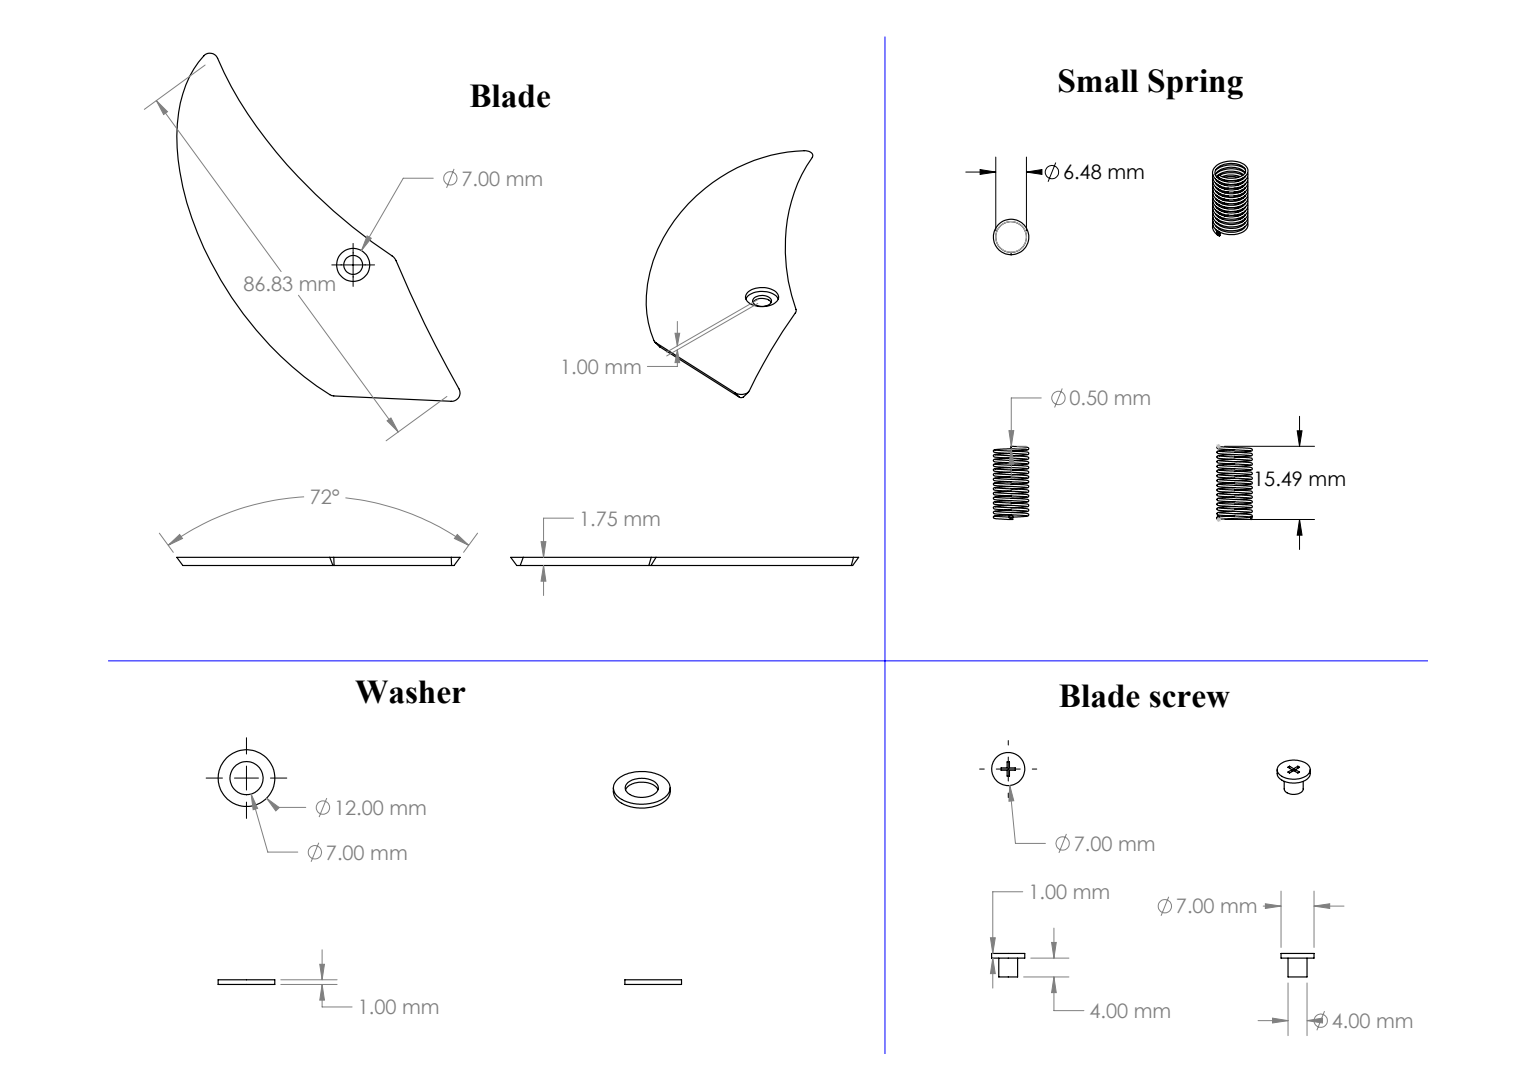
ISO-10303-21;
HEADER;
FILE_DESCRIPTION (('STEP AP203'),
    '1' );
FILE_NAME ('SmallSpring.step',
    '2026-10-08T11:28:20',
    ( '' ),
    ( '' ),
    'SwSTEP 2.0',
    'SolidWorks 2024',
    '' );
FILE_SCHEMA (( 'AUTOMOTIVE_DESIGN' ));
ENDSEC;

DATA;
#1=B_SPLINE_CURVE_WITH_KNOTS ( 'NONE', 3,
 ( #11082, #3985, #4982, #9929, #8605, #7599 ),
 .UNSPECIFIED., .F., .F.,
 ( 4, 2, 4 ),
 ( 0.000000000000000000, 0.0003771276215161150453, 0.0007542552430322300907 ),
 .UNSPECIFIED. ) ;
#3=CARTESIAN_POINT ( 'NONE',  ( 3.749999999999999112, 3.187500000000000444, -5.053300858899108405 ) ) ;
#9=CARTESIAN_POINT ( 'NONE',  ( 3.249999999999999556, 12.75000000000000178, -3.500000000000000000 ) ) ;
#19=CARTESIAN_POINT ( 'NONE',  ( -3.750000000000000000, 6.250000000000000000, -3.499999999999999112 ) ) ;
#20=CARTESIAN_POINT ( 'NONE',  ( 3.749999999999999556, 3.250000000000000000, -3.500000000000000444 ) ) ;
#24=CARTESIAN_POINT ( 'NONE',  ( -2.298097038856279362, 0.8750000000000000000, -5.798097038856278473 ) ) ;
#31=CARTESIAN_POINT ( 'NONE',  ( 0.000000000000000000, 3.000000000000000000, -0.2500000000000002220 ) ) ;
#37=CARTESIAN_POINT ( 'NONE',  ( -3.249999999999999556, 14.18750000000000000, -2.153805922287440833 ) ) ;
#42=CARTESIAN_POINT ( 'NONE',  ( 1.553300858899105963, 4.062500000000001776, -7.250000000000000888 ) ) ;
#43=CARTESIAN_POINT ( 'NONE',  ( -1.346194077712559167, 5.937500000000002665, -6.749999999999999112 ) ) ;
#47=CARTESIAN_POINT ( 'NONE',  ( 1.346194077712558057, 4.562500000000000888, -6.750000000000000000 ) ) ;
#59=CARTESIAN_POINT ( 'NONE',  ( 2.651650429449553314, 14.37500000000000000, -0.8483495705504476847 ) ) ;
#63=CARTESIAN_POINT ( 'NONE',  ( -3.249999999999999556, 3.750000000000000444, -3.500000000000000000 ) ) ;
#70=CARTESIAN_POINT ( 'NONE',  ( -3.249999999999999556, 1.250000000000000000, -3.499999999999999556 ) ) ;
#73=CARTESIAN_POINT ( 'NONE',  ( 2.298097038856278029, 7.125000000000000888, -5.798097038856279362 ) ) ;
#79=CARTESIAN_POINT ( 'NONE',  ( 2.298097038856279362, 1.875000000000000000, -1.201902961143720860 ) ) ;
#80=CARTESIAN_POINT ( 'NONE',  ( -1.553300858899107073, 1.937500000000000222, -7.249999999999999112 ) ) ;
#82=CARTESIAN_POINT ( 'NONE',  ( -3.750000000000000000, 7.312500000000000000, -5.053300858899105741 ) ) ;
#84=CARTESIAN_POINT ( 'NONE',  ( 3.749999999999999556, 4.250000000000000000, -3.500000000000000444 ) ) ;
#87=DIRECTION ( 'NONE',  ( 0.000000000000000000, 0.000000000000000000, -1.000000000000000000 ) ) ;
#90=CARTESIAN_POINT ( 'NONE',  ( 1.346194077712560944, 10.93750000000000000, -0.2500000000000010547 ) ) ;
#97=CARTESIAN_POINT ( 'NONE',  ( 3.749999999999998668, 4.687500000000000888, -5.053300858899107517 ) ) ;
#99=CARTESIAN_POINT ( 'NONE',  ( -3.750000000000000000, 5.812500000000000888, -5.053300858899105741 ) ) ;
#103=CARTESIAN_POINT ( 'NONE',  ( 3.249999999999998224, 3.187500000000000444, -4.846194077712561388 ) ) ;
#106=CARTESIAN_POINT ( 'NONE',  ( -2.298097038856278918, 2.375000000000000000, -5.798097038856277585 ) ) ;
#113=CARTESIAN_POINT ( 'NONE',  ( 1.346194077712560944, 14.93750000000000178, -0.2500000000000011102 ) ) ;
#115=EDGE_LOOP ( 'NONE', ( #2577, #6448, #3644, #14462 ) ) ;
#117=CARTESIAN_POINT ( 'NONE',  ( -4.592425496802573972E-16, 5.000000000000000000, -7.250000000000000000 ) ) ;
#118=CARTESIAN_POINT ( 'NONE',  ( -1.346194077712558945, 10.56249999999999822, -0.2500000000000002220 ) ) ;
#122=CARTESIAN_POINT ( 'NONE',  ( 1.346194077712558057, 3.562500000000000444, -6.750000000000000000 ) ) ;
#129=CARTESIAN_POINT ( 'NONE',  ( -3.249999999999999556, 9.187500000000000000, -2.153805922287440833 ) ) ;
#131=CARTESIAN_POINT ( 'NONE',  ( -4.592425496802573972E-16, 14.00000000000000000, -7.250000000000000000 ) ) ;
#136=CARTESIAN_POINT ( 'NONE',  ( 1.346194077712561166, 4.437500000000001776, -0.2500000000000011102 ) ) ;
#143=EDGE_LOOP ( 'NONE', ( #10004, #6723, #11790, #8217 ) ) ;
#145=CARTESIAN_POINT ( 'NONE',  ( 2.298097038856279362, 1.875000000000000000, -1.201902961143720860 ) ) ;
#147=CARTESIAN_POINT ( 'NONE',  ( 3.249999999999999556, 14.75000000000000178, -3.500000000000000000 ) ) ;
#148=CARTESIAN_POINT ( 'NONE',  ( -1.346194077712559167, 5.937500000000002665, -6.749999999999999112 ) ) ;
#154=CARTESIAN_POINT ( 'NONE',  ( -2.298097038856278918, 0.3750000000000000000, -5.798097038856277585 ) ) ;
#155=CARTESIAN_POINT ( 'NONE',  ( 2.651650429449552870, 1.124999999999999778, -6.151650429449553314 ) ) ;
#156=CARTESIAN_POINT ( 'NONE',  ( -2.651650429449552870, 4.125000000000000000, -0.8483495705504462414 ) ) ;
#158=CARTESIAN_POINT ( 'NONE',  ( 2.651650429449552870, 8.125000000000000000, -6.151650429449555091 ) ) ;
#161=EDGE_CURVE ( 'NONE', #6131, #12717, #6840, .T. ) ;
#166=CARTESIAN_POINT ( 'NONE',  ( 0.000000000000000000, 14.00000000000000000, -0.2500000000000002220 ) ) ;
#170=CARTESIAN_POINT ( 'NONE',  ( -3.749999999999999556, 8.750000000000000000, -3.499999999999999112 ) ) ;
#174=CARTESIAN_POINT ( 'NONE',  ( 1.553300858899108849, 9.937499999999998224, 0.2499999999999993616 ) ) ;
#175=CARTESIAN_POINT ( 'NONE',  ( -3.749999999999999556, 5.750000000000000000, -3.499999999999999112 ) ) ;
#178=CARTESIAN_POINT ( 'NONE',  ( -2.298097038856278029, 2.625000000000000000, -1.201902961143720638 ) ) ;
#181=CARTESIAN_POINT ( 'NONE',  ( 2.298097038856279362, 6.875000000000000000, -1.201902961143720860 ) ) ;
#189=CARTESIAN_POINT ( 'NONE',  ( -3.980102097228897245E-16, 14.50000000000000000, -6.749999999999999112 ) ) ;
#193=CARTESIAN_POINT ( 'NONE',  ( 2.651650429449552870, 7.125000000000000888, -6.151650429449555091 ) ) ;
#194=CARTESIAN_POINT ( 'NONE',  ( -2.298097038856279362, 8.874999999999996447, -5.798097038856278473 ) ) ;
#197=CARTESIAN_POINT ( 'NONE',  ( -3.249999999999999556, 5.187500000000001776, -2.153805922287440833 ) ) ;
#204=CARTESIAN_POINT ( 'NONE',  ( -3.249999999999999556, 0.3125000000000000555, -4.846194077712557835 ) ) ;
#206=CARTESIAN_POINT ( 'NONE',  ( -3.750000000000000000, 12.81250000000000178, -5.053300858899105741 ) ) ;
#209=CARTESIAN_POINT ( 'NONE',  ( 1.346194077712561166, 3.437500000000000444, -0.2500000000000011102 ) ) ;
#216=CARTESIAN_POINT ( 'NONE',  ( -2.298097038856278918, 8.375000000000000000, -5.798097038856277585 ) ) ;
#218=CARTESIAN_POINT ( 'NONE',  ( 2.298097038856278473, 14.62500000000000000, -5.798097038856279362 ) ) ;
#220=CARTESIAN_POINT ( 'NONE',  ( 0.000000000000000000, 7.500000000000000888, -0.2500000000000002220 ) ) ;
#225=CARTESIAN_POINT ( 'NONE',  ( 2.298097038856278473, 1.625000000000000222, -5.798097038856279362 ) ) ;
#226=CARTESIAN_POINT ( 'NONE',  ( -2.651650429449552870, 2.625000000000000000, -0.8483495705504467965 ) ) ;
#227=CARTESIAN_POINT ( 'NONE',  ( 1.553300858899108849, 4.937500000000000888, 0.2499999999999993616 ) ) ;
#229=CARTESIAN_POINT ( 'NONE',  ( 1.553300858899105963, 6.062500000000000888, -7.250000000000000888 ) ) ;
#239=CARTESIAN_POINT ( 'NONE',  ( 1.346194077712560944, 8.937500000000001776, -0.2500000000000010547 ) ) ;
#242=CARTESIAN_POINT ( 'NONE',  ( -3.750000000000000000, 10.81250000000000000, -5.053300858899105741 ) ) ;
#246=CARTESIAN_POINT ( 'NONE',  ( 2.651650429449553759, 9.875000000000000000, -0.8483495705504471296 ) ) ;
#247=CARTESIAN_POINT ( 'NONE',  ( 3.749999999999998668, 4.187500000000000888, -5.053300858899108405 ) ) ;
#251=CARTESIAN_POINT ( 'NONE',  ( 2.298097038856278029, 5.125000000000000000, -5.798097038856279362 ) ) ;
#253=CARTESIAN_POINT ( 'NONE',  ( 2.651650429449553759, 10.87500000000000178, -0.8483495705504471296 ) ) ;
#258=CARTESIAN_POINT ( 'NONE',  ( 3.249999999999998668, 8.687500000000000000, -4.846194077712560500 ) ) ;
#260=CARTESIAN_POINT ( 'NONE',  ( -0.3766621274091715987, 0.2398196381212478467, -0.1347136637304948426 ) ) ;
#270=CARTESIAN_POINT ( 'NONE',  ( -3.750000000000000000, 10.68750000000000178, -1.946699141100893149 ) ) ;
#271=CARTESIAN_POINT ( 'NONE',  ( 1.346194077712558279, 6.062500000000000000, -6.750000000000000888 ) ) ;
#272=CARTESIAN_POINT ( 'NONE',  ( -3.249999999999999556, 10.75000000000000000, -3.500000000000000000 ) ) ;
#274=VECTOR ( 'NONE', #10771, 1000.000000000000000 ) ;
#277=CARTESIAN_POINT ( 'NONE',  ( -2.298097038856278473, 5.125000000000000000, -1.201902961143720416 ) ) ;
#287=CARTESIAN_POINT ( 'NONE',  ( 2.298097038856279362, 0.8750000000000000000, -1.201902961143720860 ) ) ;
#288=CARTESIAN_POINT ( 'NONE',  ( -1.553300858899107295, 11.43750000000000000, -7.250000000000000000 ) ) ;
#291=CARTESIAN_POINT ( 'NONE',  ( -2.651650429449552870, 11.62500000000000000, -0.8483495705504467965 ) ) ;
#294=CARTESIAN_POINT ( 'NONE',  ( -2.298097038856279362, 1.874999999999999778, -5.798097038856278473 ) ) ;
#303=CARTESIAN_POINT ( 'NONE',  ( 3.249999999999998668, 6.687500000000000888, -4.846194077712560500 ) ) ;
#305=CARTESIAN_POINT ( 'NONE',  ( 3.249999999999999556, 1.249999999999999778, -3.500000000000000000 ) ) ;
#306=CARTESIAN_POINT ( 'NONE',  ( 0.000000000000000000, 9.500000000000000000, -0.2500000000000002220 ) ) ;
#310=CARTESIAN_POINT ( 'NONE',  ( -1.346194077712559389, 4.062500000000000000, -0.2500000000000002220 ) ) ;
#311=CARTESIAN_POINT ( 'NONE',  ( 0.000000000000000000, 15.50000000000000178, -0.2500000000000002220 ) ) ;
#312=CARTESIAN_POINT ( 'NONE',  ( -1.553300858899106407, 7.062500000000000000, 0.2500000000000002220 ) ) ;
#314=CARTESIAN_POINT ( 'NONE',  ( -3.750000000000000000, 6.812500000000001776, -5.053300858899105741 ) ) ;
#318=VECTOR ( 'NONE', #638, 1000.000000000000000 ) ;
#326=CARTESIAN_POINT ( 'NONE',  ( 2.651650429449552870, 9.125000000000000000, -6.151650429449555091 ) ) ;
#330=CARTESIAN_POINT ( 'NONE',  ( 3.750000000000000000, 9.750000000000000000, -3.500000000000000444 ) ) ;
#331=CARTESIAN_POINT ( 'NONE',  ( -1.553300858899106629, 7.562500000000000888, 0.2499999999999998335 ) ) ;
#335=CARTESIAN_POINT ( 'NONE',  ( 1.346194077712561166, 4.437499999999999112, -0.2500000000000011102 ) ) ;
#336=CARTESIAN_POINT ( 'NONE',  ( 2.651650429449553759, 8.875000000000001776, -0.8483495705504471296 ) ) ;
#340=CARTESIAN_POINT ( 'NONE',  ( -1.346194077712559389, 7.437500000000000888, -6.749999999999999112 ) ) ;
#353=CARTESIAN_POINT ( 'NONE',  ( -2.651650429449552870, 12.62500000000000000, -0.8483495705504467965 ) ) ;
#354=CARTESIAN_POINT ( 'NONE',  ( 1.346194077712561166, 12.43750000000000000, -0.2500000000000011102 ) ) ;
#355=CARTESIAN_POINT ( 'NONE',  ( -3.249999999999999112, 11.81250000000000178, -4.846194077712558723 ) ) ;
#358=CARTESIAN_POINT ( 'NONE',  ( -1.346194077712559389, 7.062500000000000000, -0.2500000000000002220 ) ) ;
#367=EDGE_CURVE ( 'NONE', #14660, #7693, #12911, .T. ) ;
#370=CARTESIAN_POINT ( 'NONE',  ( -3.249999999999999556, 9.250000000000000000, -3.499999999999999556 ) ) ;
#371=CARTESIAN_POINT ( 'NONE',  ( -3.249999999999999556, 0.1875000000000000278, -2.153805922287440833 ) ) ;
#373=CARTESIAN_POINT ( 'NONE',  ( 3.749999999999999112, 14.81250000000000000, -1.946699141100892039 ) ) ;
#376=CARTESIAN_POINT ( 'NONE',  ( 0.000000000000000000, 1.000000000000000000, 0.2500000000000002220 ) ) ;
#385=CARTESIAN_POINT ( 'NONE',  ( 1.346194077712558279, 5.562500000000000000, -6.750000000000000000 ) ) ;
#387=CARTESIAN_POINT ( 'NONE',  ( -2.298097038856278473, 13.12500000000000000, -1.201902961143720416 ) ) ;
#388=CARTESIAN_POINT ( 'NONE',  ( 3.249999999999998224, 12.18750000000000178, -4.846194077712561388 ) ) ;
#392=CARTESIAN_POINT ( 'NONE',  ( 0.000000000000000000, 6.000000000000000000, -0.2500000000000002220 ) ) ;
#393=CARTESIAN_POINT ( 'NONE',  ( -3.749999999999999556, 0.7499999999999998890, -3.499999999999999112 ) ) ;
#394=CARTESIAN_POINT ( 'NONE',  ( 1.553300858899105963, 5.562500000000000000, -7.250000000000000000 ) ) ;
#396=CARTESIAN_POINT ( 'NONE',  ( 3.749999999999999556, 8.250000000000000000, -3.500000000000000444 ) ) ;
#401=CARTESIAN_POINT ( 'NONE',  ( 2.298097038856279362, 14.87500000000000178, -1.201902961143720860 ) ) ;
#404=CARTESIAN_POINT ( 'NONE',  ( 3.249999999999998224, 0.1875000000000000833, -4.846194077712561388 ) ) ;
#408=CARTESIAN_POINT ( 'NONE',  ( 2.651650429449553759, 7.875000000000000000, -0.8483495705504471296 ) ) ;
#409=CARTESIAN_POINT ( 'NONE',  ( -4.592425496802573972E-16, 8.000000000000000000, -7.250000000000000000 ) ) ;
#413=CARTESIAN_POINT ( 'NONE',  ( 2.298097038856278029, 6.125000000000000000, -5.798097038856279362 ) ) ;
#414=CARTESIAN_POINT ( 'NONE',  ( 2.651650429449552870, 11.62500000000000000, -6.151650429449554203 ) ) ;
#416=LINE ( 'NONE', #571, #1497 ) ;
#418=CARTESIAN_POINT ( 'NONE',  ( -3.249999999999999556, 7.250000000000000000, -3.499999999999999556 ) ) ;
#430=CARTESIAN_POINT ( 'NONE',  ( 1.553300858899105963, 11.06250000000000178, -7.249999999999999112 ) ) ;
#431=CARTESIAN_POINT ( 'NONE',  ( -3.249999999999999112, 11.68749999999999822, -2.153805922287440833 ) ) ;
#432=CARTESIAN_POINT ( 'NONE',  ( 2.298097038856279362, 12.37500000000000178, -1.201902961143720860 ) ) ;
#437=CARTESIAN_POINT ( 'NONE',  ( 1.346194077712560944, 6.937500000000000000, -0.2500000000000010547 ) ) ;
#438=EDGE_CURVE ( 'NONE', #15209, #13242, #13713, .T. ) ;
#443=CARTESIAN_POINT ( 'NONE',  ( -0.3766621274091715432, -0.2054769798019681903, -0.1347136637304948981 ) ) ;
#445=CARTESIAN_POINT ( 'NONE',  ( -3.249999999999999556, 1.187500000000000444, -2.153805922287440833 ) ) ;
#446=CARTESIAN_POINT ( 'NONE',  ( 3.749999999999999112, 12.81250000000000000, -1.946699141100892039 ) ) ;
#450=CARTESIAN_POINT ( 'NONE',  ( -3.749999999999999556, 0.1875000000000001110, -1.946699141100892927 ) ) ;
#459=CARTESIAN_POINT ( 'NONE',  ( -3.249999999999999556, 8.312500000000000000, -4.846194077712557835 ) ) ;
#461=CARTESIAN_POINT ( 'NONE',  ( 3.249999999999998668, 12.68750000000000178, -4.846194077712560500 ) ) ;
#462=CARTESIAN_POINT ( 'NONE',  ( 3.249999999999998224, 9.187500000000001776, -4.846194077712561388 ) ) ;
#466=CARTESIAN_POINT ( 'NONE',  ( -2.298097038856278918, 5.375000000000000000, -5.798097038856277585 ) ) ;
#467=CARTESIAN_POINT ( 'NONE',  ( 3.749999999999999556, 7.250000000000000000, -3.500000000000000444 ) ) ;
#469=CARTESIAN_POINT ( 'NONE',  ( 2.651650429449552870, 7.625000000000000000, -6.151650429449554203 ) ) ;
#471=CARTESIAN_POINT ( 'NONE',  ( 2.651650429449554203, 9.374999999999998224, -0.8483495705504471296 ) ) ;
#479=CARTESIAN_POINT ( 'NONE',  ( -3.249999999999999112, -0.3124999999999999445, -2.153805922287440833 ) ) ;
#483=CARTESIAN_POINT ( 'NONE',  ( -1.553300858899106629, 7.062500000000000000, 0.2500000000000002220 ) ) ;
#484=CARTESIAN_POINT ( 'NONE',  ( -1.553300858899106629, 9.562500000000000000, 0.2499999999999998335 ) ) ;
#487=CARTESIAN_POINT ( 'NONE',  ( 2.298097038856279362, 10.37500000000000000, -1.201902961143720860 ) ) ;
#488=CARTESIAN_POINT ( 'NONE',  ( -1.553300858899107295, 8.437500000000000000, -7.250000000000000000 ) ) ;
#491=CARTESIAN_POINT ( 'NONE',  ( 1.346194077712560944, 8.937500000000001776, -0.2500000000000010547 ) ) ;
#497=FACE_OUTER_BOUND ( 'NONE', #2057, .T. ) ;
#502=CARTESIAN_POINT ( 'NONE',  ( -2.651650429449552870, 10.62500000000000178, -0.8483495705504467965 ) ) ;
#503=CARTESIAN_POINT ( 'NONE',  ( 0.000000000000000000, 9.500000000000001776, -0.2500000000000002220 ) ) ;
#504=CARTESIAN_POINT ( 'NONE',  ( 1.346194077712558057, 1.562500000000000000, -6.750000000000000000 ) ) ;
#506=CARTESIAN_POINT ( 'NONE',  ( -3.249999999999999556, 7.250000000000000000, -3.499999999999999556 ) ) ;
#518=CARTESIAN_POINT ( 'NONE',  ( -3.980102097228897245E-16, 0.5000000000000000000, -6.749999999999999112 ) ) ;
#519=CARTESIAN_POINT ( 'NONE',  ( -1.553300858899107295, 12.43750000000000000, -7.250000000000000000 ) ) ;
#523=CARTESIAN_POINT ( 'NONE',  ( 3.749999999999998668, 1.687500000000000000, -5.053300858899107517 ) ) ;
#533=CARTESIAN_POINT ( 'NONE',  ( -3.249999999999999556, 7.250000000000000000, -3.499999999999999556 ) ) ;
#536=CARTESIAN_POINT ( 'NONE',  ( 3.249999999999998224, 1.312500000000000000, -2.153805922287439945 ) ) ;
#538=CARTESIAN_POINT ( 'NONE',  ( 2.298097038856279362, 11.37500000000000000, -1.201902961143720860 ) ) ;
#541=CARTESIAN_POINT ( 'NONE',  ( 3.249999999999999556, 4.750000000000000000, -3.500000000000000000 ) ) ;
#542=CARTESIAN_POINT ( 'NONE',  ( -2.651650429449552870, 5.875000000000000888, -6.151650429449552426 ) ) ;
#543=CARTESIAN_POINT ( 'NONE',  ( -1.553300858899106407, 11.06250000000000000, 0.2500000000000002220 ) ) ;
#546=CARTESIAN_POINT ( 'NONE',  ( 0.000000000000000000, 8.500000000000000000, 0.2500000000000002220 ) ) ;
#558=CARTESIAN_POINT ( 'NONE',  ( 1.553300858899109516, 12.43750000000000000, 0.2499999999999993616 ) ) ;
#559=VERTEX_POINT ( 'NONE', #11746 ) ;
#562=CARTESIAN_POINT ( 'NONE',  ( -2.651650429449552870, 11.12500000000000000, -0.8483495705504462414 ) ) ;
#563=CARTESIAN_POINT ( 'NONE',  ( 1.553300858899105963, 9.062500000000003553, -7.249999999999999112 ) ) ;
#567=CARTESIAN_POINT ( 'NONE',  ( -1.346194077712559167, 7.937500000000001776, -6.749999999999999112 ) ) ;
#568=CARTESIAN_POINT ( 'NONE',  ( 1.553300858899105963, 0.06250000000000016653, -7.250000000000000888 ) ) ;
#571=CARTESIAN_POINT ( 'NONE',  ( -0.3766621274091715987, -0.2500000000000000000, 0.1491815183709511716 ) ) ;
#573=CARTESIAN_POINT ( 'NONE',  ( -3.980102097228897245E-16, 13.50000000000000000, -6.749999999999999112 ) ) ;
#578=CARTESIAN_POINT ( 'NONE',  ( 0.000000000000000000, 1.530808498934191509E-17, 0.000000000000000000 ) ) ;
#582=CARTESIAN_POINT ( 'NONE',  ( 3.749999999999998668, 14.18750000000000178, -5.053300858899108405 ) ) ;
#584=CARTESIAN_POINT ( 'NONE',  ( -3.249999999999999556, 10.75000000000000178, -3.500000000000000000 ) ) ;
#586=CARTESIAN_POINT ( 'NONE',  ( 0.000000000000000000, 0.000000000000000000, -0.2500000000000002220 ) ) ;
#588=CARTESIAN_POINT ( 'NONE',  ( -1.346194077712559389, 9.437500000000000000, -6.749999999999999112 ) ) ;
#600=CARTESIAN_POINT ( 'NONE',  ( -3.249999999999999556, 5.187500000000001776, -2.153805922287440833 ) ) ;
#601=CARTESIAN_POINT ( 'NONE',  ( 2.651650429449552870, 12.62500000000000000, -6.151650429449554203 ) ) ;
#607=CARTESIAN_POINT ( 'NONE',  ( -2.651650429449552870, 0.1250000000000000278, -0.8483495705504462414 ) ) ;
#612=DIRECTION ( 'NONE',  ( -1.000000000000000000, 0.000000000000000000, 0.000000000000000000 ) ) ;
#614=LINE ( 'NONE', #5091, #1247 ) ;
#616=CARTESIAN_POINT ( 'NONE',  ( -2.298097038856278918, 9.375000000000000000, -5.798097038856277585 ) ) ;
#617=DIRECTION ( 'NONE',  ( 0.000000000000000000, 0.000000000000000000, -1.000000000000000000 ) ) ;
#618=CARTESIAN_POINT ( 'NONE',  ( -3.980102097228897738E-16, 5.000000000000000000, -6.749999999999999112 ) ) ;
#619=CARTESIAN_POINT ( 'NONE',  ( 3.249999999999998224, 10.31250000000000000, -2.153805922287439945 ) ) ;
#622=CARTESIAN_POINT ( 'NONE',  ( 1.346194077712560944, 4.937500000000001776, -0.2500000000000010547 ) ) ;
#623=CARTESIAN_POINT ( 'NONE',  ( -1.553300858899106629, 4.562500000000000000, 0.2499999999999998335 ) ) ;
#624=CARTESIAN_POINT ( 'NONE',  ( 2.651650429449552870, 10.62500000000000000, -6.151650429449554203 ) ) ;
#628=CARTESIAN_POINT ( 'NONE',  ( -1.553300858899106629, 10.56249999999999822, 0.2500000000000002220 ) ) ;
#636=CARTESIAN_POINT ( 'NONE',  ( 1.553300858899105963, 12.06250000000000000, -7.250000000000000888 ) ) ;
#638=DIRECTION ( 'NONE',  ( -0.000000000000000000, -1.000000000000000000, -0.000000000000000000 ) ) ;
#640=CARTESIAN_POINT ( 'NONE',  ( 3.749999999999999556, 10.25000000000000178, -3.500000000000000444 ) ) ;
#642=CARTESIAN_POINT ( 'NONE',  ( 0.000000000000000000, 8.500000000000000000, -0.2500000000000002220 ) ) ;
#645=CARTESIAN_POINT ( 'NONE',  ( -3.749999999999999556, 13.31250000000000000, -5.053300858899104853 ) ) ;
#650=CARTESIAN_POINT ( 'NONE',  ( -3.249999999999999556, 10.31250000000000000, -4.846194077712557835 ) ) ;
#652=CARTESIAN_POINT ( 'NONE',  ( -1.346194077712559389, 11.06250000000000000, -0.2500000000000002220 ) ) ;
#653=DIRECTION ( 'NONE',  ( 1.000000000000000000, 0.000000000000000000, -0.000000000000000000 ) ) ;
#659=CARTESIAN_POINT ( 'NONE',  ( 2.651650429449552870, 2.625000000000000000, -6.151650429449554203 ) ) ;
#660=CARTESIAN_POINT ( 'NONE',  ( -1.346194077712558945, 12.56250000000000355, -0.2500000000000002220 ) ) ;
#661=CARTESIAN_POINT ( 'NONE',  ( 3.249999999999999112, 0.8125000000000001110, -2.153805922287439945 ) ) ;
#663=CARTESIAN_POINT ( 'NONE',  ( 0.000000000000000000, 11.00000000000000000, -0.2500000000000002220 ) ) ;
#674=CARTESIAN_POINT ( 'NONE',  ( -3.249999999999999556, 6.312500000000000888, -4.846194077712557835 ) ) ;
#676=CARTESIAN_POINT ( 'NONE',  ( -4.592425496802573972E-16, 2.000000000000000000, -7.250000000000000000 ) ) ;
#680=CARTESIAN_POINT ( 'NONE',  ( -3.749999999999999556, 3.312500000000000000, -5.053300858899104853 ) ) ;
#684=CARTESIAN_POINT ( 'NONE',  ( 2.651650429449553759, 1.875000000000000000, -0.8483495705504471296 ) ) ;
#690=CARTESIAN_POINT ( 'NONE',  ( -2.298097038856279362, 3.875000000000000444, -5.798097038856278473 ) ) ;
#691=CARTESIAN_POINT ( 'NONE',  ( -1.346194077712559167, 12.93750000000000178, -6.749999999999999112 ) ) ;
#694=CARTESIAN_POINT ( 'NONE',  ( 3.249999999999999112, 6.812500000000000000, -2.153805922287439945 ) ) ;
#695=CARTESIAN_POINT ( 'NONE',  ( -3.750000000000000000, 3.687500000000000444, -1.946699141100893149 ) ) ;
#696=CARTESIAN_POINT ( 'NONE',  ( -3.750000000000000000, 10.25000000000000000, -3.499999999999999112 ) ) ;
#697=LINE ( 'NONE', #14933, #4951 ) ;
#700=CARTESIAN_POINT ( 'NONE',  ( -4.592425496802573972E-16, 10.00000000000000000, -7.250000000000000000 ) ) ;
#709=CARTESIAN_POINT ( 'NONE',  ( 2.651650429449552870, 14.12500000000000000, -6.151650429449555091 ) ) ;
#715=CARTESIAN_POINT ( 'NONE',  ( -1.346194077712559167, 8.937500000000000000, -6.749999999999999112 ) ) ;
#717=CARTESIAN_POINT ( 'NONE',  ( -1.553300858899106629, -0.4374999999999998890, 0.2500000000000002220 ) ) ;
#721=CARTESIAN_POINT ( 'NONE',  ( 1.346194077712558057, 11.56249999999999822, -6.750000000000000000 ) ) ;
#724=CARTESIAN_POINT ( 'NONE',  ( -1.346194077712559389, 8.437500000000000000, -6.749999999999999112 ) ) ;
#731=CARTESIAN_POINT ( 'NONE',  ( -2.651650429449553314, 1.375000000000000000, -6.151650429449552426 ) ) ;
#732=CARTESIAN_POINT ( 'NONE',  ( 2.651650429449553314, 1.375000000000000000, -0.8483495705504476847 ) ) ;
#734=CARTESIAN_POINT ( 'NONE',  ( -3.980102097228897738E-16, 14.00000000000000000, -6.749999999999999112 ) ) ;
#736=CARTESIAN_POINT ( 'NONE',  ( -2.298097038856278473, 9.125000000000000000, -1.201902961143720416 ) ) ;
#746=CARTESIAN_POINT ( 'NONE',  ( 3.249999999999999112, 5.812500000000000000, -2.153805922287439945 ) ) ;
#748=CARTESIAN_POINT ( 'NONE',  ( -1.553300858899107073, 0.9375000000000002220, -7.249999999999999112 ) ) ;
#753=CARTESIAN_POINT ( 'NONE',  ( 0.000000000000000000, 0.000000000000000000, -0.2500000000000002220 ) ) ;
#755=CARTESIAN_POINT ( 'NONE',  ( 2.651650429449553759, 6.875000000000000000, -0.8483495705504471296 ) ) ;
#758=CARTESIAN_POINT ( 'NONE',  ( 1.553300858899105963, 0.5625000000000002220, -7.250000000000000000 ) ) ;
#760=CARTESIAN_POINT ( 'NONE',  ( 2.298097038856278029, 13.12500000000000178, -5.798097038856279362 ) ) ;
#767=CARTESIAN_POINT ( 'NONE',  ( 1.346194077712558279, 4.062500000000001776, -6.750000000000000888 ) ) ;
#772=CARTESIAN_POINT ( 'NONE',  ( 3.749999999999999556, 5.249999999999999112, -3.500000000000000444 ) ) ;
#774=CARTESIAN_POINT ( 'NONE',  ( 3.749999999999999556, 8.812500000000000000, -1.946699141100892261 ) ) ;
#777=CARTESIAN_POINT ( 'NONE',  ( -2.298097038856278918, 8.375000000000000000, -5.798097038856277585 ) ) ;
#778=CARTESIAN_POINT ( 'NONE',  ( -3.749999999999999556, 10.75000000000000000, -3.499999999999999112 ) ) ;
#787=CARTESIAN_POINT ( 'NONE',  ( 2.298097038856278029, 4.125000000000000000, -5.798097038856279362 ) ) ;
#794=CARTESIAN_POINT ( 'NONE',  ( 1.346194077712561166, 8.437500000000000000, -0.2500000000000011102 ) ) ;
#798=CARTESIAN_POINT ( 'NONE',  ( -2.651650429449552870, 14.12500000000000000, -0.8483495705504462414 ) ) ;
#802=CARTESIAN_POINT ( 'NONE',  ( 0.000000000000000000, 12.00000000000000000, -0.2500000000000002220 ) ) ;
#805=CARTESIAN_POINT ( 'NONE',  ( 1.346194077712560944, 9.937499999999998224, -0.2500000000000010547 ) ) ;
#811=CARTESIAN_POINT ( 'NONE',  ( 1.553300858899105963, 15.06250000000000178, -7.249999999999999112 ) ) ;
#812=CARTESIAN_POINT ( 'NONE',  ( 3.749999999999999112, 1.312500000000000000, -1.946699141100893149 ) ) ;
#813=CARTESIAN_POINT ( 'NONE',  ( 3.249999999999999112, 1.812500000000000222, -2.153805922287439945 ) ) ;
#815=CARTESIAN_POINT ( 'NONE',  ( 2.298097038856278473, 12.62500000000000000, -5.798097038856279362 ) ) ;
#816=DIRECTION ( 'NONE',  ( 0.000000000000000000, 0.000000000000000000, -1.000000000000000000 ) ) ;
#825=CARTESIAN_POINT ( 'NONE',  ( 1.346194077712558057, 3.562500000000000444, -6.750000000000000000 ) ) ;
#827=CARTESIAN_POINT ( 'NONE',  ( 3.749999999999999556, 0.2500000000000001110, -3.500000000000000444 ) ) ;
#831=CARTESIAN_POINT ( 'NONE',  ( 3.749999999999998668, 4.687500000000000888, -5.053300858899107517 ) ) ;
#836=CARTESIAN_POINT ( 'NONE',  ( 3.749999999999999556, 2.812500000000000000, -1.946699141100892261 ) ) ;
#845=CARTESIAN_POINT ( 'NONE',  ( -3.249999999999999112, 1.687499999999999778, -2.153805922287440833 ) ) ;
#847=CARTESIAN_POINT ( 'NONE',  ( -3.749999999999999556, 10.75000000000000178, -3.499999999999999112 ) ) ;
#848=CARTESIAN_POINT ( 'NONE',  ( -4.592425496802573972E-16, 14.50000000000000000, -7.249999999999999112 ) ) ;
#851=CARTESIAN_POINT ( 'NONE',  ( 3.249999999999998668, 7.687500000000000000, -4.846194077712560500 ) ) ;
#852=CARTESIAN_POINT ( 'NONE',  ( 0.000000000000000000, 14.50000000000000000, 0.2500000000000002220 ) ) ;
#862=CARTESIAN_POINT ( 'NONE',  ( 1.346194077712561166, 4.437500000000001776, -0.2500000000000011102 ) ) ;
#863=EDGE_LOOP ( 'NONE', ( #950, #5112, #7904, #11736 ) ) ;
#869=CARTESIAN_POINT ( 'NONE',  ( -1.346194077712558945, 11.56250000000000178, -0.2500000000000002220 ) ) ;
#871=CARTESIAN_POINT ( 'NONE',  ( 1.553300858899105963, 14.56250000000000000, -7.250000000000000888 ) ) ;
#874=PLANE ( 'NONE',  #5289 ) ;
#877=CARTESIAN_POINT ( 'NONE',  ( -2.298097038856278918, 7.375000000000000888, -5.798097038856277585 ) ) ;
#884=CARTESIAN_POINT ( 'NONE',  ( 3.749999999999999112, 2.812500000000000000, -1.946699141100892039 ) ) ;
#885=CARTESIAN_POINT ( 'NONE',  ( 3.249999999999999556, 15.25000000000000355, -3.500000000000000000 ) ) ;
#888=CARTESIAN_POINT ( 'NONE',  ( -3.249999999999999556, 7.250000000000000000, -3.499999999999999556 ) ) ;
#889=CARTESIAN_POINT ( 'NONE',  ( 1.346194077712560944, 10.93750000000000000, -0.2500000000000010547 ) ) ;
#892=( LENGTH_UNIT ( ) NAMED_UNIT ( * ) SI_UNIT ( .MILLI., .METRE. ) );
#899=CARTESIAN_POINT ( 'NONE',  ( 3.249999999999998668, 11.68750000000000000, -4.846194077712560500 ) ) ;
#900=ORIENTED_EDGE ( 'NONE', *, *, #13823, .F. ) ;
#902=CARTESIAN_POINT ( 'NONE',  ( 2.298097038856278473, 5.625000000000000000, -5.798097038856279362 ) ) ;
#904=CARTESIAN_POINT ( 'NONE',  ( 3.749999999999999556, 1.250000000000000222, -3.500000000000000444 ) ) ;
#908=CARTESIAN_POINT ( 'NONE',  ( 1.346194077712560944, 0.9374999999999998890, -0.2500000000000010547 ) ) ;
#909=CARTESIAN_POINT ( 'NONE',  ( 1.553300858899108849, 3.937500000000000000, 0.2499999999999993616 ) ) ;
#910=CARTESIAN_POINT ( 'NONE',  ( 0.000000000000000000, 3.061616997868383018E-17, 0.2500000000000002220 ) ) ;
#915=CARTESIAN_POINT ( 'NONE',  ( 3.249999999999999556, 6.250000000000000000, -3.500000000000000000 ) ) ;
#919=CARTESIAN_POINT ( 'NONE',  ( -3.750000000000000000, 10.68750000000000178, -1.946699141100893149 ) ) ;
#920=CARTESIAN_POINT ( 'NONE',  ( 2.651650429449553759, 11.87500000000000000, -0.8483495705504471296 ) ) ;
#924=CARTESIAN_POINT ( 'NONE',  ( 3.249999999999999556, 7.750000000000000000, -3.500000000000000000 ) ) ;
#925=CARTESIAN_POINT ( 'NONE',  ( 1.346194077712558279, 1.062500000000000444, -6.750000000000000888 ) ) ;
#930=CARTESIAN_POINT ( 'NONE',  ( -2.298097038856278918, 0.3750000000000000000, -5.798097038856277585 ) ) ;
#932=CARTESIAN_POINT ( 'NONE',  ( 1.346194077712558279, 3.062500000000000000, -6.750000000000000888 ) ) ;
#939=CARTESIAN_POINT ( 'NONE',  ( -2.298097038856278029, 10.62500000000000178, -1.201902961143720638 ) ) ;
#941=CARTESIAN_POINT ( 'NONE',  ( -3.750000000000000000, 1.812499999999999778, -5.053300858899105741 ) ) ;
#946=CARTESIAN_POINT ( 'NONE',  ( -3.249999999999999556, 10.25000000000000000, -3.499999999999999556 ) ) ;
#950=ORIENTED_EDGE ( 'NONE', *, *, #9967, .F. ) ;
#952=CARTESIAN_POINT ( 'NONE',  ( 3.749999999999999556, 15.25000000000000355, -3.500000000000000444 ) ) ;
#953=CARTESIAN_POINT ( 'NONE',  ( 3.249999999999998224, 13.31250000000000178, -2.153805922287439945 ) ) ;
#956=CARTESIAN_POINT ( 'NONE',  ( -1.346194077712559389, 14.43750000000000000, -6.749999999999999112 ) ) ;
#959=CARTESIAN_POINT ( 'NONE',  ( -1.346194077712559389, 5.437500000000002665, -6.749999999999999112 ) ) ;
#966=CARTESIAN_POINT ( 'NONE',  ( 2.298097038856279362, 11.87500000000000000, -1.201902961143720860 ) ) ;
#968=EDGE_LOOP ( 'NONE', ( #12812, #2857, #5859, #13093 ) ) ;
#969=CARTESIAN_POINT ( 'NONE',  ( 1.553300858899105963, 9.062500000000000000, -7.250000000000000888 ) ) ;
#971=CARTESIAN_POINT ( 'NONE',  ( -3.750000000000000000, 0.8125000000000001110, -5.053300858899105741 ) ) ;
#972=CARTESIAN_POINT ( 'NONE',  ( 1.346194077712561166, 5.437500000000000888, -0.2500000000000011102 ) ) ;
#975=CARTESIAN_POINT ( 'NONE',  ( -2.298097038856278918, 4.375000000000000000, -5.798097038856277585 ) ) ;
#976=CARTESIAN_POINT ( 'NONE',  ( -2.651650429449552870, 7.125000000000000000, -0.8483495705504462414 ) ) ;
#986=CARTESIAN_POINT ( 'NONE',  ( 1.346194077712561166, 6.437499999999999112, -0.2500000000000011102 ) ) ;
#988=CARTESIAN_POINT ( 'NONE',  ( -2.651650429449552870, 7.874999999999999112, -6.151650429449552426 ) ) ;
#989=CARTESIAN_POINT ( 'NONE',  ( 1.553300858899108849, 11.93750000000000000, 0.2499999999999993616 ) ) ;
#993=CARTESIAN_POINT ( 'NONE',  ( -3.750000000000000000, 13.68750000000000178, -1.946699141100893149 ) ) ;
#1001=CARTESIAN_POINT ( 'NONE',  ( -3.249999999999999556, 4.250000000000000000, -3.499999999999999556 ) ) ;
#1004=CARTESIAN_POINT ( 'NONE',  ( -2.298097038856279362, 3.875000000000000444, -5.798097038856278473 ) ) ;
#1006=DIRECTION ( 'NONE',  ( 0.000000000000000000, 0.000000000000000000, -1.000000000000000000 ) ) ;
#1012=CARTESIAN_POINT ( 'NONE',  ( -3.249999999999999556, 11.75000000000000178, -3.500000000000000000 ) ) ;
#1015=CARTESIAN_POINT ( 'NONE',  ( 2.651650429449554203, 0.3750000000000001110, -0.8483495705504471296 ) ) ;
#1024=CARTESIAN_POINT ( 'NONE',  ( 0.000000000000000000, 10.00000000000000000, -0.2500000000000002220 ) ) ;
#1026=CARTESIAN_POINT ( 'NONE',  ( 0.000000000000000000, 3.061616997868383018E-17, 0.1491815183709511716 ) ) ;
#1030=CARTESIAN_POINT ( 'NONE',  ( -2.651650429449553314, 5.375000000000000000, -6.151650429449552426 ) ) ;
#1031=CARTESIAN_POINT ( 'NONE',  ( -2.651650429449552870, 1.625000000000000000, -0.8483495705504467965 ) ) ;
#1035=CARTESIAN_POINT ( 'NONE',  ( -3.249999999999999556, 13.25000000000000000, -3.499999999999999556 ) ) ;
#1038=CARTESIAN_POINT ( 'NONE',  ( 3.249999999999999556, 2.750000000000000000, -3.500000000000000000 ) ) ;
#1045=CARTESIAN_POINT ( 'NONE',  ( 1.346194077712560944, 12.93750000000000355, -0.2500000000000011102 ) ) ;
#1049=CARTESIAN_POINT ( 'NONE',  ( 3.750000000000000000, 8.312500000000003553, -1.946699141100892705 ) ) ;
#1051=CARTESIAN_POINT ( 'NONE',  ( -1.553300858899107073, 6.937500000000001776, -7.249999999999999112 ) ) ;
#1052=CARTESIAN_POINT ( 'NONE',  ( 3.249999999999998224, 6.312500000000000000, -2.153805922287439945 ) ) ;
#1055=CARTESIAN_POINT ( 'NONE',  ( -3.249999999999999556, 3.187500000000000000, -2.153805922287440833 ) ) ;
#1057=CARTESIAN_POINT ( 'NONE',  ( 3.750000000000000000, 7.750000000000000000, -3.500000000000000444 ) ) ;
#1064=CARTESIAN_POINT ( 'NONE',  ( -2.298097038856278029, 7.625000000000000000, -1.201902961143720638 ) ) ;
#1068=CARTESIAN_POINT ( 'NONE',  ( 0.000000000000000000, 7.499999999999999112, 0.2499999999999998057 ) ) ;
#1072=CARTESIAN_POINT ( 'NONE',  ( 3.249999999999999112, 7.812500000000000000, -2.153805922287439945 ) ) ;
#1073=CARTESIAN_POINT ( 'NONE',  ( -3.750000000000000000, 13.81250000000000178, -5.053300858899105741 ) ) ;
#1081=CARTESIAN_POINT ( 'NONE',  ( 3.249999999999999556, 4.750000000000000000, -3.500000000000000000 ) ) ;
#1083=CARTESIAN_POINT ( 'NONE',  ( -1.346194077712559167, 0.9375000000000002220, -6.749999999999999112 ) ) ;
#1090=CARTESIAN_POINT ( 'NONE',  ( 3.249999999999999556, 13.25000000000000178, -3.500000000000000000 ) ) ;
#1093=CARTESIAN_POINT ( 'NONE',  ( 2.651650429449552870, 1.124999999999999778, -6.151650429449555091 ) ) ;
#1095=CARTESIAN_POINT ( 'NONE',  ( -0.3766621274091715987, 0.5000000000000000000, 0.1491815183709511716 ) ) ;
#1098=CARTESIAN_POINT ( 'NONE',  ( -3.249999999999999556, 14.31250000000000000, -4.846194077712557835 ) ) ;
#1105=DIRECTION ( 'NONE',  ( 0.000000000000000000, -1.000000000000000000, 0.000000000000000000 ) ) ;
#1106=CARTESIAN_POINT ( 'NONE',  ( 1.553300858899108849, 4.937500000000001776, 0.2499999999999993616 ) ) ;
#1107=CARTESIAN_POINT ( 'NONE',  ( -3.750000000000000000, 2.812500000000000444, -5.053300858899105741 ) ) ;
#1109=ORIENTED_EDGE ( 'NONE', *, *, #2808, .T. ) ;
#1111=CARTESIAN_POINT ( 'NONE',  ( 2.298097038856278473, 13.62500000000000000, -5.798097038856279362 ) ) ;
#1116=CARTESIAN_POINT ( 'NONE',  ( -2.298097038856278918, 5.375000000000000000, -5.798097038856277585 ) ) ;
#1122=CARTESIAN_POINT ( 'NONE',  ( 2.298097038856279362, 12.87500000000000178, -1.201902961143720860 ) ) ;
#1124=VERTEX_POINT ( 'NONE', #7016 ) ;
#1126=CARTESIAN_POINT ( 'NONE',  ( 3.749999999999999556, 7.250000000000001776, -3.500000000000000444 ) ) ;
#1127=CARTESIAN_POINT ( 'NONE',  ( 2.298097038856279362, 6.375000000000000888, -1.201902961143720860 ) ) ;
#1130=CARTESIAN_POINT ( 'NONE',  ( 1.346194077712560944, 3.937500000000000000, -0.2500000000000010547 ) ) ;
#1132=CARTESIAN_POINT ( 'NONE',  ( 2.651650429449553759, 9.875000000000000000, -0.8483495705504471296 ) ) ;
#1140=CARTESIAN_POINT ( 'NONE',  ( -3.249999999999999112, 7.687500000000000000, -2.153805922287440833 ) ) ;
#1142=CARTESIAN_POINT ( 'NONE',  ( -2.651650429449552870, 9.875000000000000000, -6.151650429449552426 ) ) ;
#1146=CARTESIAN_POINT ( 'NONE',  ( 1.346194077712561166, 0.4375000000000000555, -0.2500000000000011102 ) ) ;
#1149=CARTESIAN_POINT ( 'NONE',  ( -3.980102097228897245E-16, 14.50000000000000000, -6.749999999999999112 ) ) ;
#1153=CARTESIAN_POINT ( 'NONE',  ( -2.298097038856278473, 4.125000000000000000, -1.201902961143720416 ) ) ;
#1155=CARTESIAN_POINT ( 'NONE',  ( -3.249999999999999112, 8.687499999999998224, -2.153805922287440833 ) ) ;
#1160=CARTESIAN_POINT ( 'NONE',  ( -3.249999999999999556, 0.2500000000000000000, -3.499999999999999556 ) ) ;
#1161=CARTESIAN_POINT ( 'NONE',  ( 3.249999999999999556, 14.25000000000000178, -3.500000000000000000 ) ) ;
#1163=CARTESIAN_POINT ( 'NONE',  ( 1.553300858899105963, 3.062500000000000000, -7.250000000000000888 ) ) ;
#1170=CARTESIAN_POINT ( 'NONE',  ( -1.346194077712559389, 13.06250000000000000, -0.2500000000000002220 ) ) ;
#1177=CARTESIAN_POINT ( 'NONE',  ( -1.553300858899107295, 4.437500000000000888, -7.250000000000000000 ) ) ;
#1178=CARTESIAN_POINT ( 'NONE',  ( -3.750000000000000000, 3.687500000000000444, -1.946699141100893149 ) ) ;
#1181=CARTESIAN_POINT ( 'NONE',  ( 3.249999999999999556, 2.249999999999999556, -3.500000000000000000 ) ) ;
#1184=SHAPE_REPRESENTATION_RELATIONSHIP ( 'NONE' , 'NONE' ,  #9314, #2810 ) ;
#1185=CARTESIAN_POINT ( 'NONE',  ( -3.249999999999999556, 5.312500000000001776, -4.846194077712557835 ) ) ;
#1191=CARTESIAN_POINT ( 'NONE',  ( 1.346194077712558279, 13.56250000000000000, -6.750000000000000000 ) ) ;
#1195=CARTESIAN_POINT ( 'NONE',  ( 3.750000000000000000, 4.312500000000000000, -1.946699141100892705 ) ) ;
#1196=CARTESIAN_POINT ( 'NONE',  ( -3.980102097228897738E-16, 7.000000000000000000, -6.749999999999999112 ) ) ;
#1197=ORIENTED_EDGE ( 'NONE', *, *, #3286, .F. ) ;
#1199=CARTESIAN_POINT ( 'NONE',  ( 3.249999999999998668, 2.687500000000000888, -4.846194077712560500 ) ) ;
#1208=CARTESIAN_POINT ( 'NONE',  ( -1.553300858899106629, 11.56250000000000178, 0.2499999999999998335 ) ) ;
#1211=CARTESIAN_POINT ( 'NONE',  ( -3.249999999999999112, 2.687500000000000888, -2.153805922287440833 ) ) ;
#1220=CARTESIAN_POINT ( 'NONE',  ( 1.346194077712558279, 1.562500000000000000, -6.750000000000000000 ) ) ;
#1223=CARTESIAN_POINT ( 'NONE',  ( -2.298097038856278029, 5.625000000000000888, -1.201902961143720638 ) ) ;
#1224=ORIENTED_EDGE ( 'NONE', *, *, #8081, .T. ) ;
#1230=CARTESIAN_POINT ( 'NONE',  ( -1.346194077712559389, 1.437500000000000000, -6.749999999999999112 ) ) ;
#1232=CARTESIAN_POINT ( 'NONE',  ( -1.553300858899106629, 1.562500000000000222, 0.2499999999999998335 ) ) ;
#1234=CARTESIAN_POINT ( 'NONE',  ( 2.651650429449553759, 4.875000000000000000, -0.8483495705504471296 ) ) ;
#1236=CARTESIAN_POINT ( 'NONE',  ( 1.553300858899105963, 4.062500000000001776, -7.250000000000000888 ) ) ;
#1242=CARTESIAN_POINT ( 'NONE',  ( -1.346194077712559389, 11.06250000000000000, -0.2500000000000002220 ) ) ;
#1244=CIRCLE ( 'NONE', #12616, 0.2500000000000002220 ) ;
#1247=VECTOR ( 'NONE', #11189, 1000.000000000000000 ) ;
#1252=CARTESIAN_POINT ( 'NONE',  ( 1.553300858899105963, 3.562500000000000444, -7.250000000000000888 ) ) ;
#1253=CARTESIAN_POINT ( 'NONE',  ( -1.553300858899107073, 5.937500000000000000, -7.249999999999999112 ) ) ;
#1254=CARTESIAN_POINT ( 'NONE',  ( -0.3766621274091715987, 0.5000000000000000000, -6.863050255469941519 ) ) ;
#1258=CARTESIAN_POINT ( 'NONE',  ( 2.298097038856279362, 1.375000000000000000, -1.201902961143720860 ) ) ;
#1263=CARTESIAN_POINT ( 'NONE',  ( -3.249999999999999556, 4.250000000000000000, -3.499999999999999556 ) ) ;
#1269=CARTESIAN_POINT ( 'NONE',  ( -3.249999999999999556, 13.25000000000000000, -3.499999999999999556 ) ) ;
#1274=CARTESIAN_POINT ( 'NONE',  ( -1.553300858899107073, 3.937500000000001332, -7.249999999999999112 ) ) ;
#1275=CARTESIAN_POINT ( 'NONE',  ( 0.000000000000000000, 12.50000000000000178, -0.2500000000000002220 ) ) ;
#1278=CARTESIAN_POINT ( 'NONE',  ( 3.249999999999999112, 4.812500000000000888, -2.153805922287439945 ) ) ;
#1287=ORIENTED_EDGE ( 'NONE', *, *, #6290, .F. ) ;
#1291=CARTESIAN_POINT ( 'NONE',  ( 3.749999999999999556, 14.25000000000000178, -3.500000000000000444 ) ) ;
#1297=CARTESIAN_POINT ( 'NONE',  ( 3.249999999999998224, 2.312500000000000000, -2.153805922287439945 ) ) ;
#1304=CARTESIAN_POINT ( 'NONE',  ( 3.249999999999998668, 3.687500000000000444, -4.846194077712560500 ) ) ;
#1307=CARTESIAN_POINT ( 'NONE',  ( 3.249999999999999556, 7.250000000000001776, -3.500000000000000000 ) ) ;
#1312=CARTESIAN_POINT ( 'NONE',  ( -3.980102097228897245E-16, 0.5000000000000000000, -6.749999999999999112 ) ) ;
#1313=CARTESIAN_POINT ( 'NONE',  ( -3.749999999999999556, 2.750000000000000444, -3.499999999999999112 ) ) ;
#1314=CARTESIAN_POINT ( 'NONE',  ( 3.749999999999999112, 5.687500000000000000, -5.053300858899108405 ) ) ;
#1317=CARTESIAN_POINT ( 'NONE',  ( -2.651650429449552870, 5.625000000000000888, -0.8483495705504463524 ) ) ;
#1320=VECTOR ( 'NONE', #10549, 1000.000000000000000 ) ;
#1325=CARTESIAN_POINT ( 'NONE',  ( 2.298097038856278473, 10.62500000000000000, -5.798097038856279362 ) ) ;
#1329=CARTESIAN_POINT ( 'NONE',  ( -2.651650429449553314, 7.874999999999999112, -6.151650429449552426 ) ) ;
#1334=CARTESIAN_POINT ( 'NONE',  ( 2.651650429449553759, 6.875000000000000000, -0.8483495705504471296 ) ) ;
#1335=CARTESIAN_POINT ( 'NONE',  ( 0.000000000000000000, 4.499999999999999112, 0.2499999999999998057 ) ) ;
#1339=CARTESIAN_POINT ( 'NONE',  ( -2.298097038856279362, 2.875000000000000000, -5.798097038856278473 ) ) ;
#1343=CARTESIAN_POINT ( 'NONE',  ( -1.346194077712559389, 9.062499999999998224, -0.2500000000000002220 ) ) ;
#1354=CARTESIAN_POINT ( 'NONE',  ( -2.651650429449553314, 6.875000000000000000, -6.151650429449552426 ) ) ;
#1355=CARTESIAN_POINT ( 'NONE',  ( 3.249999999999999556, 9.249999999999998224, -3.500000000000000000 ) ) ;
#1359=CARTESIAN_POINT ( 'NONE',  ( 2.298097038856279362, 5.875000000000000000, -1.201902961143720860 ) ) ;
#1367=CARTESIAN_POINT ( 'NONE',  ( 1.346194077712558057, 9.562500000000000000, -6.750000000000000000 ) ) ;
#1370=CARTESIAN_POINT ( 'NONE',  ( 1.553300858899105963, 13.06250000000000178, -7.249999999999999112 ) ) ;
#1375=CARTESIAN_POINT ( 'NONE',  ( 1.346194077712558279, 2.062500000000000000, -6.750000000000000888 ) ) ;
#1383=CARTESIAN_POINT ( 'NONE',  ( -3.249999999999999556, 7.187500000000000000, -2.153805922287440833 ) ) ;
#1386=CARTESIAN_POINT ( 'NONE',  ( -3.249999999999999556, 0.7499999999999998890, -3.500000000000000000 ) ) ;
#1387=CARTESIAN_POINT ( 'NONE',  ( -3.249999999999999112, 6.812500000000001776, -4.846194077712558723 ) ) ;
#1392=CARTESIAN_POINT ( 'NONE',  ( 0.000000000000000000, 2.500000000000000000, 0.2499999999999998057 ) ) ;
#1393=CARTESIAN_POINT ( 'NONE',  ( -2.651650429449552870, 6.125000000000000000, -0.8483495705504462414 ) ) ;
#1395=CARTESIAN_POINT ( 'NONE',  ( -2.651650429449552870, 4.625000000000000888, -0.8483495705504463524 ) ) ;
#1399=CARTESIAN_POINT ( 'NONE',  ( 2.298097038856279362, 13.87500000000000000, -1.201902961143720860 ) ) ;
#1406=CARTESIAN_POINT ( 'NONE',  ( 3.749999999999999112, 10.18750000000000533, -5.053300858899108405 ) ) ;
#1410=CARTESIAN_POINT ( 'NONE',  ( 1.553300858899105963, 10.56250000000000000, -7.250000000000000888 ) ) ;
#1411=CARTESIAN_POINT ( 'NONE',  ( -1.553300858899107073, 3.937500000000000444, -7.249999999999999112 ) ) ;
#1414=CARTESIAN_POINT ( 'NONE',  ( 1.346194077712558279, 5.062500000000000000, -6.750000000000000888 ) ) ;
#1415=CARTESIAN_POINT ( 'NONE',  ( -3.750000000000000000, 8.250000000000000000, -3.499999999999999112 ) ) ;
#1420=CARTESIAN_POINT ( 'NONE',  ( -3.249999999999999556, 6.312500000000000888, -4.846194077712557835 ) ) ;
#1425=VERTEX_POINT ( 'NONE', #8399 ) ;
#1431=CARTESIAN_POINT ( 'NONE',  ( -4.592425496802573972E-16, 11.00000000000000178, -7.250000000000000000 ) ) ;
#1432=CARTESIAN_POINT ( 'NONE',  ( 1.346194077712561166, 7.437499999999999112, -0.2500000000000011102 ) ) ;
#1433=CARTESIAN_POINT ( 'NONE',  ( -2.298097038856278029, 11.62500000000000000, -1.201902961143720638 ) ) ;
#1436=CARTESIAN_POINT ( 'NONE',  ( -1.346194077712559389, 6.437500000000000888, -6.749999999999999112 ) ) ;
#1443=CARTESIAN_POINT ( 'NONE',  ( -3.249999999999999556, 2.250000000000000444, -3.499999999999999556 ) ) ;
#1445=CARTESIAN_POINT ( 'NONE',  ( 3.749999999999999112, 15.31250000000000355, -1.946699141100893149 ) ) ;
#1449=CARTESIAN_POINT ( 'NONE',  ( 3.249999999999998224, 3.312500000000000000, -2.153805922287439945 ) ) ;
#1456=CARTESIAN_POINT ( 'NONE',  ( -1.346194077712559167, 6.437500000000000888, -6.749999999999999112 ) ) ;
#1458=CARTESIAN_POINT ( 'NONE',  ( -2.298097038856278029, 0.6249999999999998890, -1.201902961143720638 ) ) ;
#1459=CARTESIAN_POINT ( 'NONE',  ( 2.298097038856279362, 5.375000000000000888, -1.201902961143720860 ) ) ;
#1461=LINE ( 'NONE', #2393, #4547 ) ;
#1463=CARTESIAN_POINT ( 'NONE',  ( -3.980102097228897245E-16, 5.500000000000000000, -6.749999999999999112 ) ) ;
#1464=CARTESIAN_POINT ( 'NONE',  ( -3.980102097228897738E-16, 15.00000000000000178, -6.749999999999999112 ) ) ;
#1465=CARTESIAN_POINT ( 'NONE',  ( 3.749999999999999112, 6.687500000000000888, -5.053300858899108405 ) ) ;
#1466=CARTESIAN_POINT ( 'NONE',  ( 3.749999999999999112, 8.187500000000000000, -5.053300858899108405 ) ) ;
#1474=CARTESIAN_POINT ( 'NONE',  ( 0.3766621274091721538, 0.3292059843107342232, -7.146945437571387671 ) ) ;
#1477=CARTESIAN_POINT ( 'NONE',  ( -4.592425496802573972E-16, 8.000000000000000000, -7.250000000000000000 ) ) ;
#1481=CARTESIAN_POINT ( 'NONE',  ( 3.749999999999998668, 8.687500000000000000, -5.053300858899107517 ) ) ;
#1482=CARTESIAN_POINT ( 'NONE',  ( 3.749999999999999112, 6.312500000000000000, -1.946699141100893149 ) ) ;
#1485=DIRECTION ( 'NONE',  ( -0.000000000000000000, -1.000000000000000000, -0.000000000000000000 ) ) ;
#1487=CARTESIAN_POINT ( 'NONE',  ( 0.000000000000000000, 3.500000000000000000, -0.2500000000000002220 ) ) ;
#1489=CARTESIAN_POINT ( 'NONE',  ( -1.553300858899107295, 11.43750000000000000, -7.250000000000000000 ) ) ;
#1492=EDGE_CURVE ( 'NONE', #4560, #559, #12979, .T. ) ;
#1496=CARTESIAN_POINT ( 'NONE',  ( -3.980102097228897245E-16, 7.500000000000000000, -6.749999999999999112 ) ) ;
#1497=VECTOR ( 'NONE', #9994, 1000.000000000000000 ) ;
#1503=CARTESIAN_POINT ( 'NONE',  ( -0.3766621274091715987, 0.5000000000000000000, 0.1491815183709511716 ) ) ;
#1504=CARTESIAN_POINT ( 'NONE',  ( -1.346194077712559167, 14.43750000000000000, -6.749999999999999112 ) ) ;
#1508=CARTESIAN_POINT ( 'NONE',  ( 3.749999999999999556, 14.25000000000000178, -3.500000000000000444 ) ) ;
#1509=CARTESIAN_POINT ( 'NONE',  ( 2.298097038856278029, 11.12500000000000178, -5.798097038856279362 ) ) ;
#1510=CARTESIAN_POINT ( 'NONE',  ( -3.249999999999999112, 10.68750000000000178, -2.153805922287440833 ) ) ;
#1514=CARTESIAN_POINT ( 'NONE',  ( -1.346194077712559389, 8.062500000000000000, -0.2500000000000002220 ) ) ;
#1524=CARTESIAN_POINT ( 'NONE',  ( -1.346194077712559389, 2.437500000000000444, -6.749999999999999112 ) ) ;
#1525=CARTESIAN_POINT ( 'NONE',  ( 2.651650429449553759, 11.87500000000000000, -0.8483495705504471296 ) ) ;
#1526=CARTESIAN_POINT ( 'NONE',  ( -0.3766621274091715987, -0.2500000000000000000, -0.1347136637304948981 ) ) ;
#1527=CARTESIAN_POINT ( 'NONE',  ( 2.651650429449552870, 15.12500000000000000, -6.151650429449553314 ) ) ;
#1536=CARTESIAN_POINT ( 'NONE',  ( -3.249999999999999556, 7.312500000000000000, -4.846194077712557835 ) ) ;
#1539=CARTESIAN_POINT ( 'NONE',  ( -3.980102097228897245E-16, 14.50000000000000000, -6.749999999999999112 ) ) ;
#1540=CARTESIAN_POINT ( 'NONE',  ( 2.298097038856279362, 9.374999999999998224, -1.201902961143720860 ) ) ;
#1545=CARTESIAN_POINT ( 'NONE',  ( 3.249999999999999556, 5.750000000000000000, -3.500000000000000000 ) ) ;
#1546=CARTESIAN_POINT ( 'NONE',  ( 3.749999999999999112, 1.312500000000000000, -1.946699141100893149 ) ) ;
#1547=CARTESIAN_POINT ( 'NONE',  ( -4.592425496802573972E-16, 3.500000000000000000, -7.249999999999999112 ) ) ;
#1549=CARTESIAN_POINT ( 'NONE',  ( -1.553300858899106629, 6.562500000000000888, 0.2500000000000002220 ) ) ;
#1555=CARTESIAN_POINT ( 'NONE',  ( 0.000000000000000000, 15.00000000000000000, -0.2500000000000002220 ) ) ;
#1559=CARTESIAN_POINT ( 'NONE',  ( 0.000000000000000000, 14.50000000000000000, 0.2500000000000002220 ) ) ;
#1563=CARTESIAN_POINT ( 'NONE',  ( -1.553300858899107295, 9.437500000000000000, -7.250000000000000000 ) ) ;
#1564=CARTESIAN_POINT ( 'NONE',  ( -1.553300858899107073, 8.937500000000000000, -7.249999999999999112 ) ) ;
#1569=CARTESIAN_POINT ( 'NONE',  ( -2.298097038856279362, 3.875000000000000444, -5.798097038856278473 ) ) ;
#1570=CARTESIAN_POINT ( 'NONE',  ( -3.750000000000000000, 9.250000000000000000, -3.499999999999999112 ) ) ;
#1573=CARTESIAN_POINT ( 'NONE',  ( -3.249999999999999556, 7.187500000000000000, -2.153805922287440833 ) ) ;
#1587=CARTESIAN_POINT ( 'NONE',  ( -1.553300858899106629, 11.56250000000000178, 0.2499999999999998335 ) ) ;
#1588=CARTESIAN_POINT ( 'NONE',  ( -1.346194077712559167, 9.937500000000001776, -6.749999999999999112 ) ) ;
#1590=CARTESIAN_POINT ( 'NONE',  ( -2.298097038856279362, 10.87499999999999822, -5.798097038856278473 ) ) ;
#1593=CARTESIAN_POINT ( 'NONE',  ( -2.298097038856278473, 6.125000000000000000, -1.201902961143720416 ) ) ;
#1601=CARTESIAN_POINT ( 'NONE',  ( -3.980102097228897245E-16, 1.500000000000000000, -6.749999999999999112 ) ) ;
#1603=CARTESIAN_POINT ( 'NONE',  ( -2.651650429449553314, 13.37500000000000000, -6.151650429449552426 ) ) ;
#1607=CARTESIAN_POINT ( 'NONE',  ( -3.750000000000000000, 2.250000000000000444, -3.499999999999999112 ) ) ;
#1610=CARTESIAN_POINT ( 'NONE',  ( -1.553300858899107073, 1.437500000000000000, -7.250000000000000000 ) ) ;
#1614=ORIENTED_EDGE ( 'NONE', *, *, #3097, .T. ) ;
#1616=CARTESIAN_POINT ( 'NONE',  ( 3.249999999999999112, 5.812500000000000000, -2.153805922287439945 ) ) ;
#1618=CARTESIAN_POINT ( 'NONE',  ( 1.346194077712558057, 14.56250000000000000, -6.750000000000000000 ) ) ;
#1619=CARTESIAN_POINT ( 'NONE',  ( 3.249999999999999556, 10.25000000000000178, -3.500000000000000000 ) ) ;
#1623=CARTESIAN_POINT ( 'NONE',  ( 1.346194077712560944, 2.937500000000000444, -0.2500000000000010547 ) ) ;
#1624=CARTESIAN_POINT ( 'NONE',  ( -1.553300858899106629, 5.562500000000000000, 0.2499999999999998335 ) ) ;
#1625=CARTESIAN_POINT ( 'NONE',  ( 3.750000000000000000, 8.750000000000000000, -3.500000000000000444 ) ) ;
#1627=CARTESIAN_POINT ( 'NONE',  ( -2.651650429449553314, 4.875000000000000000, -6.151650429449552426 ) ) ;
#1634=CARTESIAN_POINT ( 'NONE',  ( 0.000000000000000000, -0.4999999999999999445, -0.2500000000000002220 ) ) ;
#1636=CARTESIAN_POINT ( 'NONE',  ( 0.3766621274091715987, 0.5000000000000000000, -0.1347136637304948981 ) ) ;
#1638=CARTESIAN_POINT ( 'NONE',  ( -3.750000000000000000, 10.25000000000000000, -3.499999999999999112 ) ) ;
#1639=CARTESIAN_POINT ( 'NONE',  ( -3.750000000000000000, 8.687500000000003553, -1.946699141100893149 ) ) ;
#1643=CARTESIAN_POINT ( 'NONE',  ( -3.249999999999999556, 3.750000000000000444, -3.500000000000000000 ) ) ;
#1645=CARTESIAN_POINT ( 'NONE',  ( -2.651650429449553314, 11.37500000000000000, -6.151650429449552426 ) ) ;
#1649=CARTESIAN_POINT ( 'NONE',  ( 3.249999999999999556, 8.750000000000000000, -3.500000000000000000 ) ) ;
#1653=CARTESIAN_POINT ( 'NONE',  ( -0.3766621274091715987, -0.2500000000000000000, -7.146945437571387671 ) ) ;
#1654=DIRECTION ( 'NONE',  ( 0.000000000000000000, 1.000000000000000000, -0.000000000000000000 ) ) ;
#1658=CARTESIAN_POINT ( 'NONE',  ( 3.749999999999999112, 11.31250000000000355, -1.946699141100893149 ) ) ;
#1659=CARTESIAN_POINT ( 'NONE',  ( 0.000000000000000000, 10.50000000000000000, -0.2500000000000002220 ) ) ;
#1660=CARTESIAN_POINT ( 'NONE',  ( 3.249999999999998224, 13.18750000000000000, -4.846194077712561388 ) ) ;
#1663=CARTESIAN_POINT ( 'NONE',  ( 1.346194077712558057, 6.562500000000000000, -6.750000000000000000 ) ) ;
#1672=CARTESIAN_POINT ( 'NONE',  ( -1.346194077712559389, 0.4375000000000000555, -6.749999999999999112 ) ) ;
#1673=CARTESIAN_POINT ( 'NONE',  ( 0.000000000000000000, -0.4999999999999999445, 0.2500000000000002220 ) ) ;
#1676=CARTESIAN_POINT ( 'NONE',  ( -3.749999999999999556, 1.187500000000000444, -1.946699141100892927 ) ) ;
#1680=CARTESIAN_POINT ( 'NONE',  ( -3.750000000000000000, 2.250000000000000444, -3.499999999999999112 ) ) ;
#1681=EDGE_CURVE ( 'NONE', #9756, #1124, #614, .T. ) ;
#1687=CARTESIAN_POINT ( 'NONE',  ( -3.249999999999999556, 6.312500000000000000, -4.846194077712557835 ) ) ;
#1689=CARTESIAN_POINT ( 'NONE',  ( -3.249999999999999556, 13.31250000000000000, -4.846194077712557835 ) ) ;
#1690=CARTESIAN_POINT ( 'NONE',  ( -1.346194077712558945, 12.56250000000000355, -0.2500000000000002220 ) ) ;
#1693=CARTESIAN_POINT ( 'NONE',  ( 0.000000000000000000, 3.000000000000000000, -0.2500000000000002220 ) ) ;
#1694=CARTESIAN_POINT ( 'NONE',  ( -4.592425496802573972E-16, 5.000000000000000000, -7.250000000000000000 ) ) ;
#1695=CARTESIAN_POINT ( 'NONE',  ( 2.651650429449553759, 10.87500000000000178, -0.8483495705504471296 ) ) ;
#1698=CARTESIAN_POINT ( 'NONE',  ( 3.749999999999999556, 10.25000000000000178, -3.500000000000000444 ) ) ;
#1706=CARTESIAN_POINT ( 'NONE',  ( 3.750000000000000000, 12.31250000000000178, -1.946699141100892705 ) ) ;
#1710=CARTESIAN_POINT ( 'NONE',  ( -3.749999999999999556, 10.18750000000000000, -1.946699141100892927 ) ) ;
#1711=CARTESIAN_POINT ( 'NONE',  ( -1.553300858899107073, 7.937500000000001776, -7.249999999999999112 ) ) ;
#1714=CARTESIAN_POINT ( 'NONE',  ( 3.249999999999998224, 9.187500000000001776, -4.846194077712561388 ) ) ;
#1715=CARTESIAN_POINT ( 'NONE',  ( -3.750000000000000000, 14.25000000000000000, -3.499999999999999112 ) ) ;
#1719=CARTESIAN_POINT ( 'NONE',  ( -1.346194077712559389, 12.06250000000000000, -0.2500000000000002220 ) ) ;
#1727=ORIENTED_EDGE ( 'NONE', *, *, #1492, .F. ) ;
#1733=CARTESIAN_POINT ( 'NONE',  ( 1.553300858899109071, 11.43750000000000178, 0.2499999999999989175 ) ) ;
#1734=CARTESIAN_POINT ( 'NONE',  ( 3.249999999999998224, 12.18750000000000178, -4.846194077712561388 ) ) ;
#1735=CARTESIAN_POINT ( 'NONE',  ( -2.298097038856278029, 12.62500000000000000, -1.201902961143720638 ) ) ;
#1737=CARTESIAN_POINT ( 'NONE',  ( 0.000000000000000000, 13.00000000000000178, -0.2500000000000002220 ) ) ;
#1747=AXIS2_PLACEMENT_3D ( 'NONE', #1503, #9773, #13259 ) ;
#1749=CARTESIAN_POINT ( 'NONE',  ( -3.249999999999999556, 5.250000000000000000, -3.499999999999999556 ) ) ;
#1750=CARTESIAN_POINT ( 'NONE',  ( 3.749999999999999112, 13.81250000000000000, -1.946699141100892039 ) ) ;
#1754=ADVANCED_FACE ( 'NONE', ( #9954 ), #14844, .T. ) ;
#1756=CARTESIAN_POINT ( 'NONE',  ( 3.749999999999998668, 0.6875000000000000000, -5.053300858899107517 ) ) ;
#1765=CARTESIAN_POINT ( 'NONE',  ( -2.298097038856278918, 10.37500000000000000, -5.798097038856277585 ) ) ;
#1767=CARTESIAN_POINT ( 'NONE',  ( 3.249999999999998224, 3.312500000000000000, -2.153805922287439945 ) ) ;
#1769=CARTESIAN_POINT ( 'NONE',  ( -3.249999999999999556, 12.74999999999999822, -3.500000000000000000 ) ) ;
#1774=CARTESIAN_POINT ( 'NONE',  ( -3.249999999999999556, 3.187500000000000000, -2.153805922287440833 ) ) ;
#1775=CARTESIAN_POINT ( 'NONE',  ( 2.651650429449553314, 5.375000000000000000, -0.8483495705504476847 ) ) ;
#1776=CARTESIAN_POINT ( 'NONE',  ( -3.750000000000000000, 11.31249999999999822, -5.053300858899105741 ) ) ;
#1780=CARTESIAN_POINT ( 'NONE',  ( -1.553300858899107073, 9.937500000000001776, -7.249999999999999112 ) ) ;
#1788=CARTESIAN_POINT ( 'NONE',  ( 0.000000000000000000, 12.50000000000000178, 0.2500000000000002220 ) ) ;
#1792=CARTESIAN_POINT ( 'NONE',  ( -2.651650429449552870, 6.625000000000000000, -0.8483495705504467965 ) ) ;
#1798=CARTESIAN_POINT ( 'NONE',  ( -2.298097038856278029, 6.625000000000000000, -1.201902961143720638 ) ) ;
#1800=CARTESIAN_POINT ( 'NONE',  ( -3.749999999999999556, 12.18750000000000000, -1.946699141100892927 ) ) ;
#1805=CARTESIAN_POINT ( 'NONE',  ( 2.298097038856279362, 11.87500000000000000, -1.201902961143720860 ) ) ;
#1810=CARTESIAN_POINT ( 'NONE',  ( 0.000000000000000000, 3.061616997868383018E-17, -0.1347136637304948981 ) ) ;
#1814=CARTESIAN_POINT ( 'NONE',  ( -2.651650429449552870, 2.125000000000000000, -0.8483495705504462414 ) ) ;
#1816=CARTESIAN_POINT ( 'NONE',  ( -3.249999999999999556, 9.750000000000000000, -3.500000000000000000 ) ) ;
#1817=CARTESIAN_POINT ( 'NONE',  ( -2.298097038856278918, 0.3750000000000000000, -5.798097038856277585 ) ) ;
#1819=CARTESIAN_POINT ( 'NONE',  ( -1.346194077712559389, 10.43750000000000000, -6.749999999999999112 ) ) ;
#1831=CARTESIAN_POINT ( 'NONE',  ( -2.298097038856278918, 3.375000000000000000, -5.798097038856277585 ) ) ;
#1833=CARTESIAN_POINT ( 'NONE',  ( -3.750000000000000000, 12.25000000000000000, -3.499999999999999112 ) ) ;
#1838=CARTESIAN_POINT ( 'NONE',  ( -3.749999999999999556, 3.187500000000000000, -1.946699141100892927 ) ) ;
#1842=CARTESIAN_POINT ( 'NONE',  ( -3.750000000000000000, 0.3125000000000000555, -5.053300858899105741 ) ) ;
#1850=CARTESIAN_POINT ( 'NONE',  ( -3.980102097228897738E-16, 2.000000000000000000, -6.749999999999999112 ) ) ;
#1851=CARTESIAN_POINT ( 'NONE',  ( -2.298097038856279362, 8.874999999999996447, -5.798097038856278473 ) ) ;
#1855=CARTESIAN_POINT ( 'NONE',  ( 2.298097038856279362, 6.875000000000000000, -1.201902961143720860 ) ) ;
#1856=CARTESIAN_POINT ( 'NONE',  ( -2.651650429449552870, 3.625000000000000888, -0.8483495705504467965 ) ) ;
#1857=CARTESIAN_POINT ( 'NONE',  ( 2.651650429449553759, 8.875000000000001776, -0.8483495705504471296 ) ) ;
#1860=CARTESIAN_POINT ( 'NONE',  ( 2.651650429449554203, 10.37500000000000000, -0.8483495705504471296 ) ) ;
#1863=ADVANCED_FACE ( 'NONE', ( #4320 ), #9023, .F. ) ;
#1868=CARTESIAN_POINT ( 'NONE',  ( -2.298097038856278473, 0.1250000000000000000, -1.201902961143720416 ) ) ;
#1870=CARTESIAN_POINT ( 'NONE',  ( -2.651650429449552870, 13.62500000000000000, -0.8483495705504463524 ) ) ;
#1875=CARTESIAN_POINT ( 'NONE',  ( -3.249999999999999556, 10.18750000000000000, -2.153805922287440833 ) ) ;
#1877=CARTESIAN_POINT ( 'NONE',  ( 2.298097038856279362, 8.375000000000000000, -1.201902961143720860 ) ) ;
#1879=CARTESIAN_POINT ( 'NONE',  ( 3.749999999999998668, 13.68750000000000000, -5.053300858899107517 ) ) ;
#1882=CARTESIAN_POINT ( 'NONE',  ( 3.249999999999998668, 13.68750000000000000, -4.846194077712560500 ) ) ;
#1886=CARTESIAN_POINT ( 'NONE',  ( 3.249999999999998668, 7.687500000000000000, -4.846194077712560500 ) ) ;
#1891=CARTESIAN_POINT ( 'NONE',  ( -3.749999999999999556, 0.1875000000000001110, -1.946699141100892927 ) ) ;
#1892=CARTESIAN_POINT ( 'NONE',  ( 3.249999999999998224, 15.31250000000000355, -2.153805922287439945 ) ) ;
#1893=CARTESIAN_POINT ( 'NONE',  ( 1.346194077712561166, 14.43750000000000178, -0.2500000000000011102 ) ) ;
#1895=CARTESIAN_POINT ( 'NONE',  ( -3.249999999999999556, 12.18750000000000000, -2.153805922287440833 ) ) ;
#1905=CARTESIAN_POINT ( 'NONE',  ( 1.346194077712560944, 4.937500000000001776, -0.2500000000000010547 ) ) ;
#1907=CARTESIAN_POINT ( 'NONE',  ( 0.000000000000000000, 3.500000000000000000, 0.2500000000000002220 ) ) ;
#1908=VECTOR ( 'NONE', #3112, 1000.000000000000000 ) ;
#1912=CARTESIAN_POINT ( 'NONE',  ( 3.750000000000000000, 3.750000000000000000, -3.500000000000000444 ) ) ;
#1915=CARTESIAN_POINT ( 'NONE',  ( -1.553300858899106407, 2.062500000000000000, 0.2500000000000002220 ) ) ;
#1921=CARTESIAN_POINT ( 'NONE',  ( 2.298097038856279362, 4.375000000000000000, -1.201902961143720860 ) ) ;
#1925=CARTESIAN_POINT ( 'NONE',  ( -2.651650429449552870, 5.625000000000000000, -0.8483495705504467965 ) ) ;
#1926=CARTESIAN_POINT ( 'NONE',  ( -1.553300858899106407, 10.06250000000000000, 0.2500000000000002220 ) ) ;
#1928=ORIENTED_EDGE ( 'NONE', *, *, #10523, .T. ) ;
#1930=CARTESIAN_POINT ( 'NONE',  ( 3.749999999999999112, 11.18750000000000178, -5.053300858899108405 ) ) ;
#1938=CARTESIAN_POINT ( 'NONE',  ( -1.346194077712559167, 3.937500000000001332, -6.749999999999999112 ) ) ;
#1945=CARTESIAN_POINT ( 'NONE',  ( -3.249999999999999556, 7.750000000000000888, -3.500000000000000000 ) ) ;
#1947=CARTESIAN_POINT ( 'NONE',  ( -2.651650429449553314, 13.37500000000000000, -6.151650429449552426 ) ) ;
#1950=CARTESIAN_POINT ( 'NONE',  ( -3.980102097228897245E-16, 10.50000000000000000, -6.749999999999999112 ) ) ;
#1952=CARTESIAN_POINT ( 'NONE',  ( 3.249999999999998668, 9.687500000000000000, -4.846194077712560500 ) ) ;
#1959=CARTESIAN_POINT ( 'NONE',  ( -1.553300858899107073, 14.93750000000000000, -7.249999999999999112 ) ) ;
#1960=CARTESIAN_POINT ( 'NONE',  ( 1.553300858899105963, 1.062500000000000444, -7.249999999999999112 ) ) ;
#1961=CARTESIAN_POINT ( 'NONE',  ( 2.298097038856278473, 1.625000000000000222, -5.798097038856279362 ) ) ;
#1964=CARTESIAN_POINT ( 'NONE',  ( -3.249999999999999556, 12.25000000000000000, -3.499999999999999556 ) ) ;
#1967=FACE_OUTER_BOUND ( 'NONE', #863, .T. ) ;
#1976=ORIENTED_EDGE ( 'NONE', *, *, #12128, .F. ) ;
#1977=CARTESIAN_POINT ( 'NONE',  ( -3.249999999999999556, 3.250000000000000444, -3.499999999999999556 ) ) ;
#1979=CARTESIAN_POINT ( 'NONE',  ( -3.750000000000000000, 3.687500000000000444, -1.946699141100893149 ) ) ;
#1985=CARTESIAN_POINT ( 'NONE',  ( -4.592425496802573972E-16, 7.500000000000000000, -7.249999999999999112 ) ) ;
#1988=CARTESIAN_POINT ( 'NONE',  ( -3.750000000000000000, 3.312500000000000000, -5.053300858899105741 ) ) ;
#1995=CARTESIAN_POINT ( 'NONE',  ( 3.249999999999999556, 5.249999999999999112, -3.500000000000000000 ) ) ;
#1998=CIRCLE ( 'NONE', #13078, 0.2500000000000002220 ) ;
#1999=CARTESIAN_POINT ( 'NONE',  ( -1.553300858899106629, 10.56250000000000355, 0.2499999999999998335 ) ) ;
#2002=CARTESIAN_POINT ( 'NONE',  ( -4.592425496802573972E-16, 13.50000000000000000, -7.249999999999999112 ) ) ;
#2006=CARTESIAN_POINT ( 'NONE',  ( 1.346194077712558057, 8.562500000000001776, -6.750000000000000000 ) ) ;
#2007=CARTESIAN_POINT ( 'NONE',  ( -2.651650429449553314, 9.875000000000000000, -6.151650429449552426 ) ) ;
#2017=CARTESIAN_POINT ( 'NONE',  ( 0.000000000000000000, 3.500000000000000000, -0.2500000000000002220 ) ) ;
#2024=CARTESIAN_POINT ( 'NONE',  ( -3.980102097228897738E-16, 14.00000000000000000, -6.749999999999999112 ) ) ;
#2026=CARTESIAN_POINT ( 'NONE',  ( -3.749999999999999556, 14.31250000000000000, -5.053300858899104853 ) ) ;
#2027=CARTESIAN_POINT ( 'NONE',  ( -0.3766621274091715987, 0.2613176957160640579, -6.863050255469941519 ) ) ;
#2029=CARTESIAN_POINT ( 'NONE',  ( 0.000000000000000000, 14.00000000000000000, -0.2500000000000002220 ) ) ;
#2033=CARTESIAN_POINT ( 'NONE',  ( -1.346194077712559389, 9.062499999999998224, -0.2500000000000002220 ) ) ;
#2040=CARTESIAN_POINT ( 'NONE',  ( 1.553300858899108849, 0.9374999999999998890, 0.2499999999999993616 ) ) ;
#2041=CARTESIAN_POINT ( 'NONE',  ( 1.346194077712561166, 13.43750000000000355, -0.2500000000000011102 ) ) ;
#2044=CARTESIAN_POINT ( 'NONE',  ( 1.346194077712560944, 9.937499999999998224, -0.2500000000000010547 ) ) ;
#2056=CARTESIAN_POINT ( 'NONE',  ( -3.980102097228897245E-16, 11.50000000000000000, -6.749999999999999112 ) ) ;
#2057=EDGE_LOOP ( 'NONE', ( #1614, #6032, #7142, #9980, #14410, #900, #13890, #5734 ) ) ;
#2058=CARTESIAN_POINT ( 'NONE',  ( -1.346194077712559389, 3.437500000000000000, -6.749999999999999112 ) ) ;
#2060=CARTESIAN_POINT ( 'NONE',  ( 2.651650429449554203, 2.375000000000000000, -0.8483495705504471296 ) ) ;
#2064=CARTESIAN_POINT ( 'NONE',  ( -1.553300858899107295, 6.437500000000000888, -7.250000000000000000 ) ) ;
#2067=B_SPLINE_CURVE_WITH_KNOTS ( 'NONE', 3,
 ( #11597, #3483, #2255, #2104 ),
 .UNSPECIFIED., .F., .F.,
 ( 4, 4 ),
 ( 0.000000000000000000, 0.0003026718941486676129 ),
 .UNSPECIFIED. ) ;
#2076=CARTESIAN_POINT ( 'NONE',  ( -2.298097038856279362, 1.874999999999999778, -5.798097038856278473 ) ) ;
#2078=CARTESIAN_POINT ( 'NONE',  ( 2.651650429449553314, 10.37500000000000000, -0.8483495705504476847 ) ) ;
#2079=CARTESIAN_POINT ( 'NONE',  ( 1.553300858899108849, 14.93750000000000178, 0.2499999999999993616 ) ) ;
#2082=CARTESIAN_POINT ( 'NONE',  ( 1.553300858899105963, 14.06250000000000178, -7.250000000000000888 ) ) ;
#2091=CARTESIAN_POINT ( 'NONE',  ( -2.298097038856279362, 0.8750000000000000000, -5.798097038856278473 ) ) ;
#2094=AXIS2_PLACEMENT_3D ( 'NONE', #9344, #15087, #13922 ) ;
#2100=CARTESIAN_POINT ( 'NONE',  ( 1.346194077712561166, 13.43750000000000355, -0.2500000000000011102 ) ) ;
#2102=CARTESIAN_POINT ( 'NONE',  ( 2.651650429449554203, 1.375000000000000000, -0.8483495705504471296 ) ) ;
#2104=CARTESIAN_POINT ( 'NONE',  ( -0.3766621274091715432, -0.2054769798019681903, -0.1347136637304948981 ) ) ;
#2106=CARTESIAN_POINT ( 'NONE',  ( 2.298097038856278473, 14.62500000000000000, -5.798097038856279362 ) ) ;
#2109=CARTESIAN_POINT ( 'NONE',  ( 2.298097038856279362, 9.875000000000000000, -1.201902961143720860 ) ) ;
#2112=VERTEX_POINT ( 'NONE', #11812 ) ;
#2115=CARTESIAN_POINT ( 'NONE',  ( -3.749999999999999556, 14.75000000000000000, -3.499999999999999112 ) ) ;
#2116=CARTESIAN_POINT ( 'NONE',  ( 2.298097038856279362, 15.37500000000000178, -1.201902961143720860 ) ) ;
#2119=CARTESIAN_POINT ( 'NONE',  ( -3.249999999999999556, 7.187500000000000000, -2.153805922287440833 ) ) ;
#2120=CARTESIAN_POINT ( 'NONE',  ( -1.346194077712559167, 0.9375000000000000000, -6.749999999999999112 ) ) ;
#2121=ADVANCED_FACE ( 'NONE', ( #10515, #14075 ), #15247, .F. ) ;
#2125=CARTESIAN_POINT ( 'NONE',  ( -1.346194077712559389, 5.062500000000001776, -0.2500000000000002220 ) ) ;
#2131=CARTESIAN_POINT ( 'NONE',  ( 3.249999999999999556, 10.75000000000000000, -3.500000000000000000 ) ) ;
#2134=CARTESIAN_POINT ( 'NONE',  ( 2.651650429449554203, 11.37500000000000000, -0.8483495705504471296 ) ) ;
#2136=CARTESIAN_POINT ( 'NONE',  ( -2.651650429449552870, 0.6250000000000002220, -0.8483495705504463524 ) ) ;
#2137=CARTESIAN_POINT ( 'NONE',  ( -3.249999999999999112, 6.812500000000001776, -4.846194077712558723 ) ) ;
#2138=EDGE_LOOP ( 'NONE', ( #1727, #4975, #10021, #10676 ) ) ;
#2141=CARTESIAN_POINT ( 'NONE',  ( 2.298097038856279362, 1.875000000000000000, -1.201902961143720860 ) ) ;
#2143=CARTESIAN_POINT ( 'NONE',  ( 2.651650429449552870, 6.625000000000000000, -6.151650429449554203 ) ) ;
#2151=CARTESIAN_POINT ( 'NONE',  ( 0.000000000000000000, 8.500000000000000000, -0.2500000000000002220 ) ) ;
#2155=CARTESIAN_POINT ( 'NONE',  ( -1.553300858899107073, 7.937500000000001776, -7.249999999999999112 ) ) ;
#2161=CARTESIAN_POINT ( 'NONE',  ( 3.749999999999999556, 13.25000000000000000, -3.500000000000000444 ) ) ;
#2167=CARTESIAN_POINT ( 'NONE',  ( -1.346194077712558945, 4.062500000000000000, -0.2500000000000002220 ) ) ;
#2169=CARTESIAN_POINT ( 'NONE',  ( -3.249999999999999112, 1.812499999999999778, -4.846194077712558723 ) ) ;
#2174=CARTESIAN_POINT ( 'NONE',  ( -2.298097038856278029, 12.62500000000000000, -1.201902961143720638 ) ) ;
#2176=CARTESIAN_POINT ( 'NONE',  ( 1.553300858899109516, 2.437500000000000444, 0.2499999999999993616 ) ) ;
#2181=CARTESIAN_POINT ( 'NONE',  ( 2.298097038856278473, 6.625000000000000000, -5.798097038856279362 ) ) ;
#2187=CARTESIAN_POINT ( 'NONE',  ( 0.000000000000000000, 7.000000000000000000, 0.2500000000000002220 ) ) ;
#2188=CARTESIAN_POINT ( 'NONE',  ( -1.553300858899107073, 0.9375000000000000000, -7.249999999999999112 ) ) ;
#2191=CARTESIAN_POINT ( 'NONE',  ( 3.249999999999998224, 2.312500000000000000, -2.153805922287439945 ) ) ;
#2193=CARTESIAN_POINT ( 'NONE',  ( 1.346194077712560944, 5.937500000000000000, -0.2500000000000010547 ) ) ;
#2197=EDGE_CURVE ( 'NONE', #6060, #2112, #9479, .T. ) ;
#2200=CARTESIAN_POINT ( 'NONE',  ( 2.298097038856278473, 11.62500000000000000, -5.798097038856279362 ) ) ;
#2201=ORIENTED_EDGE ( 'NONE', *, *, #6737, .F. ) ;
#2203=CARTESIAN_POINT ( 'NONE',  ( -1.553300858899106629, 11.56250000000000178, 0.2500000000000002220 ) ) ;
#2205=CARTESIAN_POINT ( 'NONE',  ( 0.000000000000000000, 6.500000000000000000, 0.2500000000000002220 ) ) ;
#2206=CARTESIAN_POINT ( 'NONE',  ( -3.249999999999999112, 4.812500000000001776, -4.846194077712558723 ) ) ;
#2209=CARTESIAN_POINT ( 'NONE',  ( -3.249999999999999556, 1.312500000000000444, -4.846194077712557835 ) ) ;
#2210=CARTESIAN_POINT ( 'NONE',  ( 3.749999999999998668, 7.687500000000000000, -5.053300858899107517 ) ) ;
#2221=CARTESIAN_POINT ( 'NONE',  ( -1.346194077712559167, 7.937500000000001776, -6.749999999999999112 ) ) ;
#2223=CARTESIAN_POINT ( 'NONE',  ( -4.592425496802573972E-16, 8.000000000000000000, -7.250000000000000000 ) ) ;
#2224=CARTESIAN_POINT ( 'NONE',  ( 3.750000000000000000, 12.75000000000000178, -3.500000000000000444 ) ) ;
#2225=CARTESIAN_POINT ( 'NONE',  ( 3.249999999999999556, 11.75000000000000000, -3.500000000000000000 ) ) ;
#2226=CARTESIAN_POINT ( 'NONE',  ( 3.249999999999999556, 1.750000000000000000, -3.500000000000000000 ) ) ;
#2229=CARTESIAN_POINT ( 'NONE',  ( -3.249999999999999556, 8.250000000000000000, -3.499999999999999556 ) ) ;
#2230=CARTESIAN_POINT ( 'NONE',  ( 0.000000000000000000, -0.4999999999999999445, -0.2500000000000002220 ) ) ;
#2238=CARTESIAN_POINT ( 'NONE',  ( -2.298097038856278473, 2.125000000000000000, -1.201902961143720416 ) ) ;
#2243=CARTESIAN_POINT ( 'NONE',  ( 3.249999999999998224, 3.312500000000000000, -2.153805922287439945 ) ) ;
#2251=CARTESIAN_POINT ( 'NONE',  ( 2.298097038856279362, 13.37500000000000000, -1.201902961143720860 ) ) ;
#2253=CARTESIAN_POINT ( 'NONE',  ( 1.553300858899105963, 1.062500000000000444, -7.250000000000000888 ) ) ;
#2255=CARTESIAN_POINT ( 'NONE',  ( -0.3766621274094114624, -0.2521619801956713203, -0.04364880428836830084 ) ) ;
#2260=CARTESIAN_POINT ( 'NONE',  ( -1.346194077712559389, 14.43750000000000000, -6.749999999999999112 ) ) ;
#2261=ADVANCED_FACE ( 'NONE', ( #2944 ), #9667, .F. ) ;
#2262=CARTESIAN_POINT ( 'NONE',  ( 0.3766621274091715987, -0.2500000000000000000, -6.863050255469941519 ) ) ;
#2267=CARTESIAN_POINT ( 'NONE',  ( 3.749999999999998668, 3.687500000000000444, -5.053300858899107517 ) ) ;
#2268=CARTESIAN_POINT ( 'NONE',  ( 3.749999999999998668, 5.187499999999999112, -5.053300858899108405 ) ) ;
#2272=CARTESIAN_POINT ( 'NONE',  ( 3.249999999999998224, 1.187499999999999778, -4.846194077712561388 ) ) ;
#2276=CARTESIAN_POINT ( 'NONE',  ( -3.249999999999999556, 5.250000000000000000, -3.499999999999999556 ) ) ;
#2282=CARTESIAN_POINT ( 'NONE',  ( 3.249999999999999556, 9.750000000000000000, -3.500000000000000000 ) ) ;
#2285=CARTESIAN_POINT ( 'NONE',  ( 3.749999999999999556, 10.25000000000000178, -3.500000000000000444 ) ) ;
#2287=CARTESIAN_POINT ( 'NONE',  ( -2.651650429449553314, 3.875000000000000444, -6.151650429449552426 ) ) ;
#2288=CARTESIAN_POINT ( 'NONE',  ( 0.000000000000000000, 6.500000000000000000, -0.2500000000000002220 ) ) ;
#2290=B_SPLINE_CURVE_WITH_KNOTS ( 'NONE', 3,
 ( #1474, #6190, #2640, #7344 ),
 .UNSPECIFIED., .F., .F.,
 ( 4, 4 ),
 ( 0.000000000000000000, 0.0003021952495015066973 ),
 .UNSPECIFIED. ) ;
#2292=CARTESIAN_POINT ( 'NONE',  ( 3.249999999999999112, 3.812500000000000000, -2.153805922287439945 ) ) ;
#2293=CARTESIAN_POINT ( 'NONE',  ( -2.651650429449552870, 8.125000000000000000, -0.8483495705504462414 ) ) ;
#2301=CARTESIAN_POINT ( 'NONE',  ( 0.000000000000000000, 5.500000000000000000, -0.2500000000000002220 ) ) ;
#2305=CARTESIAN_POINT ( 'NONE',  ( -1.553300858899106629, 7.562500000000000888, 0.2499999999999998335 ) ) ;
#2306=CARTESIAN_POINT ( 'NONE',  ( -1.553300858899107073, 14.43750000000000000, -7.250000000000000000 ) ) ;
#2310=CARTESIAN_POINT ( 'NONE',  ( 1.346194077712558279, 0.06250000000000016653, -6.750000000000000888 ) ) ;
#2319=CARTESIAN_POINT ( 'NONE',  ( 1.346194077712560944, 2.937500000000000000, -0.2500000000000011102 ) ) ;
#2322=CARTESIAN_POINT ( 'NONE',  ( 0.000000000000000000, 8.500000000000000000, -0.2500000000000002220 ) ) ;
#2327=CARTESIAN_POINT ( 'NONE',  ( 0.000000000000000000, 1.000000000000000000, -0.2500000000000002220 ) ) ;
#2329=CARTESIAN_POINT ( 'NONE',  ( -2.298097038856279362, 11.87500000000000000, -5.798097038856278473 ) ) ;
#2332=CARTESIAN_POINT ( 'NONE',  ( -3.749999999999999556, 2.750000000000000444, -3.499999999999999112 ) ) ;
#2337=CARTESIAN_POINT ( 'NONE',  ( 2.298097038856278473, 12.62500000000000000, -5.798097038856279362 ) ) ;
#2344=CARTESIAN_POINT ( 'NONE',  ( 2.651650429449552870, 5.625000000000000000, -6.151650429449554203 ) ) ;
#2345=CARTESIAN_POINT ( 'NONE',  ( -2.651650429449552870, 3.625000000000000888, -0.8483495705504467965 ) ) ;
#2348=CARTESIAN_POINT ( 'NONE',  ( -3.249999999999999112, 1.812499999999999778, -4.846194077712558723 ) ) ;
#2352=CARTESIAN_POINT ( 'NONE',  ( -2.298097038856278918, 3.375000000000000000, -5.798097038856277585 ) ) ;
#2362=CARTESIAN_POINT ( 'NONE',  ( -3.750000000000000000, 7.812500000000000000, -5.053300858899105741 ) ) ;
#2363=CARTESIAN_POINT ( 'NONE',  ( 1.346194077712561166, 8.437500000000000000, -0.2500000000000011102 ) ) ;
#2366=CARTESIAN_POINT ( 'NONE',  ( -2.298097038856278473, 3.125000000000000000, -1.201902961143720416 ) ) ;
#2367=CARTESIAN_POINT ( 'NONE',  ( 2.651650429449552870, 10.62500000000000000, -6.151650429449554203 ) ) ;
#2375=CARTESIAN_POINT ( 'NONE',  ( -1.553300858899107073, 12.93750000000000178, -7.249999999999999112 ) ) ;
#2379=CARTESIAN_POINT ( 'NONE',  ( -2.298097038856278029, 0.6250000000000002220, -1.201902961143720638 ) ) ;
#2387=CARTESIAN_POINT ( 'NONE',  ( -2.298097038856278918, 2.375000000000000000, -5.798097038856277585 ) ) ;
#2389=CARTESIAN_POINT ( 'NONE',  ( 0.000000000000000000, 6.500000000000000000, -0.2500000000000002220 ) ) ;
#2393=CARTESIAN_POINT ( 'NONE',  ( -0.3766621274091715987, 0.5000000000000000000, -7.146945437571387671 ) ) ;
#2395=CARTESIAN_POINT ( 'NONE',  ( -3.249999999999999556, 1.250000000000000000, -3.499999999999999556 ) ) ;
#2396=CARTESIAN_POINT ( 'NONE',  ( 3.749999999999998668, 1.187499999999999778, -5.053300858899108405 ) ) ;
#2397=CARTESIAN_POINT ( 'NONE',  ( 2.651650429449552870, 3.625000000000000000, -6.151650429449554203 ) ) ;
#2399=CARTESIAN_POINT ( 'NONE',  ( -1.553300858899107073, 0.9375000000000002220, -7.249999999999999112 ) ) ;
#2404=CARTESIAN_POINT ( 'NONE',  ( 0.000000000000000000, 12.00000000000000000, -0.2500000000000002220 ) ) ;
#2412=CARTESIAN_POINT ( 'NONE',  ( 3.749999999999998668, 5.687500000000000000, -5.053300858899107517 ) ) ;
#2413=CARTESIAN_POINT ( 'NONE',  ( 1.553300858899105963, 4.062500000000001776, -7.249999999999999112 ) ) ;
#2416=CARTESIAN_POINT ( 'NONE',  ( 3.249999999999999556, 14.75000000000000178, -3.500000000000000000 ) ) ;
#2419=( NAMED_UNIT ( * ) SI_UNIT ( $, .STERADIAN. ) SOLID_ANGLE_UNIT ( ) );
#2420=CARTESIAN_POINT ( 'NONE',  ( 3.249999999999999112, 5.812500000000000000, -2.153805922287439945 ) ) ;
#2432=CARTESIAN_POINT ( 'NONE',  ( 2.651650429449552870, 4.125000000000000000, -6.151650429449555091 ) ) ;
#2434=CARTESIAN_POINT ( 'NONE',  ( -2.298097038856279362, 4.875000000000000000, -5.798097038856278473 ) ) ;
#2438=CARTESIAN_POINT ( 'NONE',  ( 3.249999999999998668, 4.687500000000000888, -4.846194077712560500 ) ) ;
#2446=CARTESIAN_POINT ( 'NONE',  ( 0.3766621274091715987, 0.5000000000000000000, -6.863050255469941519 ) ) ;
#2450=CARTESIAN_POINT ( 'NONE',  ( -1.553300858899106629, 13.56250000000000000, 0.2499999999999998335 ) ) ;
#2454=CARTESIAN_POINT ( 'NONE',  ( 3.249999999999998224, 4.312500000000000000, -2.153805922287439945 ) ) ;
#2458=CARTESIAN_POINT ( 'NONE',  ( 1.346194077712558057, 14.56250000000000000, -6.750000000000000000 ) ) ;
#2463=CARTESIAN_POINT ( 'NONE',  ( -3.249999999999999556, 1.187500000000000000, -2.153805922287440833 ) ) ;
#2465=CARTESIAN_POINT ( 'NONE',  ( -1.346194077712559167, 4.937500000000000888, -6.749999999999999112 ) ) ;
#2472=CARTESIAN_POINT ( 'NONE',  ( -3.249999999999999556, 1.187500000000000444, -2.153805922287440833 ) ) ;
#2473=CARTESIAN_POINT ( 'NONE',  ( -3.750000000000000000, 2.687500000000000888, -1.946699141100893149 ) ) ;
#2475=CARTESIAN_POINT ( 'NONE',  ( 3.750000000000000000, 6.750000000000000000, -3.500000000000000444 ) ) ;
#2477=CARTESIAN_POINT ( 'NONE',  ( -2.651650429449552870, 6.625000000000000888, -0.8483495705504463524 ) ) ;
#2483=CARTESIAN_POINT ( 'NONE',  ( 3.249999999999999556, 13.75000000000000000, -3.500000000000000000 ) ) ;
#2492=CARTESIAN_POINT ( 'NONE',  ( 3.749999999999999112, 6.812500000000000000, -1.946699141100892039 ) ) ;
#2493=CARTESIAN_POINT ( 'NONE',  ( 1.553300858899109071, 2.437500000000000444, 0.2499999999999989175 ) ) ;
#2497=CARTESIAN_POINT ( 'NONE',  ( -1.346194077712558945, 3.562500000000000888, -0.2500000000000002220 ) ) ;
#2502=EDGE_CURVE ( 'NONE', #6131, #13895, #14758, .T. ) ;
#2503=CARTESIAN_POINT ( 'NONE',  ( 1.346194077712558057, 6.562500000000000000, -6.750000000000000000 ) ) ;
#2515=CARTESIAN_POINT ( 'NONE',  ( -3.750000000000000000, 5.812500000000000888, -5.053300858899105741 ) ) ;
#2517=CARTESIAN_POINT ( 'NONE',  ( 2.298097038856279362, 9.374999999999998224, -1.201902961143720860 ) ) ;
#2520=CARTESIAN_POINT ( 'NONE',  ( -1.346194077712559389, 8.437500000000000000, -6.749999999999999112 ) ) ;
#2528=ORIENTED_EDGE ( 'NONE', *, *, #2502, .F. ) ;
#2531=CARTESIAN_POINT ( 'NONE',  ( 2.651650429449553314, 13.37500000000000000, -0.8483495705504476847 ) ) ;
#2536=CARTESIAN_POINT ( 'NONE',  ( -1.346194077712559167, 1.937500000000000222, -6.749999999999999112 ) ) ;
#2540=CARTESIAN_POINT ( 'NONE',  ( 1.346194077712560944, 14.93750000000000178, -0.2500000000000010547 ) ) ;
#2544=CARTESIAN_POINT ( 'NONE',  ( -1.346194077712558945, 6.062500000000000000, -0.2500000000000002220 ) ) ;
#2547=CARTESIAN_POINT ( 'NONE',  ( -2.298097038856279362, 0.8750000000000000000, -5.798097038856278473 ) ) ;
#2548=CARTESIAN_POINT ( 'NONE',  ( 3.249999999999999556, 6.250000000000000888, -3.500000000000000000 ) ) ;
#2553=CARTESIAN_POINT ( 'NONE',  ( 1.346194077712558057, 2.562500000000000444, -6.750000000000000000 ) ) ;
#2554=CARTESIAN_POINT ( 'NONE',  ( -2.651650429449552870, 1.874999999999999778, -6.151650429449552426 ) ) ;
#2555=CARTESIAN_POINT ( 'NONE',  ( -1.553300858899107073, 7.437500000000000888, -7.250000000000000000 ) ) ;
#2557=CARTESIAN_POINT ( 'NONE',  ( 2.651650429449554203, 5.375000000000000888, -0.8483495705504471296 ) ) ;
#2564=CARTESIAN_POINT ( 'NONE',  ( -2.298097038856278918, 12.37500000000000000, -5.798097038856277585 ) ) ;
#2568=CARTESIAN_POINT ( 'NONE',  ( -3.750000000000000000, 9.687500000000000000, -1.946699141100893149 ) ) ;
#2572=CARTESIAN_POINT ( 'NONE',  ( 2.651650429449553759, 8.875000000000001776, -0.8483495705504471296 ) ) ;
#2574=CARTESIAN_POINT ( 'NONE',  ( 3.749999999999998668, 3.187500000000000444, -5.053300858899108405 ) ) ;
#2575=AXIS2_PLACEMENT_3D ( 'NONE', #9445, #1105, #7107 ) ;
#2577=ORIENTED_EDGE ( 'NONE', *, *, #5243, .T. ) ;
#2578=CARTESIAN_POINT ( 'NONE',  ( -3.249999999999999112, 2.812500000000000444, -4.846194077712558723 ) ) ;
#2581=CARTESIAN_POINT ( 'NONE',  ( 1.346194077712560944, 6.937500000000000000, -0.2500000000000010547 ) ) ;
#2591=CARTESIAN_POINT ( 'NONE',  ( 3.749999999999999112, 14.31250000000000355, -1.946699141100893149 ) ) ;
#2592=CARTESIAN_POINT ( 'NONE',  ( 3.249999999999999556, 8.250000000000000000, -3.500000000000000000 ) ) ;
#2593=CARTESIAN_POINT ( 'NONE',  ( 3.249999999999998224, 10.18750000000000533, -4.846194077712561388 ) ) ;
#2598=CARTESIAN_POINT ( 'NONE',  ( 2.298097038856279362, 6.875000000000000000, -1.201902961143720860 ) ) ;
#2605=CARTESIAN_POINT ( 'NONE',  ( 3.249999999999998224, 13.31250000000000178, -2.153805922287439945 ) ) ;
#2609=CARTESIAN_POINT ( 'NONE',  ( 3.749999999999998668, 15.18750000000000355, -5.053300858899108405 ) ) ;
#2612=CARTESIAN_POINT ( 'NONE',  ( 2.298097038856279362, 2.375000000000000000, -1.201902961143720860 ) ) ;
#2619=CARTESIAN_POINT ( 'NONE',  ( 2.298097038856279362, 8.875000000000001776, -1.201902961143720860 ) ) ;
#2621=CARTESIAN_POINT ( 'NONE',  ( -1.346194077712559389, 13.06250000000000000, -0.2500000000000002220 ) ) ;
#2623=CARTESIAN_POINT ( 'NONE',  ( 1.346194077712561166, 8.437500000000000000, -0.2500000000000011102 ) ) ;
#2627=EDGE_CURVE ( 'NONE', #3762, #11999, #7419, .T. ) ;
#2630=CARTESIAN_POINT ( 'NONE',  ( 1.553300858899105963, 3.062500000000000000, -7.249999999999999112 ) ) ;
#2631=CARTESIAN_POINT ( 'NONE',  ( 0.000000000000000000, 5.000000000000000000, 0.2500000000000002220 ) ) ;
#2633=CARTESIAN_POINT ( 'NONE',  ( -1.553300858899106629, 7.562500000000000888, 0.2500000000000002220 ) ) ;
#2640=CARTESIAN_POINT ( 'NONE',  ( 0.3766621274094206773, 0.2481712481078264254, -6.953504530381456661 ) ) ;
#2644=CARTESIAN_POINT ( 'NONE',  ( 3.749999999999999556, 11.25000000000000000, -3.500000000000000444 ) ) ;
#2648=CARTESIAN_POINT ( 'NONE',  ( -3.749999999999999556, 7.312500000000000888, -5.053300858899104853 ) ) ;
#2649=CARTESIAN_POINT ( 'NONE',  ( 3.749999999999999556, 6.250000000000000000, -3.500000000000000444 ) ) ;
#2653=CARTESIAN_POINT ( 'NONE',  ( -3.249999999999999112, 5.812500000000000888, -4.846194077712558723 ) ) ;
#2655=CARTESIAN_POINT ( 'NONE',  ( -3.749999999999999556, 11.18749999999999822, -1.946699141100892927 ) ) ;
#2659=CARTESIAN_POINT ( 'NONE',  ( 2.298097038856279362, 8.875000000000001776, -1.201902961143720860 ) ) ;
#2669=CARTESIAN_POINT ( 'NONE',  ( -3.750000000000000000, 12.81250000000000178, -5.053300858899105741 ) ) ;
#2670=CARTESIAN_POINT ( 'NONE',  ( -1.346194077712558945, 10.56250000000000355, -0.2500000000000002220 ) ) ;
#2671=CARTESIAN_POINT ( 'NONE',  ( 3.249999999999998224, 9.312500000000000000, -2.153805922287439945 ) ) ;
#2674=CARTESIAN_POINT ( 'NONE',  ( 3.249999999999999556, 6.750000000000000000, -3.500000000000000000 ) ) ;
#2682=CARTESIAN_POINT ( 'NONE',  ( -2.298097038856278473, 1.125000000000000222, -1.201902961143720416 ) ) ;
#2683=CARTESIAN_POINT ( 'NONE',  ( -3.749999999999999556, 14.31250000000000000, -5.053300858899104853 ) ) ;
#2685=CARTESIAN_POINT ( 'NONE',  ( -3.750000000000000000, 13.81250000000000178, -5.053300858899105741 ) ) ;
#2689=CARTESIAN_POINT ( 'NONE',  ( -3.249999999999999556, 2.750000000000000444, -3.500000000000000000 ) ) ;
#2697=CARTESIAN_POINT ( 'NONE',  ( -3.980102097228897245E-16, 5.500000000000000000, -6.749999999999999112 ) ) ;
#2699=CARTESIAN_POINT ( 'NONE',  ( 2.298097038856279362, 11.87500000000000000, -1.201902961143720860 ) ) ;
#2700=CARTESIAN_POINT ( 'NONE',  ( -1.346194077712559167, 9.937500000000001776, -6.749999999999999112 ) ) ;
#2704=CARTESIAN_POINT ( 'NONE',  ( 1.346194077712558057, 5.562500000000000000, -6.750000000000000000 ) ) ;
#2705=CARTESIAN_POINT ( 'NONE',  ( 1.346194077712561166, 15.43750000000000178, -0.2500000000000011102 ) ) ;
#2706=CARTESIAN_POINT ( 'NONE',  ( -2.651650429449552870, 7.125000000000000000, -0.8483495705504462414 ) ) ;
#2708=CARTESIAN_POINT ( 'NONE',  ( -2.651650429449553314, 5.875000000000001776, -6.151650429449552426 ) ) ;
#2714=EDGE_CURVE ( 'NONE', #13895, #5120, #1998, .T. ) ;
#2720=CARTESIAN_POINT ( 'NONE',  ( 3.749999999999999112, 12.18750000000000178, -5.053300858899108405 ) ) ;
#2724=CARTESIAN_POINT ( 'NONE',  ( 3.750000000000000000, 8.750000000000000000, -3.500000000000000444 ) ) ;
#2725=CARTESIAN_POINT ( 'NONE',  ( -3.750000000000000000, 7.812500000000000000, -5.053300858899105741 ) ) ;
#2728=EDGE_LOOP ( 'NONE', ( #13599, #1224, #3776 ) ) ;
#2729=CARTESIAN_POINT ( 'NONE',  ( -3.980102097228897738E-16, 5.999999999999999112, -6.749999999999999112 ) ) ;
#2730=CARTESIAN_POINT ( 'NONE',  ( 3.750000000000000000, 8.750000000000000000, -3.500000000000000444 ) ) ;
#2735=CARTESIAN_POINT ( 'NONE',  ( 3.249999999999999112, 6.812500000000000000, -2.153805922287439945 ) ) ;
#2749=CARTESIAN_POINT ( 'NONE',  ( -1.553300858899107073, 13.93750000000000000, -7.249999999999999112 ) ) ;
#2750=CARTESIAN_POINT ( 'NONE',  ( 1.346194077712561166, 10.43750000000000178, -0.2500000000000011102 ) ) ;
#2751=CARTESIAN_POINT ( 'NONE',  ( -3.249999999999999112, 9.687500000000000000, -2.153805922287440833 ) ) ;
#2756=CARTESIAN_POINT ( 'NONE',  ( -3.249999999999999556, 8.250000000000000000, -3.499999999999999556 ) ) ;
#2763=ORIENTED_EDGE ( 'NONE', *, *, #7781, .F. ) ;
#2764=CARTESIAN_POINT ( 'NONE',  ( 3.249999999999998668, 0.6875000000000000000, -4.846194077712560500 ) ) ;
#2765=CARTESIAN_POINT ( 'NONE',  ( -2.651650429449553314, 12.37500000000000000, -6.151650429449552426 ) ) ;
#2768=CARTESIAN_POINT ( 'NONE',  ( -4.592425496802573972E-16, 0.5000000000000000000, -7.249999999999999112 ) ) ;
#2776=VERTEX_POINT ( 'NONE', #9925 ) ;
#2778=CARTESIAN_POINT ( 'NONE',  ( 2.298097038856278473, 7.625000000000000000, -5.798097038856279362 ) ) ;
#2780=CARTESIAN_POINT ( 'NONE',  ( -3.980102097228897245E-16, 12.50000000000000000, -6.749999999999999112 ) ) ;
#2782=CARTESIAN_POINT ( 'NONE',  ( 3.249999999999998224, 10.18750000000000533, -4.846194077712561388 ) ) ;
#2787=CARTESIAN_POINT ( 'NONE',  ( -3.249999999999999556, 4.312500000000000888, -4.846194077712557835 ) ) ;
#2788=CARTESIAN_POINT ( 'NONE',  ( -3.750000000000000000, 4.687500000000000000, -1.946699141100893149 ) ) ;
#2789=CARTESIAN_POINT ( 'NONE',  ( 3.750000000000000000, 10.75000000000000000, -3.500000000000000444 ) ) ;
#2791=CARTESIAN_POINT ( 'NONE',  ( -4.592425496802573972E-16, 7.000000000000000000, -7.250000000000000000 ) ) ;
#2800=CARTESIAN_POINT ( 'NONE',  ( 1.553300858899105963, 14.06250000000000178, -7.250000000000000888 ) ) ;
#2804=CARTESIAN_POINT ( 'NONE',  ( -1.553300858899106629, 8.062500000000000000, 0.2500000000000002220 ) ) ;
#2805=CARTESIAN_POINT ( 'NONE',  ( 3.749999999999998668, 7.187500000000000888, -5.053300858899108405 ) ) ;
#2808=EDGE_CURVE ( 'NONE', #5961, #12717, #5292, .T. ) ;
#2810=ADVANCED_BREP_SHAPE_REPRESENTATION ( '', ( #7115, #9419 ), #6710 ) ;
#2811=CARTESIAN_POINT ( 'NONE',  ( -1.346194077712558945, 4.562500000000000000, -0.2500000000000002220 ) ) ;
#2813=CARTESIAN_POINT ( 'NONE',  ( -4.592425496802573972E-16, 9.500000000000000000, -7.249999999999999112 ) ) ;
#2817=CARTESIAN_POINT ( 'NONE',  ( -2.298097038856278918, 9.375000000000000000, -5.798097038856277585 ) ) ;
#2827=DIRECTION ( 'NONE',  ( 0.000000000000000000, 0.000000000000000000, -1.000000000000000000 ) ) ;
#2830=CARTESIAN_POINT ( 'NONE',  ( -2.651650429449552870, 13.87500000000000178, -6.151650429449552426 ) ) ;
#2831=CARTESIAN_POINT ( 'NONE',  ( 2.298097038856278029, 13.12500000000000178, -5.798097038856279362 ) ) ;
#2832=CARTESIAN_POINT ( 'NONE',  ( 1.346194077712561166, 10.43750000000000178, -0.2500000000000011102 ) ) ;
#2835=CARTESIAN_POINT ( 'NONE',  ( 1.346194077712558057, 8.562500000000001776, -6.750000000000000000 ) ) ;
#2837=VECTOR ( 'NONE', #4354, 1000.000000000000000 ) ;
#2845=CARTESIAN_POINT ( 'NONE',  ( -1.346194077712559389, 2.062500000000000000, -0.2500000000000002220 ) ) ;
#2847=CARTESIAN_POINT ( 'NONE',  ( -2.651650429449552870, 14.12500000000000000, -0.8483495705504462414 ) ) ;
#2850=CARTESIAN_POINT ( 'NONE',  ( -3.749999999999999556, 0.3125000000000000555, -5.053300858899104853 ) ) ;
#2853=CARTESIAN_POINT ( 'NONE',  ( -2.651650429449553314, 0.3750000000000000555, -6.151650429449552426 ) ) ;
#2857=ORIENTED_EDGE ( 'NONE', *, *, #8813, .F. ) ;
#2858=CARTESIAN_POINT ( 'NONE',  ( 3.249999999999998668, 8.687500000000000000, -4.846194077712560500 ) ) ;
#2860=CARTESIAN_POINT ( 'NONE',  ( 1.346194077712560944, 14.93750000000000178, -0.2500000000000010547 ) ) ;
#2861=CARTESIAN_POINT ( 'NONE',  ( -1.346194077712559167, 8.937500000000000000, -6.749999999999999112 ) ) ;
#2865=CARTESIAN_POINT ( 'NONE',  ( 1.346194077712558057, 6.562500000000000000, -6.750000000000000000 ) ) ;
#2866=CARTESIAN_POINT ( 'NONE',  ( -2.651650429449552870, 4.875000000000000000, -6.151650429449552426 ) ) ;
#2867=CARTESIAN_POINT ( 'NONE',  ( -2.651650429449552870, 10.12500000000000000, -0.8483495705504462414 ) ) ;
#2870=CARTESIAN_POINT ( 'NONE',  ( 1.553300858899109516, 11.43750000000000178, 0.2499999999999993616 ) ) ;
#2875=CARTESIAN_POINT ( 'NONE',  ( -0.3766621274091713767, 0.2975415354274087432, -7.146945437571386783 ) ) ;
#2877=CARTESIAN_POINT ( 'NONE',  ( 1.346194077712558279, 0.06250000000000016653, -6.750000000000000888 ) ) ;
#2880=CARTESIAN_POINT ( 'NONE',  ( 2.651650429449552870, 7.625000000000000000, -6.151650429449554203 ) ) ;
#2881=CARTESIAN_POINT ( 'NONE',  ( 1.553300858899105963, 10.06250000000000000, -7.249999999999999112 ) ) ;
#2884=CARTESIAN_POINT ( 'NONE',  ( -3.249999999999999112, 7.812500000000000000, -4.846194077712558723 ) ) ;
#2885=CARTESIAN_POINT ( 'NONE',  ( -3.750000000000000000, 13.25000000000000000, -3.499999999999999112 ) ) ;
#2889=CARTESIAN_POINT ( 'NONE',  ( 1.346194077712558057, 10.56250000000000000, -6.750000000000000000 ) ) ;
#2899=CARTESIAN_POINT ( 'NONE',  ( -2.651650429449552870, 13.62500000000000000, -0.8483495705504467965 ) ) ;
#2900=CARTESIAN_POINT ( 'NONE',  ( -3.249999999999999112, 10.68750000000000178, -2.153805922287440833 ) ) ;
#2901=CARTESIAN_POINT ( 'NONE',  ( -2.298097038856279362, 12.87500000000000000, -5.798097038856278473 ) ) ;
#2903=CARTESIAN_POINT ( 'NONE',  ( -3.249999999999999556, 9.187500000000000000, -2.153805922287440833 ) ) ;
#2915=CARTESIAN_POINT ( 'NONE',  ( -2.298097038856278029, 13.62500000000000000, -1.201902961143720638 ) ) ;
#2916=CARTESIAN_POINT ( 'NONE',  ( -1.553300858899106629, 14.06249999999999822, 0.2500000000000002220 ) ) ;
#2919=CARTESIAN_POINT ( 'NONE',  ( -4.592425496802573972E-16, 1.500000000000000000, -7.249999999999999112 ) ) ;
#2922=CARTESIAN_POINT ( 'NONE',  ( -3.750000000000000000, 1.187500000000000000, -1.946699141100892927 ) ) ;
#2927=CARTESIAN_POINT ( 'NONE',  ( 1.346194077712560944, 9.937499999999998224, -0.2500000000000011102 ) ) ;
#2929=DIRECTION ( 'NONE',  ( -1.000000000000000000, 0.000000000000000000, -0.000000000000000000 ) ) ;
#2930=CARTESIAN_POINT ( 'NONE',  ( 3.249999999999998224, 2.312500000000000000, -2.153805922287439945 ) ) ;
#2931=CARTESIAN_POINT ( 'NONE',  ( 0.000000000000000000, 12.50000000000000178, -0.2500000000000002220 ) ) ;
#2934=CARTESIAN_POINT ( 'NONE',  ( 1.346194077712560944, 3.937500000000000000, -0.2500000000000010547 ) ) ;
#2935=CARTESIAN_POINT ( 'NONE',  ( 2.651650429449552870, 4.125000000000000000, -6.151650429449553314 ) ) ;
#2936=CARTESIAN_POINT ( 'NONE',  ( 1.553300858899108849, 10.93750000000000178, 0.2499999999999993616 ) ) ;
#2939=CARTESIAN_POINT ( 'NONE',  ( -3.749999999999999556, 11.75000000000000178, -3.499999999999999112 ) ) ;
#2944=FACE_OUTER_BOUND ( 'NONE', #3061, .T. ) ;
#2947=CARTESIAN_POINT ( 'NONE',  ( -2.651650429449553314, 12.87500000000000000, -6.151650429449552426 ) ) ;
#2951=CARTESIAN_POINT ( 'NONE',  ( 3.749999999999999556, 7.250000000000000000, -3.500000000000000444 ) ) ;
#2953=CARTESIAN_POINT ( 'NONE',  ( -3.249999999999999112, 6.687500000000000888, -2.153805922287440833 ) ) ;
#2955=CARTESIAN_POINT ( 'NONE',  ( -3.750000000000000000, -0.1874999999999998890, -5.053300858899105741 ) ) ;
#2958=CARTESIAN_POINT ( 'NONE',  ( -2.298097038856278918, 10.37500000000000000, -5.798097038856277585 ) ) ;
#2965=DIRECTION ( 'NONE',  ( 1.000000000000000000, 0.000000000000000000, 0.000000000000000000 ) ) ;
#2969=CARTESIAN_POINT ( 'NONE',  ( 0.000000000000000000, 2.000000000000000000, 0.2500000000000002220 ) ) ;
#2970=CARTESIAN_POINT ( 'NONE',  ( -1.346194077712558945, 9.562500000000000000, -0.2500000000000002220 ) ) ;
#2971=CARTESIAN_POINT ( 'NONE',  ( -3.980102097228897245E-16, 0.5000000000000000000, -6.749999999999999112 ) ) ;
#2975=CARTESIAN_POINT ( 'NONE',  ( -3.249999999999999556, 10.18750000000000000, -2.153805922287440833 ) ) ;
#2979=CARTESIAN_POINT ( 'NONE',  ( 3.249999999999999112, 8.812500000000000000, -2.153805922287439945 ) ) ;
#2987=CARTESIAN_POINT ( 'NONE',  ( 1.346194077712560944, 5.937500000000000000, -0.2500000000000010547 ) ) ;
#2989=CARTESIAN_POINT ( 'NONE',  ( 0.000000000000000000, 12.00000000000000000, 0.2500000000000002220 ) ) ;
#2992=VERTEX_POINT ( 'NONE', #10374 ) ;
#2994=CARTESIAN_POINT ( 'NONE',  ( 0.000000000000000000, 3.000000000000000000, 0.2500000000000002220 ) ) ;
#3007=CARTESIAN_POINT ( 'NONE',  ( -3.249999999999999556, 3.750000000000000444, -3.500000000000000000 ) ) ;
#3008=AXIS2_PLACEMENT_3D ( 'NONE', #13577, #5446, #9860 ) ;
#3009=CARTESIAN_POINT ( 'NONE',  ( 2.298097038856278029, 9.125000000000000000, -5.798097038856279362 ) ) ;
#3012=CARTESIAN_POINT ( 'NONE',  ( 2.298097038856279362, 4.875000000000000000, -1.201902961143720860 ) ) ;
#3013=CARTESIAN_POINT ( 'NONE',  ( -3.750000000000000000, 6.687500000000000888, -1.946699141100893149 ) ) ;
#3015=CARTESIAN_POINT ( 'NONE',  ( -3.750000000000000000, 8.250000000000000000, -3.499999999999999112 ) ) ;
#3018=CARTESIAN_POINT ( 'NONE',  ( 1.553300858899109516, 9.437500000000000000, 0.2499999999999993616 ) ) ;
#3024=CARTESIAN_POINT ( 'NONE',  ( 3.249999999999999112, 0.8125000000000001110, -2.153805922287439945 ) ) ;
#3026=CARTESIAN_POINT ( 'NONE',  ( -3.249999999999999556, -0.2499999999999998890, -3.500000000000000000 ) ) ;
#3032=CARTESIAN_POINT ( 'NONE',  ( 1.346194077712558279, 7.062499999999999112, -6.750000000000000888 ) ) ;
#3034=CARTESIAN_POINT ( 'NONE',  ( 3.750000000000000000, 12.75000000000000178, -3.500000000000000444 ) ) ;
#3038=CARTESIAN_POINT ( 'NONE',  ( -3.249999999999999556, 13.25000000000000000, -3.499999999999999556 ) ) ;
#3041=CARTESIAN_POINT ( 'NONE',  ( -1.346194077712559389, 7.437500000000000888, -6.749999999999999112 ) ) ;
#3047=CARTESIAN_POINT ( 'NONE',  ( 3.749999999999998668, 15.18750000000000355, -5.053300858899108405 ) ) ;
#3049=CARTESIAN_POINT ( 'NONE',  ( -3.249999999999999112, 14.81250000000000355, -4.846194077712558723 ) ) ;
#3050=CARTESIAN_POINT ( 'NONE',  ( 0.000000000000000000, 13.50000000000000178, -0.2500000000000002220 ) ) ;
#3052=CARTESIAN_POINT ( 'NONE',  ( 2.298097038856278473, 11.62500000000000000, -5.798097038856279362 ) ) ;
#3061=EDGE_LOOP ( 'NONE', ( #6055, #8446, #1976, #14980 ) ) ;
#3063=CARTESIAN_POINT ( 'NONE',  ( 3.249999999999998668, 4.687500000000000888, -4.846194077712560500 ) ) ;
#3065=CARTESIAN_POINT ( 'NONE',  ( 3.749999999999999556, 3.250000000000000000, -3.500000000000000444 ) ) ;
#3068=CARTESIAN_POINT ( 'NONE',  ( -3.750000000000000000, 0.2500000000000000555, -3.499999999999999112 ) ) ;
#3071=CARTESIAN_POINT ( 'NONE',  ( -1.553300858899107073, 0.4375000000000000555, -7.250000000000000000 ) ) ;
#3079=CARTESIAN_POINT ( 'NONE',  ( 3.249999999999998224, 3.187500000000000444, -4.846194077712561388 ) ) ;
#3082=CARTESIAN_POINT ( 'NONE',  ( -4.592425496802573972E-16, 7.000000000000000000, -7.250000000000000000 ) ) ;
#3083=CARTESIAN_POINT ( 'NONE',  ( 3.750000000000000000, 7.750000000000000000, -3.500000000000000444 ) ) ;
#3086=CARTESIAN_POINT ( 'NONE',  ( 3.749999999999999112, 9.187500000000001776, -5.053300858899108405 ) ) ;
#3097=EDGE_CURVE ( 'NONE', #4358, #11999, #6887, .T. ) ;
#3098=CARTESIAN_POINT ( 'NONE',  ( 3.249999999999998224, 2.187500000000000000, -4.846194077712561388 ) ) ;
#3103=CARTESIAN_POINT ( 'NONE',  ( -1.346194077712559389, 10.06250000000000000, -0.2500000000000002220 ) ) ;
#3106=CARTESIAN_POINT ( 'NONE',  ( -3.249999999999999112, 9.687500000000000000, -2.153805922287440833 ) ) ;
#3108=CARTESIAN_POINT ( 'NONE',  ( 1.553300858899105963, 12.56250000000000000, -7.250000000000000888 ) ) ;
#3111=CARTESIAN_POINT ( 'NONE',  ( -3.249999999999999556, 13.18749999999999822, -2.153805922287440833 ) ) ;
#3112=DIRECTION ( 'NONE',  ( 1.000000000000000000, 0.000000000000000000, 0.000000000000000000 ) ) ;
#3114=CARTESIAN_POINT ( 'NONE',  ( -3.980102097228897245E-16, 8.500000000000000000, -6.749999999999999112 ) ) ;
#3120=CARTESIAN_POINT ( 'NONE',  ( -3.749999999999999556, 0.3125000000000000555, -5.053300858899104853 ) ) ;
#3121=CARTESIAN_POINT ( 'NONE',  ( -3.750000000000000000, 1.687499999999999778, -1.946699141100893149 ) ) ;
#3122=CARTESIAN_POINT ( 'NONE',  ( -2.298097038856279362, 13.87500000000000178, -5.798097038856278473 ) ) ;
#3124=CARTESIAN_POINT ( 'NONE',  ( 1.346194077712558057, 11.56249999999999822, -6.750000000000000000 ) ) ;
#3134=CARTESIAN_POINT ( 'NONE',  ( -1.346194077712559389, 4.062500000000000000, -0.2500000000000002220 ) ) ;
#3136=CARTESIAN_POINT ( 'NONE',  ( 3.750000000000000000, 3.312500000000000000, -1.946699141100892705 ) ) ;
#3137=EDGE_LOOP ( 'NONE', ( #12523, #12066, #11392, #5379 ) ) ;
#3139=CARTESIAN_POINT ( 'NONE',  ( 0.000000000000000000, 6.000000000000000000, 0.2500000000000002220 ) ) ;
#3142=CARTESIAN_POINT ( 'NONE',  ( 1.553300858899108849, 2.937500000000000000, 0.2499999999999993616 ) ) ;
#3147=CARTESIAN_POINT ( 'NONE',  ( 2.298097038856279362, 2.375000000000000000, -1.201902961143720860 ) ) ;
#3150=CARTESIAN_POINT ( 'NONE',  ( -1.553300858899107073, 8.937500000000000000, -7.249999999999999112 ) ) ;
#3151=CARTESIAN_POINT ( 'NONE',  ( 0.000000000000000000, 12.00000000000000000, 0.2500000000000002220 ) ) ;
#3155=CARTESIAN_POINT ( 'NONE',  ( -1.346194077712559389, 8.437500000000000000, -6.749999999999999112 ) ) ;
#3156=CARTESIAN_POINT ( 'NONE',  ( -3.749999999999999556, 9.750000000000000000, -3.499999999999999112 ) ) ;
#3164=CARTESIAN_POINT ( 'NONE',  ( -3.249999999999999556, 2.750000000000000444, -3.500000000000000000 ) ) ;
#3172=CARTESIAN_POINT ( 'NONE',  ( 3.249999999999998224, 10.18750000000000533, -4.846194077712561388 ) ) ;
#3175=CARTESIAN_POINT ( 'NONE',  ( -4.592425496802573972E-16, 14.50000000000000000, -7.249999999999999112 ) ) ;
#3180=CARTESIAN_POINT ( 'NONE',  ( 1.346194077712560944, 10.93750000000000000, -0.2500000000000010547 ) ) ;
#3183=CARTESIAN_POINT ( 'NONE',  ( -3.980102097228897245E-16, 10.50000000000000000, -6.749999999999999112 ) ) ;
#3189=CARTESIAN_POINT ( 'NONE',  ( 2.651650429449552870, 1.625000000000000222, -6.151650429449554203 ) ) ;
#3190=CARTESIAN_POINT ( 'NONE',  ( 2.651650429449552870, 2.125000000000000000, -6.151650429449553314 ) ) ;
#3191=CARTESIAN_POINT ( 'NONE',  ( -3.249999999999999556, 13.75000000000000000, -3.500000000000000000 ) ) ;
#3193=CARTESIAN_POINT ( 'NONE',  ( 3.249999999999999556, 11.75000000000000000, -3.500000000000000000 ) ) ;
#3205=CARTESIAN_POINT ( 'NONE',  ( -3.249999999999999556, 11.31249999999999822, -4.846194077712557835 ) ) ;
#3207=CARTESIAN_POINT ( 'NONE',  ( 2.298097038856279362, 5.875000000000000000, -1.201902961143720860 ) ) ;
#3209=CARTESIAN_POINT ( 'NONE',  ( -3.750000000000000000, 1.812499999999999778, -5.053300858899105741 ) ) ;
#3212=CARTESIAN_POINT ( 'NONE',  ( 1.346194077712558057, 0.5625000000000001110, -6.750000000000000000 ) ) ;
#3214=CARTESIAN_POINT ( 'NONE',  ( 0.000000000000000000, 5.000000000000000000, 0.2500000000000002220 ) ) ;
#3225=CARTESIAN_POINT ( 'NONE',  ( 0.000000000000000000, 4.499999999999999112, -0.2500000000000002220 ) ) ;
#3229=CARTESIAN_POINT ( 'NONE',  ( 1.553300858899105963, 8.062500000000001776, -7.249999999999999112 ) ) ;
#3230=CARTESIAN_POINT ( 'NONE',  ( -3.750000000000000000, 14.18750000000000000, -1.946699141100892927 ) ) ;
#3234=CARTESIAN_POINT ( 'NONE',  ( 3.249999999999998224, 1.187500000000000222, -4.846194077712561388 ) ) ;
#3244=CARTESIAN_POINT ( 'NONE',  ( -1.346194077712558945, 1.562500000000000222, -0.2500000000000002220 ) ) ;
#3251=CARTESIAN_POINT ( 'NONE',  ( 0.000000000000000000, 10.50000000000000000, -0.2500000000000002220 ) ) ;
#3254=CARTESIAN_POINT ( 'NONE',  ( 2.651650429449552870, 4.125000000000000000, -6.151650429449555091 ) ) ;
#3257=CARTESIAN_POINT ( 'NONE',  ( -3.249999999999999556, 14.25000000000000000, -3.499999999999999556 ) ) ;
#3260=CARTESIAN_POINT ( 'NONE',  ( -3.249999999999999556, 8.250000000000000000, -3.499999999999999556 ) ) ;
#3268=CARTESIAN_POINT ( 'NONE',  ( 1.553300858899105963, 1.562500000000000000, -7.250000000000000888 ) ) ;
#3269=CARTESIAN_POINT ( 'NONE',  ( 2.298097038856278029, 15.12500000000000000, -5.798097038856279362 ) ) ;
#3271=CARTESIAN_POINT ( 'NONE',  ( -0.3766621274091715987, -0.2500000000000000000, -0.1347136637304948981 ) ) ;
#3273=CARTESIAN_POINT ( 'NONE',  ( -2.298097038856278473, 13.12500000000000000, -1.201902961143720416 ) ) ;
#3276=CARTESIAN_POINT ( 'NONE',  ( 1.346194077712558057, 2.562500000000000444, -6.750000000000000000 ) ) ;
#3284=CARTESIAN_POINT ( 'NONE',  ( -1.346194077712558945, 12.06250000000000000, -0.2500000000000002220 ) ) ;
#3286=EDGE_CURVE ( 'NONE', #4560, #2776, #2290, .T. ) ;
#3288=CARTESIAN_POINT ( 'NONE',  ( 0.000000000000000000, 3.000000000000000000, -0.2500000000000002220 ) ) ;
#3290=CARTESIAN_POINT ( 'NONE',  ( -4.592425496802573972E-16, 3.000000000000000444, -7.250000000000000000 ) ) ;
#3292=CARTESIAN_POINT ( 'NONE',  ( -2.298097038856278029, 5.625000000000000888, -1.201902961143720638 ) ) ;
#3297=CARTESIAN_POINT ( 'NONE',  ( -1.346194077712559389, 0.06250000000000000000, -0.2500000000000002220 ) ) ;
#3298=CARTESIAN_POINT ( 'NONE',  ( -1.553300858899106629, 4.062500000000000000, 0.2500000000000002220 ) ) ;
#3307=CARTESIAN_POINT ( 'NONE',  ( 1.346194077712561166, 5.437500000000000888, -0.2500000000000011102 ) ) ;
#3310=CARTESIAN_POINT ( 'NONE',  ( -4.592425496802573972E-16, 10.00000000000000000, -7.250000000000000000 ) ) ;
#3311=CARTESIAN_POINT ( 'NONE',  ( 1.553300858899105963, 14.56250000000000000, -7.250000000000000000 ) ) ;
#3314=CARTESIAN_POINT ( 'NONE',  ( 1.553300858899109516, 12.43750000000000000, 0.2499999999999993616 ) ) ;
#3321=CARTESIAN_POINT ( 'NONE',  ( -3.249999999999999556, 0.2500000000000000000, -3.499999999999999556 ) ) ;
#3323=CARTESIAN_POINT ( 'NONE',  ( -1.346194077712558945, 3.562500000000000888, -0.2500000000000002220 ) ) ;
#3330=CARTESIAN_POINT ( 'NONE',  ( 3.249999999999998224, 11.18750000000000178, -4.846194077712561388 ) ) ;
#3332=CARTESIAN_POINT ( 'NONE',  ( -3.750000000000000000, 2.812500000000000444, -5.053300858899105741 ) ) ;
#3338=CARTESIAN_POINT ( 'NONE',  ( 2.298097038856278473, 9.625000000000000000, -5.798097038856279362 ) ) ;
#3344=CARTESIAN_POINT ( 'NONE',  ( -2.651650429449553314, 6.375000000000000888, -6.151650429449552426 ) ) ;
#3345=CARTESIAN_POINT ( 'NONE',  ( 0.000000000000000000, 1.500000000000000222, 0.2499999999999998057 ) ) ;
#3348=CARTESIAN_POINT ( 'NONE',  ( 3.249999999999998224, 2.187500000000000000, -4.846194077712561388 ) ) ;
#3353=CARTESIAN_POINT ( 'NONE',  ( 2.298097038856279362, 3.875000000000000000, -1.201902961143720860 ) ) ;
#3359=CARTESIAN_POINT ( 'NONE',  ( 3.249999999999999556, 12.75000000000000178, -3.500000000000000000 ) ) ;
#3362=CARTESIAN_POINT ( 'NONE',  ( -1.553300858899107073, 8.937500000000000000, -7.249999999999999112 ) ) ;
#3364=CARTESIAN_POINT ( 'NONE',  ( 2.651650429449552870, 1.124999999999999778, -6.151650429449555091 ) ) ;
#3365=CARTESIAN_POINT ( 'NONE',  ( -3.249999999999999556, 7.750000000000000888, -3.500000000000000000 ) ) ;
#3368=CARTESIAN_POINT ( 'NONE',  ( 1.346194077712558057, 1.562500000000000000, -6.750000000000000000 ) ) ;
#3369=CARTESIAN_POINT ( 'NONE',  ( 1.553300858899108849, 6.937500000000000000, 0.2499999999999993616 ) ) ;
#3378=CARTESIAN_POINT ( 'NONE',  ( -3.249999999999999556, 6.750000000000000888, -3.500000000000000000 ) ) ;
#3380=CARTESIAN_POINT ( 'NONE',  ( 1.553300858899109071, 9.437500000000003553, 0.2499999999999989175 ) ) ;
#3384=CARTESIAN_POINT ( 'NONE',  ( -0.3766621274091715987, -0.1687972351630583345, 0.1491815183709511161 ) ) ;
#3385=CARTESIAN_POINT ( 'NONE',  ( 2.298097038856278029, 0.1250000000000001110, -5.798097038856279362 ) ) ;
#3393=CARTESIAN_POINT ( 'NONE',  ( -1.346194077712559167, 4.437500000000001776, -6.749999999999999112 ) ) ;
#3396=CARTESIAN_POINT ( 'NONE',  ( -3.249999999999999112, 0.8125000000000001110, -4.846194077712558723 ) ) ;
#3402=CARTESIAN_POINT ( 'NONE',  ( 2.298097038856279362, 11.37500000000000178, -1.201902961143720860 ) ) ;
#3404=CARTESIAN_POINT ( 'NONE',  ( -3.749999999999999556, 1.750000000000000222, -3.499999999999999112 ) ) ;
#3409=CARTESIAN_POINT ( 'NONE',  ( -3.249999999999999556, 12.31250000000000000, -4.846194077712557835 ) ) ;
#3415=CARTESIAN_POINT ( 'NONE',  ( -1.553300858899107295, 6.437500000000000888, -7.250000000000000000 ) ) ;
#3416=CARTESIAN_POINT ( 'NONE',  ( 2.651650429449553314, 3.375000000000000444, -0.8483495705504476847 ) ) ;
#3419=CARTESIAN_POINT ( 'NONE',  ( -1.346194077712559389, 14.06249999999999822, -0.2500000000000002220 ) ) ;
#3423=CARTESIAN_POINT ( 'NONE',  ( 2.298097038856278473, 4.625000000000000000, -5.798097038856279362 ) ) ;
#3429=CARTESIAN_POINT ( 'NONE',  ( 1.346194077712558279, 11.56250000000000000, -6.750000000000000000 ) ) ;
#3433=CARTESIAN_POINT ( 'NONE',  ( 0.000000000000000000, 8.500000000000000000, 0.2500000000000002220 ) ) ;
#3435=CARTESIAN_POINT ( 'NONE',  ( -3.750000000000000000, 7.687500000000000888, -1.946699141100893149 ) ) ;
#3436=CARTESIAN_POINT ( 'NONE',  ( 2.298097038856278029, 5.125000000000000888, -5.798097038856279362 ) ) ;
#3440=CARTESIAN_POINT ( 'NONE',  ( 3.249999999999999556, 3.750000000000000000, -3.500000000000000000 ) ) ;
#3441=CARTESIAN_POINT ( 'NONE',  ( -2.651650429449552870, 5.125000000000000000, -0.8483495705504462414 ) ) ;
#3451=CARTESIAN_POINT ( 'NONE',  ( -1.346194077712559167, 8.937500000000000000, -6.749999999999999112 ) ) ;
#3455=CARTESIAN_POINT ( 'NONE',  ( -3.749999999999999556, 8.750000000000001776, -3.499999999999999112 ) ) ;
#3456=CARTESIAN_POINT ( 'NONE',  ( 3.749999999999999556, 12.81250000000000178, -1.946699141100892261 ) ) ;
#3460=CARTESIAN_POINT ( 'NONE',  ( 1.553300858899105963, 13.06249999999999822, -7.250000000000000888 ) ) ;
#3469=CARTESIAN_POINT ( 'NONE',  ( 2.298097038856278473, 2.625000000000000000, -5.798097038856279362 ) ) ;
#3472=CARTESIAN_POINT ( 'NONE',  ( 3.249999999999998224, 8.312500000000003553, -2.153805922287439945 ) ) ;
#3480=CARTESIAN_POINT ( 'NONE',  ( -3.249999999999999112, 10.68750000000000178, -2.153805922287440833 ) ) ;
#3482=CARTESIAN_POINT ( 'NONE',  ( 3.749999999999999556, 1.250000000000000222, -3.500000000000000444 ) ) ;
#3483=CARTESIAN_POINT ( 'NONE',  ( -0.3766621274091715987, -0.2374287473167014662, 0.07324965529007555765 ) ) ;
#3489=CARTESIAN_POINT ( 'NONE',  ( 1.346194077712558057, 11.56249999999999822, -6.750000000000000000 ) ) ;
#3497=CARTESIAN_POINT ( 'NONE',  ( -3.749999999999999556, 5.187500000000001776, -1.946699141100892927 ) ) ;
#3498=CARTESIAN_POINT ( 'NONE',  ( -1.553300858899106629, 3.562500000000000888, 0.2499999999999998335 ) ) ;
#3499=CARTESIAN_POINT ( 'NONE',  ( 0.3766621274091715987, -0.2500000000000000000, 0.1491815183709511716 ) ) ;
#3502=CARTESIAN_POINT ( 'NONE',  ( -3.249999999999999556, 14.25000000000000000, -3.499999999999999556 ) ) ;
#3505=CARTESIAN_POINT ( 'NONE',  ( 3.249999999999999112, 3.812500000000000000, -2.153805922287439945 ) ) ;
#3513=CARTESIAN_POINT ( 'NONE',  ( -2.298097038856278473, 14.12500000000000000, -1.201902961143720416 ) ) ;
#3517=CARTESIAN_POINT ( 'NONE',  ( 2.651650429449552870, 6.125000000000000000, -6.151650429449555091 ) ) ;
#3518=CARTESIAN_POINT ( 'NONE',  ( 3.249999999999998224, 8.312500000000003553, -2.153805922287439945 ) ) ;
#3521=CARTESIAN_POINT ( 'NONE',  ( -3.249999999999999556, 2.187500000000000444, -2.153805922287440833 ) ) ;
#3522=CARTESIAN_POINT ( 'NONE',  ( 0.000000000000000000, 9.000000000000001776, 0.2500000000000002220 ) ) ;
#3525=CARTESIAN_POINT ( 'NONE',  ( 0.000000000000000000, 15.00000000000000000, 0.2500000000000002220 ) ) ;
#3530=CARTESIAN_POINT ( 'NONE',  ( -2.298097038856279362, 8.875000000000000000, -5.798097038856278473 ) ) ;
#3534=CARTESIAN_POINT ( 'NONE',  ( 1.553300858899109071, 12.43750000000000000, 0.2499999999999989175 ) ) ;
#3538=CARTESIAN_POINT ( 'NONE',  ( 2.651650429449554203, 14.37500000000000000, -0.8483495705504471296 ) ) ;
#3548=CARTESIAN_POINT ( 'NONE',  ( 3.249999999999998668, 1.687500000000000000, -4.846194077712560500 ) ) ;
#3550=CARTESIAN_POINT ( 'NONE',  ( -3.249999999999999556, 8.750000000000000000, -3.500000000000000000 ) ) ;
#3557=CARTESIAN_POINT ( 'NONE',  ( 1.346194077712561166, 11.43750000000000178, -0.2500000000000011102 ) ) ;
#3559=CARTESIAN_POINT ( 'NONE',  ( 1.553300858899108849, 6.937500000000000000, 0.2499999999999993616 ) ) ;
#3561=CARTESIAN_POINT ( 'NONE',  ( -3.749999999999999556, 0.7500000000000001110, -3.499999999999999112 ) ) ;
#3569=CARTESIAN_POINT ( 'NONE',  ( -2.298097038856278473, 11.12500000000000000, -1.201902961143720416 ) ) ;
#3577=CARTESIAN_POINT ( 'NONE',  ( 3.749999999999999112, 5.812500000000000000, -1.946699141100892039 ) ) ;
#3578=CARTESIAN_POINT ( 'NONE',  ( -3.749999999999999556, 4.750000000000000000, -3.499999999999999112 ) ) ;
#3583=CARTESIAN_POINT ( 'NONE',  ( -3.249999999999999556, 13.18749999999999822, -2.153805922287440833 ) ) ;
#3587=CARTESIAN_POINT ( 'NONE',  ( 3.249999999999998668, 5.687500000000000000, -4.846194077712560500 ) ) ;
#3597=LINE ( 'NONE', #5896, #1320 ) ;
#3598=CARTESIAN_POINT ( 'NONE',  ( 1.553300858899109516, 5.437500000000000888, 0.2499999999999993616 ) ) ;
#3599=CARTESIAN_POINT ( 'NONE',  ( -3.249999999999999112, 4.687500000000000888, -2.153805922287440833 ) ) ;
#3602=CARTESIAN_POINT ( 'NONE',  ( 1.346194077712558057, 2.562500000000000444, -6.750000000000000000 ) ) ;
#3610=CARTESIAN_POINT ( 'NONE',  ( -2.651650429449552870, 13.62500000000000000, -0.8483495705504467965 ) ) ;
#3614=CARTESIAN_POINT ( 'NONE',  ( 2.298097038856278029, 4.125000000000000000, -5.798097038856279362 ) ) ;
#3622=CARTESIAN_POINT ( 'NONE',  ( -3.249999999999999556, 3.250000000000000444, -3.499999999999999556 ) ) ;
#3624=CARTESIAN_POINT ( 'NONE',  ( 1.346194077712561166, 5.437500000000000888, -0.2500000000000011102 ) ) ;
#3627=AXIS2_PLACEMENT_3D ( 'NONE', #14889, #12471, #2827 ) ;
#3631=CARTESIAN_POINT ( 'NONE',  ( -3.249999999999999556, 2.250000000000000444, -3.499999999999999556 ) ) ;
#3632=CARTESIAN_POINT ( 'NONE',  ( 2.651650429449552870, 2.125000000000000000, -6.151650429449553314 ) ) ;
#3633=CARTESIAN_POINT ( 'NONE',  ( -1.553300858899106407, 5.062500000000000888, 0.2500000000000002220 ) ) ;
#3635=CARTESIAN_POINT ( 'NONE',  ( -3.750000000000000000, 7.812500000000000000, -5.053300858899105741 ) ) ;
#3640=CARTESIAN_POINT ( 'NONE',  ( 3.249999999999998668, 13.68750000000000000, -4.846194077712560500 ) ) ;
#3644=ORIENTED_EDGE ( 'NONE', *, *, #6843, .F. ) ;
#3647=CARTESIAN_POINT ( 'NONE',  ( 3.750000000000000000, 6.750000000000000000, -3.500000000000000444 ) ) ;
#3648=CARTESIAN_POINT ( 'NONE',  ( 2.651650429449553314, 4.375000000000000000, -0.8483495705504476847 ) ) ;
#3652=CARTESIAN_POINT ( 'NONE',  ( -1.346194077712559167, 3.937500000000000444, -6.749999999999999112 ) ) ;
#3657=CARTESIAN_POINT ( 'NONE',  ( -3.249999999999999556, 8.187500000000000000, -2.153805922287440833 ) ) ;
#3663=CARTESIAN_POINT ( 'NONE',  ( 0.000000000000000000, 0.2105996885190176970, -0.1347136637304948981 ) ) ;
#3664=CARTESIAN_POINT ( 'NONE',  ( 2.298097038856279362, 13.87500000000000000, -1.201902961143720860 ) ) ;
#3668=CARTESIAN_POINT ( 'NONE',  ( 3.749999999999999556, 5.250000000000000000, -3.500000000000000444 ) ) ;
#3669=CARTESIAN_POINT ( 'NONE',  ( -3.980102097228897738E-16, 8.999999999999998224, -6.749999999999999112 ) ) ;
#3672=CARTESIAN_POINT ( 'NONE',  ( -1.346194077712559389, 2.437500000000000444, -6.749999999999999112 ) ) ;
#3680=CARTESIAN_POINT ( 'NONE',  ( -2.651650429449552870, 14.62500000000000178, -0.8483495705504467965 ) ) ;
#3684=CARTESIAN_POINT ( 'NONE',  ( -3.249999999999999112, 3.812500000000000888, -4.846194077712558723 ) ) ;
#3693=CARTESIAN_POINT ( 'NONE',  ( -1.346194077712559167, 3.437500000000000000, -6.749999999999999112 ) ) ;
#3695=CARTESIAN_POINT ( 'NONE',  ( 0.000000000000000000, 15.00000000000000000, -0.2500000000000002220 ) ) ;
#3696=CARTESIAN_POINT ( 'NONE',  ( 3.249999999999998224, 5.187500000000001776, -4.846194077712561388 ) ) ;
#3702=CARTESIAN_POINT ( 'NONE',  ( -3.249999999999999556, 0.3125000000000000555, -4.846194077712557835 ) ) ;
#3703=CARTESIAN_POINT ( 'NONE',  ( 2.651650429449553314, 1.375000000000000000, -0.8483495705504476847 ) ) ;
#3705=CARTESIAN_POINT ( 'NONE',  ( 0.000000000000000000, 7.000000000000000000, 0.2500000000000002220 ) ) ;
#3707=CARTESIAN_POINT ( 'NONE',  ( -3.750000000000000000, 5.812500000000000888, -5.053300858899105741 ) ) ;
#3714=CARTESIAN_POINT ( 'NONE',  ( -3.249999999999999556, 11.25000000000000000, -3.499999999999999556 ) ) ;
#3721=CARTESIAN_POINT ( 'NONE',  ( 0.000000000000000000, 10.49999999999999822, 0.2500000000000002220 ) ) ;
#3725=CARTESIAN_POINT ( 'NONE',  ( -2.651650429449552870, 7.125000000000000000, -0.8483495705504462414 ) ) ;
#3726=CARTESIAN_POINT ( 'NONE',  ( 1.553300858899109071, 3.437500000000000444, 0.2499999999999989175 ) ) ;
#3727=LINE ( 'NONE', #8432, #7229 ) ;
#3729=CARTESIAN_POINT ( 'NONE',  ( 3.249999999999999556, 4.249999999999999112, -3.500000000000000000 ) ) ;
#3734=CARTESIAN_POINT ( 'NONE',  ( -2.298097038856278918, 8.375000000000000000, -5.798097038856277585 ) ) ;
#3748=CARTESIAN_POINT ( 'NONE',  ( 2.651650429449554203, 6.375000000000000888, -0.8483495705504471296 ) ) ;
#3749=CARTESIAN_POINT ( 'NONE',  ( 2.298097038856278029, 11.12500000000000000, -5.798097038856279362 ) ) ;
#3752=CARTESIAN_POINT ( 'NONE',  ( -3.249999999999999556, 6.187500000000000888, -2.153805922287440833 ) ) ;
#3762=VERTEX_POINT ( 'NONE', #910 ) ;
#3763=CARTESIAN_POINT ( 'NONE',  ( 1.346194077712560944, 9.937499999999998224, -0.2500000000000010547 ) ) ;
#3764=CARTESIAN_POINT ( 'NONE',  ( 3.249999999999999556, 13.25000000000000000, -3.500000000000000000 ) ) ;
#3767=CARTESIAN_POINT ( 'NONE',  ( -3.750000000000000000, 14.68750000000000178, -1.946699141100893149 ) ) ;
#3771=CARTESIAN_POINT ( 'NONE',  ( 3.249999999999999556, 2.249999999999999556, -3.500000000000000000 ) ) ;
#3776=ORIENTED_EDGE ( 'NONE', *, *, #2627, .T. ) ;
#3778=CARTESIAN_POINT ( 'NONE',  ( 3.249999999999998668, 5.687500000000000000, -4.846194077712560500 ) ) ;
#3781=CARTESIAN_POINT ( 'NONE',  ( -2.298097038856278918, 13.37500000000000000, -5.798097038856277585 ) ) ;
#3783=CARTESIAN_POINT ( 'NONE',  ( 3.249999999999998224, 5.312500000000000000, -2.153805922287439945 ) ) ;
#3787=CARTESIAN_POINT ( 'NONE',  ( 0.000000000000000000, 14.50000000000000355, -0.2500000000000002220 ) ) ;
#3788=CARTESIAN_POINT ( 'NONE',  ( -1.553300858899106407, 6.062500000000000000, 0.2500000000000002220 ) ) ;
#3790=CARTESIAN_POINT ( 'NONE',  ( -3.749999999999999556, 6.750000000000001776, -3.499999999999999112 ) ) ;
#3797=DIRECTION ( 'NONE',  ( 1.000000000000000000, -0.000000000000000000, 0.000000000000000000 ) ) ;
#3801=CARTESIAN_POINT ( 'NONE',  ( 1.553300858899105963, 11.06250000000000178, -7.250000000000000888 ) ) ;
#3805=CARTESIAN_POINT ( 'NONE',  ( 3.749999999999999112, 10.81250000000000178, -1.946699141100892039 ) ) ;
#3807=CARTESIAN_POINT ( 'NONE',  ( 3.749999999999999556, 9.250000000000001776, -3.500000000000000444 ) ) ;
#3812=CARTESIAN_POINT ( 'NONE',  ( 0.000000000000000000, 5.500000000000000000, -0.2500000000000002220 ) ) ;
#3813=CARTESIAN_POINT ( 'NONE',  ( 3.749999999999998668, 8.687500000000000000, -5.053300858899107517 ) ) ;
#3817=CARTESIAN_POINT ( 'NONE',  ( 2.298097038856278473, 7.625000000000000000, -5.798097038856279362 ) ) ;
#3825=CARTESIAN_POINT ( 'NONE',  ( -1.346194077712558945, 14.06250000000000178, -0.2500000000000002220 ) ) ;
#3829=CARTESIAN_POINT ( 'NONE',  ( -2.651650429449552870, 10.87500000000000000, -6.151650429449552426 ) ) ;
#3830=CARTESIAN_POINT ( 'NONE',  ( -1.346194077712558945, 7.562500000000000888, -0.2500000000000002220 ) ) ;
#3831=CARTESIAN_POINT ( 'NONE',  ( -3.249999999999999556, 8.750000000000000000, -3.500000000000000000 ) ) ;
#3835=CARTESIAN_POINT ( 'NONE',  ( -3.249999999999999556, 5.312500000000001776, -4.846194077712557835 ) ) ;
#3844=CARTESIAN_POINT ( 'NONE',  ( 2.298097038856278473, 0.6250000000000000000, -5.798097038856279362 ) ) ;
#3845=CARTESIAN_POINT ( 'NONE',  ( 1.553300858899108849, 13.93750000000000000, 0.2499999999999993616 ) ) ;
#3847=EDGE_CURVE ( 'NONE', #2992, #4833, #3916, .T. ) ;
#3848=CARTESIAN_POINT ( 'NONE',  ( -3.749999999999999556, 11.75000000000000178, -3.499999999999999112 ) ) ;
#3853=CARTESIAN_POINT ( 'NONE',  ( 3.249999999999999556, 1.250000000000000222, -3.500000000000000000 ) ) ;
#3860=CARTESIAN_POINT ( 'NONE',  ( 2.298097038856278473, 6.625000000000000000, -5.798097038856279362 ) ) ;
#3862=CARTESIAN_POINT ( 'NONE',  ( -3.249999999999999112, 0.8124999999999997780, -4.846194077712558723 ) ) ;
#3863=CARTESIAN_POINT ( 'NONE',  ( 2.298097038856279362, 10.37500000000000000, -1.201902961143720860 ) ) ;
#3867=CARTESIAN_POINT ( 'NONE',  ( -1.346194077712559389, 4.437500000000000888, -6.749999999999999112 ) ) ;
#3868=CARTESIAN_POINT ( 'NONE',  ( -2.298097038856279362, 14.87500000000000355, -5.798097038856278473 ) ) ;
#3870=CARTESIAN_POINT ( 'NONE',  ( -1.553300858899107073, 6.437500000000000888, -7.250000000000000000 ) ) ;
#3872=CARTESIAN_POINT ( 'NONE',  ( -1.553300858899106629, 5.562500000000001776, 0.2500000000000002220 ) ) ;
#3876=CARTESIAN_POINT ( 'NONE',  ( 0.000000000000000000, 11.00000000000000000, -0.2500000000000002220 ) ) ;
#3883=CARTESIAN_POINT ( 'NONE',  ( 3.749999999999999112, 11.18750000000000178, -5.053300858899108405 ) ) ;
#3887=CARTESIAN_POINT ( 'NONE',  ( 3.749999999999998668, 7.687500000000000000, -5.053300858899107517 ) ) ;
#3888=CARTESIAN_POINT ( 'NONE',  ( -2.651650429449552870, 9.875000000000000000, -6.151650429449552426 ) ) ;
#3891=CARTESIAN_POINT ( 'NONE',  ( -1.346194077712558945, 2.562500000000000444, -0.2500000000000002220 ) ) ;
#3892=CARTESIAN_POINT ( 'NONE',  ( 1.553300858899108849, 10.93750000000000000, 0.2499999999999993616 ) ) ;
#3897=CARTESIAN_POINT ( 'NONE',  ( 2.298097038856278473, 8.625000000000000000, -5.798097038856279362 ) ) ;
#3903=LINE ( 'NONE', #1653, #5689 ) ;
#3910=CARTESIAN_POINT ( 'NONE',  ( -1.553300858899106629, 12.56250000000000355, 0.2499999999999998335 ) ) ;
#3911=CARTESIAN_POINT ( 'NONE',  ( -2.298097038856279362, 10.87500000000000000, -5.798097038856278473 ) ) ;
#3912=CARTESIAN_POINT ( 'NONE',  ( -1.346194077712559167, 11.93750000000000178, -6.749999999999999112 ) ) ;
#3915=CARTESIAN_POINT ( 'NONE',  ( 0.000000000000000000, 8.000000000000000000, -0.2500000000000002220 ) ) ;
#3916=LINE ( 'NONE', #4836, #15071 ) ;
#3923=CARTESIAN_POINT ( 'NONE',  ( 3.249999999999998224, 14.18750000000000178, -4.846194077712561388 ) ) ;
#3924=CARTESIAN_POINT ( 'NONE',  ( 3.749999999999998668, 11.68750000000000000, -5.053300858899107517 ) ) ;
#3926=CARTESIAN_POINT ( 'NONE',  ( 3.750000000000000000, 1.750000000000000000, -3.500000000000000444 ) ) ;
#3935=CARTESIAN_POINT ( 'NONE',  ( -1.346194077712559167, 7.437500000000000888, -6.749999999999999112 ) ) ;
#3938=CARTESIAN_POINT ( 'NONE',  ( 3.249999999999999556, 12.75000000000000178, -3.500000000000000000 ) ) ;
#3939=CARTESIAN_POINT ( 'NONE',  ( -3.980102097228897738E-16, 10.00000000000000000, -6.749999999999999112 ) ) ;
#3941=CARTESIAN_POINT ( 'NONE',  ( -1.346194077712559389, 0.4375000000000000555, -6.749999999999999112 ) ) ;
#3943=CARTESIAN_POINT ( 'NONE',  ( -3.249999999999999556, 3.250000000000000444, -3.499999999999999556 ) ) ;
#3944=CARTESIAN_POINT ( 'NONE',  ( -3.249999999999999556, 14.75000000000000000, -3.500000000000000000 ) ) ;
#3945=CARTESIAN_POINT ( 'NONE',  ( -1.553300858899107073, 10.43750000000000000, -7.250000000000000000 ) ) ;
#3948=CARTESIAN_POINT ( 'NONE',  ( 0.000000000000000000, 7.500000000000000888, 0.2500000000000002220 ) ) ;
#3958=CARTESIAN_POINT ( 'NONE',  ( 2.651650429449552870, 13.12499999999999822, -6.151650429449555091 ) ) ;
#3960=CARTESIAN_POINT ( 'NONE',  ( 0.000000000000000000, 3.061616997868383018E-17, 0.2500000000000002220 ) ) ;
#3963=CARTESIAN_POINT ( 'NONE',  ( 0.000000000000000000, 10.00000000000000000, 0.2500000000000002220 ) ) ;
#3964=CARTESIAN_POINT ( 'NONE',  ( 1.553300858899109071, 9.437500000000003553, 0.2499999999999989175 ) ) ;
#3968=CARTESIAN_POINT ( 'NONE',  ( -2.298097038856278029, 5.625000000000000000, -1.201902961143720638 ) ) ;
#3969=CARTESIAN_POINT ( 'NONE',  ( 3.750000000000000000, 11.75000000000000000, -3.500000000000000444 ) ) ;
#3974=CARTESIAN_POINT ( 'NONE',  ( 3.249999999999999556, 9.750000000000000000, -3.500000000000000000 ) ) ;
#3985=CARTESIAN_POINT ( 'NONE',  ( 0.2508815455408998085, 0.2972145640522015908, -6.863050255469942407 ) ) ;
#3986=CARTESIAN_POINT ( 'NONE',  ( -3.750000000000000000, 13.81250000000000178, -5.053300858899105741 ) ) ;
#3987=CARTESIAN_POINT ( 'NONE',  ( 1.346194077712558279, 12.06250000000000000, -6.750000000000000888 ) ) ;
#3988=CARTESIAN_POINT ( 'NONE',  ( -2.298097038856278029, 10.62500000000000000, -1.201902961143720638 ) ) ;
#3993=CARTESIAN_POINT ( 'NONE',  ( 2.298097038856279362, 8.875000000000001776, -1.201902961143720860 ) ) ;
#3997=FACE_OUTER_BOUND ( 'NONE', #5565, .T. ) ;
#4003=CARTESIAN_POINT ( 'NONE',  ( 1.346194077712560944, 1.937500000000000000, -0.2500000000000010547 ) ) ;
#4004=CARTESIAN_POINT ( 'NONE',  ( 1.553300858899108849, 14.93750000000000178, 0.2499999999999993616 ) ) ;
#4008=CARTESIAN_POINT ( 'NONE',  ( 3.749999999999999112, 2.812500000000000000, -1.946699141100892039 ) ) ;
#4011=CARTESIAN_POINT ( 'NONE',  ( -2.651650429449552870, 1.125000000000000222, -0.8483495705504462414 ) ) ;
#4017=CARTESIAN_POINT ( 'NONE',  ( -3.980102097228897245E-16, 8.500000000000000000, -6.749999999999999112 ) ) ;
#4019=CARTESIAN_POINT ( 'NONE',  ( -1.346194077712559389, 12.06250000000000000, -0.2500000000000002220 ) ) ;
#4020=CARTESIAN_POINT ( 'NONE',  ( -3.249999999999999112, 8.812500000000001776, -4.846194077712558723 ) ) ;
#4024=CARTESIAN_POINT ( 'NONE',  ( -3.249999999999999556, 4.250000000000000000, -3.499999999999999556 ) ) ;
#4025=CARTESIAN_POINT ( 'NONE',  ( 2.651650429449553314, 7.375000000000000000, -0.8483495705504476847 ) ) ;
#4026=CARTESIAN_POINT ( 'NONE',  ( 0.000000000000000000, 9.000000000000001776, 0.2500000000000002220 ) ) ;
#4030=CARTESIAN_POINT ( 'NONE',  ( 2.651650429449552870, 11.12500000000000000, -6.151650429449555091 ) ) ;
#4038=CARTESIAN_POINT ( 'NONE',  ( -1.553300858899107073, 11.93750000000000178, -7.249999999999999112 ) ) ;
#4042=CARTESIAN_POINT ( 'NONE',  ( -2.651650429449553314, 7.375000000000000888, -6.151650429449552426 ) ) ;
#4043=CARTESIAN_POINT ( 'NONE',  ( -4.592425496802573972E-16, 10.00000000000000000, -7.250000000000000000 ) ) ;
#4046=VECTOR ( 'NONE', #1485, 1000.000000000000000 ) ;
#4047=CARTESIAN_POINT ( 'NONE',  ( -3.249999999999999112, 6.812500000000000000, -4.846194077712558723 ) ) ;
#4050=CARTESIAN_POINT ( 'NONE',  ( 1.553300858899108849, 8.937500000000001776, 0.2499999999999993616 ) ) ;
#4057=CARTESIAN_POINT ( 'NONE',  ( 1.346194077712558057, 12.56250000000000000, -6.750000000000000000 ) ) ;
#4066=ORIENTED_EDGE ( 'NONE', *, *, #2714, .F. ) ;
#4069=CARTESIAN_POINT ( 'NONE',  ( -1.553300858899107073, 12.93750000000000178, -7.249999999999999112 ) ) ;
#4070=CARTESIAN_POINT ( 'NONE',  ( 3.249999999999998224, 10.31250000000000000, -2.153805922287439945 ) ) ;
#4071=CARTESIAN_POINT ( 'NONE',  ( -1.346194077712558945, 13.56250000000000000, -0.2500000000000002220 ) ) ;
#4072=EDGE_LOOP ( 'NONE', ( #11467, #9318 ) ) ;
#4073=CARTESIAN_POINT ( 'NONE',  ( 3.249999999999999112, 12.81250000000000000, -2.153805922287439945 ) ) ;
#4082=CARTESIAN_POINT ( 'NONE',  ( 3.249999999999999556, 14.25000000000000178, -3.500000000000000000 ) ) ;
#4084=CARTESIAN_POINT ( 'NONE',  ( 1.553300858899105963, 12.56250000000000000, -7.250000000000000888 ) ) ;
#4087=CARTESIAN_POINT ( 'NONE',  ( -1.553300858899107295, 1.437500000000000000, -7.250000000000000000 ) ) ;
#4091=CARTESIAN_POINT ( 'NONE',  ( 2.651650429449552870, 2.625000000000000000, -6.151650429449554203 ) ) ;
#4096=CARTESIAN_POINT ( 'NONE',  ( -3.249999999999999556, 5.187500000000000888, -2.153805922287440833 ) ) ;
#4098=CARTESIAN_POINT ( 'NONE',  ( 2.298097038856279362, 1.375000000000000000, -1.201902961143720860 ) ) ;
#4101=CARTESIAN_POINT ( 'NONE',  ( 0.000000000000000000, 11.50000000000000000, -0.2500000000000002220 ) ) ;
#4104=CARTESIAN_POINT ( 'NONE',  ( -2.298097038856278473, 5.125000000000000000, -1.201902961143720416 ) ) ;
#4105=CARTESIAN_POINT ( 'NONE',  ( -1.553300858899106629, 6.562500000000000888, 0.2499999999999998335 ) ) ;
#4106=CARTESIAN_POINT ( 'NONE',  ( -2.651650429449553314, 9.375000000000000000, -6.151650429449552426 ) ) ;
#4109=CARTESIAN_POINT ( 'NONE',  ( -3.750000000000000000, 8.812500000000001776, -5.053300858899105741 ) ) ;
#4114=CARTESIAN_POINT ( 'NONE',  ( 1.346194077712560944, 14.93750000000000178, -0.2500000000000010547 ) ) ;
#4118=CARTESIAN_POINT ( 'NONE',  ( 3.749999999999999556, 13.25000000000000000, -3.500000000000000444 ) ) ;
#4122=CARTESIAN_POINT ( 'NONE',  ( -3.750000000000000000, 11.25000000000000000, -3.499999999999999112 ) ) ;
#4123=CARTESIAN_POINT ( 'NONE',  ( -3.750000000000000000, 9.687500000000000000, -1.946699141100893149 ) ) ;
#4125=CARTESIAN_POINT ( 'NONE',  ( -1.346194077712558945, 8.562500000000001776, -0.2500000000000002220 ) ) ;
#4126=CARTESIAN_POINT ( 'NONE',  ( 3.749999999999999112, 12.81250000000000000, -1.946699141100892039 ) ) ;
#4131=CARTESIAN_POINT ( 'NONE',  ( 3.249999999999999112, 12.81250000000000000, -2.153805922287439945 ) ) ;
#4141=CARTESIAN_POINT ( 'NONE',  ( 3.749999999999999112, 12.31250000000000178, -1.946699141100893149 ) ) ;
#4142=CARTESIAN_POINT ( 'NONE',  ( 2.298097038856279362, 10.37500000000000000, -1.201902961143720860 ) ) ;
#4144=CARTESIAN_POINT ( 'NONE',  ( -3.249999999999999112, 12.81250000000000178, -4.846194077712558723 ) ) ;
#4147=CARTESIAN_POINT ( 'NONE',  ( 3.249999999999998668, 11.68750000000000000, -4.846194077712560500 ) ) ;
#4155=CARTESIAN_POINT ( 'NONE',  ( 0.000000000000000000, 4.000000000000000000, -0.2500000000000002220 ) ) ;
#4156=CARTESIAN_POINT ( 'NONE',  ( 0.3766621274091715987, 0.5000000000000000000, -0.1347136637304948981 ) ) ;
#4157=CARTESIAN_POINT ( 'NONE',  ( 2.651650429449552870, 13.62500000000000000, -6.151650429449554203 ) ) ;
#4161=CARTESIAN_POINT ( 'NONE',  ( 1.553300858899108849, 2.937500000000000444, 0.2499999999999993616 ) ) ;
#4164=CARTESIAN_POINT ( 'NONE',  ( 3.750000000000000000, 0.7500000000000000000, -3.500000000000000444 ) ) ;
#4169=CARTESIAN_POINT ( 'NONE',  ( -0.2513523046203912648, 0.2269315213422933297, -0.1347136637270276993 ) ) ;
#4170=CARTESIAN_POINT ( 'NONE',  ( -2.298097038856278029, 2.625000000000000000, -1.201902961143720638 ) ) ;
#4171=CARTESIAN_POINT ( 'NONE',  ( -3.249999999999999556, 10.75000000000000000, -3.500000000000000000 ) ) ;
#4174=CARTESIAN_POINT ( 'NONE',  ( 2.298097038856279362, 5.875000000000000000, -1.201902961143720860 ) ) ;
#4175=CARTESIAN_POINT ( 'NONE',  ( -3.750000000000000000, 5.687500000000000888, -1.946699141100893149 ) ) ;
#4176=CARTESIAN_POINT ( 'NONE',  ( 1.553300858899108849, 8.937500000000001776, 0.2499999999999993616 ) ) ;
#4180=CARTESIAN_POINT ( 'NONE',  ( 1.553300858899109516, 8.437500000000000000, 0.2499999999999993616 ) ) ;
#4188=CARTESIAN_POINT ( 'NONE',  ( -1.553300858899106629, 12.56250000000000355, 0.2500000000000002220 ) ) ;
#4192=CARTESIAN_POINT ( 'NONE',  ( 0.000000000000000000, 10.50000000000000000, 0.2499999999999998057 ) ) ;
#4194=CARTESIAN_POINT ( 'NONE',  ( 2.298097038856279362, 9.374999999999998224, -1.201902961143720860 ) ) ;
#4197=CARTESIAN_POINT ( 'NONE',  ( 0.000000000000000000, 12.00000000000000000, 0.2500000000000002220 ) ) ;
#4201=CARTESIAN_POINT ( 'NONE',  ( 3.249999999999999556, 12.75000000000000178, -3.500000000000000000 ) ) ;
#4204=CARTESIAN_POINT ( 'NONE',  ( -0.3766621274091715987, 0.5000000000000000000, 0.1491815183709511716 ) ) ;
#4205=CARTESIAN_POINT ( 'NONE',  ( 0.000000000000000000, 7.000000000000000000, -0.2500000000000002220 ) ) ;
#4212=CARTESIAN_POINT ( 'NONE',  ( 0.000000000000000000, 3.061616997868383018E-17, 0.2500000000000002220 ) ) ;
#4213=CARTESIAN_POINT ( 'NONE',  ( 1.346194077712561166, 11.43750000000000178, -0.2500000000000011102 ) ) ;
#4214=CARTESIAN_POINT ( 'NONE',  ( -2.298097038856278473, 1.125000000000000222, -1.201902961143720416 ) ) ;
#4216=CARTESIAN_POINT ( 'NONE',  ( -3.249999999999999556, 11.25000000000000000, -3.499999999999999556 ) ) ;
#4218=CARTESIAN_POINT ( 'NONE',  ( -0.3766621274091715987, -0.1687972351630583345, 0.1491815183709511161 ) ) ;
#4229=CARTESIAN_POINT ( 'NONE',  ( -2.298097038856278473, 4.125000000000000000, -1.201902961143720416 ) ) ;
#4231=CARTESIAN_POINT ( 'NONE',  ( 2.651650429449552870, 3.125000000000000444, -6.151650429449555091 ) ) ;
#4235=CARTESIAN_POINT ( 'NONE',  ( -3.749999999999999556, 1.312500000000000444, -5.053300858899104853 ) ) ;
#4240=CARTESIAN_POINT ( 'NONE',  ( -3.750000000000000000, 0.2500000000000000555, -3.499999999999999112 ) ) ;
#4246=DIRECTION ( 'NONE',  ( 0.000000000000000000, -1.000000000000000000, 0.000000000000000000 ) ) ;
#4249=CARTESIAN_POINT ( 'NONE',  ( -3.249999999999999556, 1.750000000000000000, -3.500000000000000000 ) ) ;
#4253=CARTESIAN_POINT ( 'NONE',  ( -1.553300858899107073, 6.937500000000001776, -7.249999999999999112 ) ) ;
#4254=CARTESIAN_POINT ( 'NONE',  ( -4.592425496802573972E-16, 10.50000000000000000, -7.249999999999999112 ) ) ;
#4257=CARTESIAN_POINT ( 'NONE',  ( -2.651650429449552870, 8.624999999999998224, -0.8483495705504463524 ) ) ;
#4266=CARTESIAN_POINT ( 'NONE',  ( -2.298097038856278029, 1.625000000000000000, -1.201902961143720638 ) ) ;
#4273=CARTESIAN_POINT ( 'NONE',  ( 3.249999999999998224, 9.312500000000001776, -2.153805922287439945 ) ) ;
#4275=CARTESIAN_POINT ( 'NONE',  ( 3.750000000000000000, 14.75000000000000178, -3.500000000000000444 ) ) ;
#4276=AXIS2_PLACEMENT_3D ( 'NONE', #10281, #15246, #1006 ) ;
#4278=CARTESIAN_POINT ( 'NONE',  ( 1.346194077712560944, 11.93750000000000000, -0.2500000000000010547 ) ) ;
#4281=CARTESIAN_POINT ( 'NONE',  ( -2.298097038856278918, 9.375000000000000000, -5.798097038856277585 ) ) ;
#4288=CARTESIAN_POINT ( 'NONE',  ( -3.749999999999999556, 1.187500000000000444, -1.946699141100892927 ) ) ;
#4290=CARTESIAN_POINT ( 'NONE',  ( 1.346194077712561166, 14.43750000000000178, -0.2500000000000011102 ) ) ;
#4291=CARTESIAN_POINT ( 'NONE',  ( -3.249999999999999556, 0.3125000000000000555, -4.846194077712557835 ) ) ;
#4293=CARTESIAN_POINT ( 'NONE',  ( 2.298097038856278473, 10.62500000000000000, -5.798097038856279362 ) ) ;
#4296=DIRECTION ( 'NONE',  ( 1.000000000000000000, 0.000000000000000000, -0.000000000000000000 ) ) ;
#4305=CARTESIAN_POINT ( 'NONE',  ( -2.298097038856278473, 6.125000000000000000, -1.201902961143720416 ) ) ;
#4306=LINE ( 'NONE', #4156, #13679 ) ;
#4307=CARTESIAN_POINT ( 'NONE',  ( 1.553300858899109516, 3.437500000000000444, 0.2499999999999993616 ) ) ;
#4311=AXIS2_PLACEMENT_3D ( 'NONE', #8331, #6680, #14385 ) ;
#4313=CARTESIAN_POINT ( 'NONE',  ( 0.000000000000000000, 7.000000000000000000, 0.2500000000000002220 ) ) ;
#4316=CARTESIAN_POINT ( 'NONE',  ( 2.651650429449553759, 2.875000000000000000, -0.8483495705504471296 ) ) ;
#4319=AXIS2_PLACEMENT_3D ( 'NONE', #8834, #12308, #653 ) ;
#4320=FACE_OUTER_BOUND ( 'NONE', #115, .T. ) ;
#4323=CARTESIAN_POINT ( 'NONE',  ( 2.298097038856279362, 3.375000000000000444, -1.201902961143720860 ) ) ;
#4327=CARTESIAN_POINT ( 'NONE',  ( -3.750000000000000000, 7.687500000000000000, -1.946699141100893149 ) ) ;
#4328=CARTESIAN_POINT ( 'NONE',  ( -3.750000000000000000, 12.25000000000000000, -3.499999999999999112 ) ) ;
#4332=CARTESIAN_POINT ( 'NONE',  ( -3.749999999999999556, 8.750000000000000000, -3.499999999999999112 ) ) ;
#4340=CARTESIAN_POINT ( 'NONE',  ( 0.000000000000000000, 1.500000000000000222, -0.2500000000000002220 ) ) ;
#4348=CARTESIAN_POINT ( 'NONE',  ( -2.298097038856279362, 7.874999999999999112, -5.798097038856278473 ) ) ;
#4349=CARTESIAN_POINT ( 'NONE',  ( -3.749999999999999556, -0.2499999999999998890, -3.499999999999999112 ) ) ;
#4352=CARTESIAN_POINT ( 'NONE',  ( -1.346194077712559389, 11.43750000000000000, -6.749999999999999112 ) ) ;
#4354=DIRECTION ( 'NONE',  ( -0.000000000000000000, -1.000000000000000000, -0.000000000000000000 ) ) ;
#4355=CARTESIAN_POINT ( 'NONE',  ( 1.346194077712558057, 8.562500000000001776, -6.750000000000000000 ) ) ;
#4358=VERTEX_POINT ( 'NONE', #5966 ) ;
#4361=CARTESIAN_POINT ( 'NONE',  ( 1.553300858899109071, 15.43750000000000178, 0.2499999999999989175 ) ) ;
#4362=CARTESIAN_POINT ( 'NONE',  ( 3.749999999999999556, 1.249999999999999778, -3.500000000000000444 ) ) ;
#4364=CARTESIAN_POINT ( 'NONE',  ( -3.249999999999999556, 1.312500000000000444, -4.846194077712557835 ) ) ;
#4366=CARTESIAN_POINT ( 'NONE',  ( 0.000000000000000000, 10.00000000000000000, -0.2500000000000002220 ) ) ;
#4370=CARTESIAN_POINT ( 'NONE',  ( 0.000000000000000000, 15.00000000000000000, -0.2500000000000002220 ) ) ;
#4375=CARTESIAN_POINT ( 'NONE',  ( -3.249999999999999556, 11.18750000000000000, -2.153805922287440833 ) ) ;
#4377=CARTESIAN_POINT ( 'NONE',  ( -1.346194077712559389, 5.437500000000002665, -6.749999999999999112 ) ) ;
#4379=CARTESIAN_POINT ( 'NONE',  ( 1.553300858899105963, 0.06250000000000016653, -7.250000000000000888 ) ) ;
#4383=CARTESIAN_POINT ( 'NONE',  ( -3.249999999999999556, 0.3125000000000000555, -4.846194077712557835 ) ) ;
#4384=CARTESIAN_POINT ( 'NONE',  ( 3.750000000000000000, 5.750000000000000000, -3.500000000000000444 ) ) ;
#4392=CARTESIAN_POINT ( 'NONE',  ( 3.249999999999999556, 3.250000000000000000, -3.500000000000000000 ) ) ;
#4395=CARTESIAN_POINT ( 'NONE',  ( 2.651650429449553314, 9.374999999999998224, -0.8483495705504476847 ) ) ;
#4396=CARTESIAN_POINT ( 'NONE',  ( -1.553300858899107073, 12.43750000000000000, -7.250000000000000000 ) ) ;
#4399=CARTESIAN_POINT ( 'NONE',  ( -1.346194077712559167, 0.9375000000000002220, -6.749999999999999112 ) ) ;
#4406=CARTESIAN_POINT ( 'NONE',  ( -3.249999999999999112, 4.687500000000000888, -2.153805922287440833 ) ) ;
#4408=CARTESIAN_POINT ( 'NONE',  ( -0.3766621274091715987, 0.5000000000000000000, -0.1347136637304948981 ) ) ;
#4410=CARTESIAN_POINT ( 'NONE',  ( 3.249999999999998668, 10.68750000000000000, -4.846194077712560500 ) ) ;
#4414=CARTESIAN_POINT ( 'NONE',  ( 3.249999999999998224, 14.31250000000000355, -2.153805922287439945 ) ) ;
#4416=CARTESIAN_POINT ( 'NONE',  ( -2.651650429449553314, -0.1249999999999999029, -6.151650429449552426 ) ) ;
#4426=CARTESIAN_POINT ( 'NONE',  ( 0.000000000000000000, 8.000000000000000000, -0.2500000000000002220 ) ) ;
#4432=CARTESIAN_POINT ( 'NONE',  ( -4.592425496802573972E-16, 1.500000000000000000, -7.249999999999999112 ) ) ;
#4433=CARTESIAN_POINT ( 'NONE',  ( 3.249999999999998224, 14.18750000000000178, -4.846194077712561388 ) ) ;
#4436=CARTESIAN_POINT ( 'NONE',  ( 3.249999999999998668, 13.68750000000000000, -4.846194077712560500 ) ) ;
#4437=DIRECTION ( 'NONE',  ( 1.000000000000000000, 0.000000000000000000, 0.000000000000000000 ) ) ;
#4447=CARTESIAN_POINT ( 'NONE',  ( -3.249999999999999556, 12.25000000000000000, -3.499999999999999556 ) ) ;
#4450=CARTESIAN_POINT ( 'NONE',  ( -1.346194077712559389, 5.062500000000001776, -0.2500000000000002220 ) ) ;
#4452=CARTESIAN_POINT ( 'NONE',  ( 0.000000000000000000, 2.500000000000000000, 0.2500000000000002220 ) ) ;
#4453=CARTESIAN_POINT ( 'NONE',  ( 2.298097038856278029, 6.125000000000000000, -5.798097038856279362 ) ) ;
#4459=CARTESIAN_POINT ( 'NONE',  ( 3.750000000000000000, 6.750000000000000000, -3.500000000000000444 ) ) ;
#4468=CARTESIAN_POINT ( 'NONE',  ( 0.000000000000000000, 7.499999999999999112, -0.2500000000000002220 ) ) ;
#4471=CARTESIAN_POINT ( 'NONE',  ( -3.750000000000000000, 10.81250000000000000, -5.053300858899105741 ) ) ;
#4472=CARTESIAN_POINT ( 'NONE',  ( -2.651650429449552870, 12.12500000000000000, -0.8483495705504462414 ) ) ;
#4475=CARTESIAN_POINT ( 'NONE',  ( 1.553300858899109516, 13.43750000000000178, 0.2499999999999993616 ) ) ;
#4483=CARTESIAN_POINT ( 'NONE',  ( -1.346194077712558945, 0.06250000000000000000, -0.2500000000000002220 ) ) ;
#4486=CARTESIAN_POINT ( 'NONE',  ( -3.249999999999999556, 1.750000000000000222, -3.500000000000000000 ) ) ;
#4492=EDGE_CURVE ( 'NONE', #1124, #9716, #416, .T. ) ;
#4494=CARTESIAN_POINT ( 'NONE',  ( 0.000000000000000000, 13.50000000000000355, -0.2500000000000002220 ) ) ;
#4496=CARTESIAN_POINT ( 'NONE',  ( 0.000000000000000000, 2.500000000000000000, 0.2500000000000002220 ) ) ;
#4502=CARTESIAN_POINT ( 'NONE',  ( 3.249999999999999556, 8.750000000000000000, -3.500000000000000000 ) ) ;
#4508=CARTESIAN_POINT ( 'NONE',  ( 3.750000000000000000, 3.750000000000000000, -3.500000000000000444 ) ) ;
#4509=CARTESIAN_POINT ( 'NONE',  ( -3.980102097228897738E-16, 15.00000000000000178, -6.749999999999999112 ) ) ;
#4514=CARTESIAN_POINT ( 'NONE',  ( -3.249999999999999556, 14.31250000000000000, -4.846194077712557835 ) ) ;
#4520=CARTESIAN_POINT ( 'NONE',  ( -3.249999999999999556, 2.250000000000000444, -3.499999999999999556 ) ) ;
#4527=CARTESIAN_POINT ( 'NONE',  ( -3.249999999999999556, 9.187500000000000000, -2.153805922287440833 ) ) ;
#4530=CARTESIAN_POINT ( 'NONE',  ( -3.750000000000000000, 11.68749999999999822, -1.946699141100893149 ) ) ;
#4532=CARTESIAN_POINT ( 'NONE',  ( 2.651650429449552870, 2.125000000000000000, -6.151650429449555091 ) ) ;
#4533=CARTESIAN_POINT ( 'NONE',  ( 3.249999999999999556, 7.250000000000001776, -3.500000000000000000 ) ) ;
#4536=CARTESIAN_POINT ( 'NONE',  ( -3.249999999999999556, 2.250000000000000444, -3.499999999999999556 ) ) ;
#4539=CARTESIAN_POINT ( 'NONE',  ( -3.750000000000000000, 6.250000000000000000, -3.499999999999999112 ) ) ;
#4547=VECTOR ( 'NONE', #13299, 1000.000000000000000 ) ;
#4549=CARTESIAN_POINT ( 'NONE',  ( -1.346194077712558945, 5.562500000000000000, -0.2500000000000002220 ) ) ;
#4551=CARTESIAN_POINT ( 'NONE',  ( 3.749999999999998668, 9.187500000000001776, -5.053300858899108405 ) ) ;
#4552=CARTESIAN_POINT ( 'NONE',  ( 3.750000000000000000, 11.75000000000000000, -3.500000000000000444 ) ) ;
#4555=CARTESIAN_POINT ( 'NONE',  ( -3.249999999999999556, -0.2499999999999998890, -3.500000000000000000 ) ) ;
#4560=VERTEX_POINT ( 'NONE', #12382 ) ;
#4562=CARTESIAN_POINT ( 'NONE',  ( -2.298097038856278918, 3.375000000000000000, -5.798097038856277585 ) ) ;
#4564=CARTESIAN_POINT ( 'NONE',  ( -2.298097038856279362, 2.875000000000000000, -5.798097038856278473 ) ) ;
#4570=CARTESIAN_POINT ( 'NONE',  ( 2.298097038856278029, 11.12500000000000178, -5.798097038856279362 ) ) ;
#4571=CARTESIAN_POINT ( 'NONE',  ( 0.3766621274091721538, 0.3292059843107342232, -7.146945437571387671 ) ) ;
#4572=CARTESIAN_POINT ( 'NONE',  ( 3.750000000000000000, 1.312500000000000444, -1.946699141100892705 ) ) ;
#4580=CARTESIAN_POINT ( 'NONE',  ( 0.000000000000000000, 13.00000000000000178, -0.2500000000000002220 ) ) ;
#4583=EDGE_LOOP ( 'NONE', ( #12957, #7204, #4066, #2528, #10336, #6565, #1287, #11922 ) ) ;
#4586=CARTESIAN_POINT ( 'NONE',  ( -1.553300858899107295, 5.437500000000002665, -7.250000000000000000 ) ) ;
#4587=CARTESIAN_POINT ( 'NONE',  ( -3.249999999999999112, 13.81250000000000178, -4.846194077712558723 ) ) ;
#4590=CARTESIAN_POINT ( 'NONE',  ( -3.249999999999999556, 0.7499999999999998890, -3.500000000000000000 ) ) ;
#4594=CARTESIAN_POINT ( 'NONE',  ( -3.980102097228897245E-16, 4.500000000000000888, -6.749999999999999112 ) ) ;
#4601=CARTESIAN_POINT ( 'NONE',  ( -3.249999999999999556, 12.31250000000000000, -4.846194077712557835 ) ) ;
#4604=CARTESIAN_POINT ( 'NONE',  ( -1.553300858899107073, 7.937500000000001776, -7.249999999999999112 ) ) ;
#4606=CARTESIAN_POINT ( 'NONE',  ( 3.749999999999999112, 7.187500000000000888, -5.053300858899108405 ) ) ;
#4607=CARTESIAN_POINT ( 'NONE',  ( 3.249999999999998224, 8.187500000000000000, -4.846194077712561388 ) ) ;
#4610=CARTESIAN_POINT ( 'NONE',  ( -3.980102097228897245E-16, 1.500000000000000000, -6.749999999999999112 ) ) ;
#4611=CARTESIAN_POINT ( 'NONE',  ( 3.749999999999999112, 5.812500000000000000, -1.946699141100892039 ) ) ;
#4620=CARTESIAN_POINT ( 'NONE',  ( -1.346194077712558945, 8.562500000000001776, -0.2500000000000002220 ) ) ;
#4622=CARTESIAN_POINT ( 'NONE',  ( -4.592425496802573972E-16, 11.00000000000000178, -7.250000000000000000 ) ) ;
#4624=CARTESIAN_POINT ( 'NONE',  ( -2.651650429449553314, 12.37500000000000000, -6.151650429449552426 ) ) ;
#4627=CARTESIAN_POINT ( 'NONE',  ( -2.298097038856278029, -0.3749999999999998890, -1.201902961143720638 ) ) ;
#4634=CARTESIAN_POINT ( 'NONE',  ( 2.298097038856278473, 4.625000000000000000, -5.798097038856279362 ) ) ;
#4636=CARTESIAN_POINT ( 'NONE',  ( 3.249999999999998224, 8.187500000000000000, -4.846194077712561388 ) ) ;
#4642=CARTESIAN_POINT ( 'NONE',  ( -1.346194077712558945, 13.56250000000000000, -0.2500000000000002220 ) ) ;
#4644=CARTESIAN_POINT ( 'NONE',  ( -2.651650429449552870, 2.625000000000000000, -0.8483495705504463524 ) ) ;
#4649=CARTESIAN_POINT ( 'NONE',  ( -1.346194077712559389, 14.06249999999999822, -0.2500000000000002220 ) ) ;
#4655=CARTESIAN_POINT ( 'NONE',  ( 2.651650429449552870, 4.625000000000000000, -6.151650429449554203 ) ) ;
#4656=CARTESIAN_POINT ( 'NONE',  ( -2.651650429449552870, 5.625000000000000000, -0.8483495705504467965 ) ) ;
#4659=CARTESIAN_POINT ( 'NONE',  ( -3.249999999999999112, 0.6875000000000000000, -2.153805922287440833 ) ) ;
#4665=CARTESIAN_POINT ( 'NONE',  ( -1.346194077712559389, 2.062500000000000000, -0.2500000000000002220 ) ) ;
#4671=CARTESIAN_POINT ( 'NONE',  ( 3.249999999999998668, 13.68750000000000000, -4.846194077712560500 ) ) ;
#4675=CARTESIAN_POINT ( 'NONE',  ( -3.750000000000000000, 4.687500000000000888, -1.946699141100893149 ) ) ;
#4676=CARTESIAN_POINT ( 'NONE',  ( 0.000000000000000000, 5.500000000000000888, -0.2500000000000002220 ) ) ;
#4679=CARTESIAN_POINT ( 'NONE',  ( -1.346194077712559389, 4.437500000000000888, -6.749999999999999112 ) ) ;
#4681=CARTESIAN_POINT ( 'NONE',  ( -1.553300858899107295, 10.43750000000000000, -7.250000000000000000 ) ) ;
#4689=CARTESIAN_POINT ( 'NONE',  ( 2.298097038856279362, 7.375000000000000000, -1.201902961143720860 ) ) ;
#4693=CARTESIAN_POINT ( 'NONE',  ( -1.553300858899107073, 11.93750000000000178, -7.249999999999999112 ) ) ;
#4700=CARTESIAN_POINT ( 'NONE',  ( 3.750000000000000000, 12.31250000000000178, -1.946699141100892705 ) ) ;
#4705=CARTESIAN_POINT ( 'NONE',  ( -2.298097038856278918, 14.37500000000000000, -5.798097038856277585 ) ) ;
#4709=CARTESIAN_POINT ( 'NONE',  ( 3.249999999999999112, 3.812500000000000000, -2.153805922287439945 ) ) ;
#4712=CARTESIAN_POINT ( 'NONE',  ( -3.249999999999999112, 6.687500000000000888, -2.153805922287440833 ) ) ;
#4719=CARTESIAN_POINT ( 'NONE',  ( 0.000000000000000000, 2.000000000000000000, -0.2500000000000002220 ) ) ;
#4720=CARTESIAN_POINT ( 'NONE',  ( -2.298097038856278029, 11.62500000000000000, -1.201902961143720638 ) ) ;
#4721=CARTESIAN_POINT ( 'NONE',  ( -0.1251224477187976580, 0.2925544614197072568, -7.146945437571384119 ) ) ;
#4722=CARTESIAN_POINT ( 'NONE',  ( 0.000000000000000000, 3.500000000000000000, 0.2500000000000002220 ) ) ;
#4728=CARTESIAN_POINT ( 'NONE',  ( -3.249999999999999556, 13.18749999999999822, -2.153805922287440833 ) ) ;
#4735=CARTESIAN_POINT ( 'NONE',  ( 3.749999999999999112, 3.812500000000000000, -1.946699141100892039 ) ) ;
#4736=CARTESIAN_POINT ( 'NONE',  ( 1.553300858899105963, 5.062500000000000000, -7.249999999999999112 ) ) ;
#4739=CARTESIAN_POINT ( 'NONE',  ( -2.298097038856278918, 13.37500000000000000, -5.798097038856277585 ) ) ;
#4742=CARTESIAN_POINT ( 'NONE',  ( -3.249999999999999556, 3.250000000000000444, -3.499999999999999556 ) ) ;
#4751=CARTESIAN_POINT ( 'NONE',  ( 0.000000000000000000, 0.2006112523677016646, 0.1491815183709511716 ) ) ;
#4752=CARTESIAN_POINT ( 'NONE',  ( 3.749999999999999556, 6.250000000000000888, -3.500000000000000444 ) ) ;
#4753=CARTESIAN_POINT ( 'NONE',  ( -2.298097038856278029, 7.625000000000001776, -1.201902961143720638 ) ) ;
#4757=CARTESIAN_POINT ( 'NONE',  ( 2.298097038856278473, 4.625000000000000000, -5.798097038856279362 ) ) ;
#4768=CARTESIAN_POINT ( 'NONE',  ( -1.553300858899107073, 14.93750000000000000, -7.249999999999999112 ) ) ;
#4772=CARTESIAN_POINT ( 'NONE',  ( 0.000000000000000000, 2.500000000000000000, -0.2500000000000002220 ) ) ;
#4782=CARTESIAN_POINT ( 'NONE',  ( -3.249999999999999556, 2.250000000000000444, -3.499999999999999556 ) ) ;
#4785=CARTESIAN_POINT ( 'NONE',  ( -3.249999999999999112, 7.812500000000000000, -4.846194077712558723 ) ) ;
#4791=CARTESIAN_POINT ( 'NONE',  ( -1.346194077712559389, 1.062500000000000222, -0.2500000000000002220 ) ) ;
#4793=CARTESIAN_POINT ( 'NONE',  ( -1.346194077712558945, 14.56250000000000000, -0.2500000000000002220 ) ) ;
#4794=CARTESIAN_POINT ( 'NONE',  ( 2.651650429449552870, 4.625000000000000000, -6.151650429449554203 ) ) ;
#4796=CARTESIAN_POINT ( 'NONE',  ( 2.651650429449552870, 7.125000000000000888, -6.151650429449555091 ) ) ;
#4801=CARTESIAN_POINT ( 'NONE',  ( 1.346194077712560944, 11.93750000000000000, -0.2500000000000010547 ) ) ;
#4809=LINE ( 'NONE', #9292, #15178 ) ;
#4810=CARTESIAN_POINT ( 'NONE',  ( 0.000000000000000000, 6.000000000000000000, 0.2500000000000002220 ) ) ;
#4811=CARTESIAN_POINT ( 'NONE',  ( -2.651650429449552870, 2.625000000000000000, -0.8483495705504467965 ) ) ;
#4816=CARTESIAN_POINT ( 'NONE',  ( 2.298097038856279362, 4.375000000000000000, -1.201902961143720860 ) ) ;
#4819=CARTESIAN_POINT ( 'NONE',  ( -2.298097038856278473, 3.125000000000000000, -1.201902961143720416 ) ) ;
#4821=APPLICATION_CONTEXT ( 'configuration controlled 3d designs of mechanical parts and assemblies' ) ;
#4830=CARTESIAN_POINT ( 'NONE',  ( -0.1255563994759004987, 0.2058028268504220881, 0.1491815183709512549 ) ) ;
#4831=CARTESIAN_POINT ( 'NONE',  ( -1.553300858899106629, 4.562500000000000000, 0.2500000000000002220 ) ) ;
#4832=CARTESIAN_POINT ( 'NONE',  ( -1.346194077712559167, 10.93750000000000000, -6.749999999999999112 ) ) ;
#4833=VERTEX_POINT ( 'NONE', #1095 ) ;
#4835=CARTESIAN_POINT ( 'NONE',  ( -3.249999999999999556, 3.250000000000000444, -3.499999999999999556 ) ) ;
#4836=CARTESIAN_POINT ( 'NONE',  ( -0.3766621274091715987, 0.5000000000000000000, 0.1491815183709511716 ) ) ;
#4842=CARTESIAN_POINT ( 'NONE',  ( 1.553300858899109071, 14.43750000000000178, 0.2499999999999989175 ) ) ;
#4848=CARTESIAN_POINT ( 'NONE',  ( 0.000000000000000000, 4.499999999999999112, -0.2500000000000002220 ) ) ;
#4855=CARTESIAN_POINT ( 'NONE',  ( 3.249999999999999556, 2.750000000000000000, -3.500000000000000000 ) ) ;
#4857=CARTESIAN_POINT ( 'NONE',  ( -2.298097038856278473, 12.12500000000000000, -1.201902961143720416 ) ) ;
#4858=CARTESIAN_POINT ( 'NONE',  ( -3.249999999999999556, 7.750000000000000888, -3.500000000000000000 ) ) ;
#4864=CARTESIAN_POINT ( 'NONE',  ( 0.000000000000000000, 0.4999999999999999445, 0.2499999999999998057 ) ) ;
#4865=CARTESIAN_POINT ( 'NONE',  ( -3.750000000000000000, 5.250000000000000000, -3.499999999999999112 ) ) ;
#4867=CARTESIAN_POINT ( 'NONE',  ( -3.749999999999999556, 5.750000000000000888, -3.499999999999999112 ) ) ;
#4873=CARTESIAN_POINT ( 'NONE',  ( -1.346194077712559389, 13.43749999999999822, -6.749999999999999112 ) ) ;
#4877=CARTESIAN_POINT ( 'NONE',  ( -1.553300858899107073, 9.937500000000001776, -7.249999999999999112 ) ) ;
#4881=CARTESIAN_POINT ( 'NONE',  ( 3.750000000000000000, 7.750000000000000000, -3.500000000000000444 ) ) ;
#4882=CARTESIAN_POINT ( 'NONE',  ( 2.651650429449553314, 5.375000000000000000, -0.8483495705504476847 ) ) ;
#4885=ORIENTED_EDGE ( 'NONE', *, *, #7532, .F. ) ;
#4887=CARTESIAN_POINT ( 'NONE',  ( -3.249999999999999112, 2.687500000000000888, -2.153805922287440833 ) ) ;
#4893=CARTESIAN_POINT ( 'NONE',  ( 2.298097038856279362, 9.875000000000000000, -1.201902961143720860 ) ) ;
#4903=CARTESIAN_POINT ( 'NONE',  ( 1.553300858899109516, 7.437500000000000000, 0.2499999999999993616 ) ) ;
#4904=CARTESIAN_POINT ( 'NONE',  ( 2.298097038856278029, 9.125000000000000000, -5.798097038856279362 ) ) ;
#4907=CARTESIAN_POINT ( 'NONE',  ( 3.249999999999998668, 7.687500000000000000, -4.846194077712560500 ) ) ;
#4916=CARTESIAN_POINT ( 'NONE',  ( 3.249999999999998668, 9.687500000000000000, -4.846194077712560500 ) ) ;
#4917=CARTESIAN_POINT ( 'NONE',  ( -1.346194077712559389, 1.062500000000000222, -0.2500000000000002220 ) ) ;
#4919=CARTESIAN_POINT ( 'NONE',  ( -2.651650429449552870, 13.87500000000000178, -6.151650429449552426 ) ) ;
#4922=CARTESIAN_POINT ( 'NONE',  ( 3.249999999999998224, 1.312500000000000444, -2.153805922287439945 ) ) ;
#4929=ORIENTED_EDGE ( 'NONE', *, *, #2502, .T. ) ;
#4931=CARTESIAN_POINT ( 'NONE',  ( -3.249999999999999556, 6.250000000000000000, -3.499999999999999556 ) ) ;
#4932=EDGE_CURVE ( 'NONE', #5961, #6131, #1244, .T. ) ;
#4934=CARTESIAN_POINT ( 'NONE',  ( 2.298097038856278029, 1.124999999999999778, -5.798097038856279362 ) ) ;
#4935=CARTESIAN_POINT ( 'NONE',  ( -1.346194077712558945, 7.562500000000000888, -0.2500000000000002220 ) ) ;
#4940=CARTESIAN_POINT ( 'NONE',  ( 1.346194077712560944, 1.937500000000000000, -0.2500000000000010547 ) ) ;
#4941=CARTESIAN_POINT ( 'NONE',  ( -3.750000000000000000, 1.687499999999999778, -1.946699141100893149 ) ) ;
#4943=CARTESIAN_POINT ( 'NONE',  ( 1.553300858899105963, 6.562500000000000000, -7.250000000000000000 ) ) ;
#4945=CARTESIAN_POINT ( 'NONE',  ( -1.553300858899107073, 4.937500000000000888, -7.249999999999999112 ) ) ;
#4951=VECTOR ( 'NONE', #10044, 1000.000000000000000 ) ;
#4957=CARTESIAN_POINT ( 'NONE',  ( -2.651650429449553314, 10.87499999999999822, -6.151650429449552426 ) ) ;
#4961=CARTESIAN_POINT ( 'NONE',  ( -2.651650429449553314, 10.37500000000000000, -6.151650429449552426 ) ) ;
#4962=CARTESIAN_POINT ( 'NONE',  ( 2.651650429449553314, 6.374999999999999112, -0.8483495705504476847 ) ) ;
#4966=CARTESIAN_POINT ( 'NONE',  ( 1.346194077712561166, 3.437500000000000444, -0.2500000000000011102 ) ) ;
#4968=CARTESIAN_POINT ( 'NONE',  ( 0.000000000000000000, 11.00000000000000000, 0.2500000000000002220 ) ) ;
#4971=CARTESIAN_POINT ( 'NONE',  ( -2.298097038856278473, 9.125000000000000000, -1.201902961143720416 ) ) ;
#4975=ORIENTED_EDGE ( 'NONE', *, *, #3286, .T. ) ;
#4982=CARTESIAN_POINT ( 'NONE',  ( 0.1251546907736567626, 0.2964742070510372751, -6.863050255469943295 ) ) ;
#4984=CARTESIAN_POINT ( 'NONE',  ( 1.553300858899109071, 14.43750000000000178, 0.2499999999999989175 ) ) ;
#4985=CARTESIAN_POINT ( 'NONE',  ( -2.298097038856279362, 7.874999999999999112, -5.798097038856278473 ) ) ;
#4987=CARTESIAN_POINT ( 'NONE',  ( 3.249999999999998224, 11.18750000000000178, -4.846194077712561388 ) ) ;
#4988=ORIENTED_EDGE ( 'NONE', *, *, #7044, .F. ) ;
#4991=CARTESIAN_POINT ( 'NONE',  ( -2.298097038856278918, 5.375000000000000000, -5.798097038856277585 ) ) ;
#5000=CARTESIAN_POINT ( 'NONE',  ( 3.249999999999998224, 13.18750000000000000, -4.846194077712561388 ) ) ;
#5001=CARTESIAN_POINT ( 'NONE',  ( -3.749999999999999556, 12.18750000000000000, -1.946699141100892927 ) ) ;
#5003=PRODUCT_DEFINITION_FORMATION_WITH_SPECIFIED_SOURCE ( 'ANY', '', #8425, .NOT_KNOWN. ) ;
#5005=CARTESIAN_POINT ( 'NONE',  ( 3.749999999999999556, 13.25000000000000178, -3.500000000000000444 ) ) ;
#5009=CARTESIAN_POINT ( 'NONE',  ( -3.249999999999999112, 3.687500000000000444, -2.153805922287440833 ) ) ;
#5016=CARTESIAN_POINT ( 'NONE',  ( -3.980102097228897245E-16, 7.500000000000000000, -6.749999999999999112 ) ) ;
#5019=CARTESIAN_POINT ( 'NONE',  ( 1.346194077712558279, 1.062500000000000444, -6.750000000000000888 ) ) ;
#5020=CARTESIAN_POINT ( 'NONE',  ( -3.249999999999999112, 9.687500000000000000, -2.153805922287440833 ) ) ;
#5024=CARTESIAN_POINT ( 'NONE',  ( 3.249999999999998668, 4.687500000000000888, -4.846194077712560500 ) ) ;
#5025=CARTESIAN_POINT ( 'NONE',  ( -4.592425496802573972E-16, 2.000000000000000000, -7.250000000000000000 ) ) ;
#5026=CARTESIAN_POINT ( 'NONE',  ( -3.750000000000000000, 5.187500000000000888, -1.946699141100892927 ) ) ;
#5028=CARTESIAN_POINT ( 'NONE',  ( -2.651650429449552870, 7.625000000000001776, -0.8483495705504463524 ) ) ;
#5039=CARTESIAN_POINT ( 'NONE',  ( 3.750000000000000000, 10.31250000000000000, -1.946699141100892705 ) ) ;
#5043=CARTESIAN_POINT ( 'NONE',  ( -2.651650429449553314, 8.375000000000000000, -6.151650429449552426 ) ) ;
#5045=CARTESIAN_POINT ( 'NONE',  ( -3.749999999999999556, 9.750000000000000000, -3.499999999999999112 ) ) ;
#5049=CARTESIAN_POINT ( 'NONE',  ( 2.298097038856279362, 5.375000000000000000, -1.201902961143720860 ) ) ;
#5050=CARTESIAN_POINT ( 'NONE',  ( -3.749999999999999556, 8.187500000000000000, -1.946699141100892927 ) ) ;
#5055=CARTESIAN_POINT ( 'NONE',  ( 3.249999999999999556, 7.750000000000000000, -3.500000000000000000 ) ) ;
#5061=LINE ( 'NONE', #7447, #14599 ) ;
#5066=CARTESIAN_POINT ( 'NONE',  ( -2.651650429449552870, 11.62500000000000000, -0.8483495705504467965 ) ) ;
#5067=CARTESIAN_POINT ( 'NONE',  ( 1.346194077712558279, 13.06250000000000178, -6.750000000000000888 ) ) ;
#5068=CARTESIAN_POINT ( 'NONE',  ( -3.980102097228897738E-16, 12.00000000000000178, -6.749999999999999112 ) ) ;
#5071=CARTESIAN_POINT ( 'NONE',  ( 3.249999999999999556, 5.750000000000000000, -3.500000000000000000 ) ) ;
#5075=CARTESIAN_POINT ( 'NONE',  ( -0.3766621274091715987, 0.5000000000000000000, 0.1491815183709511716 ) ) ;
#5080=CARTESIAN_POINT ( 'NONE',  ( -2.298097038856278918, 9.375000000000000000, -5.798097038856277585 ) ) ;
#5081=CARTESIAN_POINT ( 'NONE',  ( 3.249999999999998668, 1.687500000000000000, -4.846194077712560500 ) ) ;
#5082=CARTESIAN_POINT ( 'NONE',  ( 2.651650429449552870, 11.62500000000000000, -6.151650429449554203 ) ) ;
#5084=CARTESIAN_POINT ( 'NONE',  ( 3.749999999999998668, 3.687500000000000444, -5.053300858899107517 ) ) ;
#5091=CARTESIAN_POINT ( 'NONE',  ( -0.3766621274091715987, -0.2500000000000000000, 0.1491815183709511716 ) ) ;
#5094=CARTESIAN_POINT ( 'NONE',  ( -3.249999999999999556, 5.250000000000000000, -3.499999999999999556 ) ) ;
#5096=CARTESIAN_POINT ( 'NONE',  ( 3.249999999999999112, 14.81250000000000000, -2.153805922287439945 ) ) ;
#5097=CARTESIAN_POINT ( 'NONE',  ( 1.346194077712558279, 9.062500000000000000, -6.750000000000000888 ) ) ;
#5101=CARTESIAN_POINT ( 'NONE',  ( -3.249999999999999556, 5.250000000000000000, -3.499999999999999556 ) ) ;
#5102=CARTESIAN_POINT ( 'NONE',  ( 2.651650429449552870, 3.125000000000000444, -6.151650429449553314 ) ) ;
#5103=CARTESIAN_POINT ( 'NONE',  ( -1.553300858899107073, 4.437500000000001776, -7.250000000000000000 ) ) ;
#5105=CARTESIAN_POINT ( 'NONE',  ( 0.000000000000000000, 5.500000000000000888, 0.2500000000000002220 ) ) ;
#5112=ORIENTED_EDGE ( 'NONE', *, *, #2197, .T. ) ;
#5113=CARTESIAN_POINT ( 'NONE',  ( 2.298097038856279362, 0.3750000000000001110, -1.201902961143720860 ) ) ;
#5117=CARTESIAN_POINT ( 'NONE',  ( 0.000000000000000000, 8.000000000000000000, 0.2500000000000002220 ) ) ;
#5118=CARTESIAN_POINT ( 'NONE',  ( -3.749999999999999556, 8.750000000000001776, -3.499999999999999112 ) ) ;
#5120=VERTEX_POINT ( 'NONE', #3525 ) ;
#5121=CARTESIAN_POINT ( 'NONE',  ( 1.346194077712561166, 5.437500000000000888, -0.2500000000000011102 ) ) ;
#5122=CARTESIAN_POINT ( 'NONE',  ( 1.553300858899108849, 7.937500000000000888, 0.2499999999999993616 ) ) ;
#5124=B_SPLINE_CURVE_WITH_KNOTS ( 'NONE', 3,
 ( #6091, #14469, #10807, #13222 ),
 .UNSPECIFIED., .F., .F.,
 ( 4, 4 ),
 ( 0.000000000000000000, 0.0003766969609235024303 ),
 .UNSPECIFIED. ) ;
#5128=CARTESIAN_POINT ( 'NONE',  ( 2.298097038856278473, 9.625000000000000000, -5.798097038856279362 ) ) ;
#5140=CARTESIAN_POINT ( 'NONE',  ( 1.553300858899109071, 13.43750000000000355, 0.2499999999999989175 ) ) ;
#5141=CARTESIAN_POINT ( 'NONE',  ( 0.000000000000000000, 12.50000000000000178, -0.2500000000000002220 ) ) ;
#5142=CARTESIAN_POINT ( 'NONE',  ( 0.000000000000000000, 10.49999999999999822, -0.2500000000000002220 ) ) ;
#5145=CARTESIAN_POINT ( 'NONE',  ( -3.249999999999999556, 8.312500000000000000, -4.846194077712557835 ) ) ;
#5153=CARTESIAN_POINT ( 'NONE',  ( -1.346194077712559389, 9.437500000000000000, -6.749999999999999112 ) ) ;
#5154=CARTESIAN_POINT ( 'NONE',  ( 2.298097038856279362, 1.875000000000000000, -1.201902961143720860 ) ) ;
#5155=CARTESIAN_POINT ( 'NONE',  ( 3.750000000000000000, 13.75000000000000000, -3.500000000000000444 ) ) ;
#5156=ORIENTED_EDGE ( 'NONE', *, *, #14209, .F. ) ;
#5159=CARTESIAN_POINT ( 'NONE',  ( 2.651650429449552870, 0.6250000000000000000, -6.151650429449554203 ) ) ;
#5163=CARTESIAN_POINT ( 'NONE',  ( 0.000000000000000000, 2.000000000000000000, 0.2500000000000002220 ) ) ;
#5166=DIRECTION ( 'NONE',  ( 0.000000000000000000, -0.000000000000000000, -1.000000000000000000 ) ) ;
#5169=CARTESIAN_POINT ( 'NONE',  ( -1.346194077712559167, 8.437500000000000000, -6.749999999999999112 ) ) ;
#5171=CARTESIAN_POINT ( 'NONE',  ( 2.298097038856279362, 12.87500000000000178, -1.201902961143720860 ) ) ;
#5173=CARTESIAN_POINT ( 'NONE',  ( -3.249999999999999556, 11.75000000000000178, -3.500000000000000000 ) ) ;
#5176=CARTESIAN_POINT ( 'NONE',  ( 0.000000000000000000, 1.000000000000000000, -0.2500000000000002220 ) ) ;
#5179=CARTESIAN_POINT ( 'NONE',  ( -1.346194077712559389, 6.062500000000000000, -0.2500000000000002220 ) ) ;
#5180=CARTESIAN_POINT ( 'NONE',  ( 3.749999999999998668, 6.187500000000001776, -5.053300858899108405 ) ) ;
#5181=CARTESIAN_POINT ( 'NONE',  ( 2.651650429449553759, 7.875000000000000000, -0.8483495705504471296 ) ) ;
#5184=CARTESIAN_POINT ( 'NONE',  ( -2.651650429449553314, 10.87499999999999822, -6.151650429449552426 ) ) ;
#5193=CARTESIAN_POINT ( 'NONE',  ( -3.750000000000000000, 12.81250000000000178, -5.053300858899105741 ) ) ;
#5197=CARTESIAN_POINT ( 'NONE',  ( -3.749999999999999556, 8.187500000000000000, -1.946699141100892927 ) ) ;
#5198=CARTESIAN_POINT ( 'NONE',  ( 3.749999999999998668, 8.187500000000000000, -5.053300858899108405 ) ) ;
#5202=CARTESIAN_POINT ( 'NONE',  ( 1.346194077712561166, 10.43750000000000178, -0.2500000000000011102 ) ) ;
#5203=CARTESIAN_POINT ( 'NONE',  ( -4.592425496802573972E-16, 8.500000000000000000, -7.249999999999999112 ) ) ;
#5208=CARTESIAN_POINT ( 'NONE',  ( -1.346194077712559389, 11.06250000000000000, -0.2500000000000002220 ) ) ;
#5209=AXIS2_PLACEMENT_3D ( 'NONE', #6681, #4437, #816 ) ;
#5220=CARTESIAN_POINT ( 'NONE',  ( 2.651650429449553314, 12.37500000000000178, -0.8483495705504476847 ) ) ;
#5221=CARTESIAN_POINT ( 'NONE',  ( -3.249999999999999112, 9.812500000000000000, -4.846194077712558723 ) ) ;
#5222=CARTESIAN_POINT ( 'NONE',  ( -1.346194077712559167, 13.93750000000000000, -6.749999999999999112 ) ) ;
#5227=CARTESIAN_POINT ( 'NONE',  ( 2.298097038856278473, 6.625000000000000000, -5.798097038856279362 ) ) ;
#5235=CARTESIAN_POINT ( 'NONE',  ( 1.346194077712558057, 0.5625000000000001110, -6.750000000000000000 ) ) ;
#5236=CARTESIAN_POINT ( 'NONE',  ( 2.651650429449553759, 12.87500000000000178, -0.8483495705504471296 ) ) ;
#5238=CARTESIAN_POINT ( 'NONE',  ( -1.553300858899106629, 2.062500000000000000, 0.2500000000000002220 ) ) ;
#5243=EDGE_CURVE ( 'NONE', #5493, #9716, #14047, .T. ) ;
#5248=CARTESIAN_POINT ( 'NONE',  ( -1.346194077712559167, 5.437500000000001776, -6.749999999999999112 ) ) ;
#5250=CARTESIAN_POINT ( 'NONE',  ( -3.980102097228897738E-16, 3.000000000000000444, -6.749999999999999112 ) ) ;
#5251=CARTESIAN_POINT ( 'NONE',  ( -3.249999999999999112, 11.81250000000000178, -4.846194077712558723 ) ) ;
#5254=CARTESIAN_POINT ( 'NONE',  ( -3.249999999999999556, 4.187500000000000000, -2.153805922287440833 ) ) ;
#5255=CARTESIAN_POINT ( 'NONE',  ( 3.749999999999998668, 5.187499999999999112, -5.053300858899108405 ) ) ;
#5256=CARTESIAN_POINT ( 'NONE',  ( -2.651650429449552870, 11.12500000000000000, -0.8483495705504462414 ) ) ;
#5259=CARTESIAN_POINT ( 'NONE',  ( -3.750000000000000000, 11.68749999999999822, -1.946699141100893149 ) ) ;
#5269=CARTESIAN_POINT ( 'NONE',  ( -3.750000000000000000, 12.68750000000000000, -1.946699141100893149 ) ) ;
#5273=CARTESIAN_POINT ( 'NONE',  ( -3.749999999999999556, 11.18749999999999822, -1.946699141100892927 ) ) ;
#5274=CARTESIAN_POINT ( 'NONE',  ( -3.749999999999999556, 6.750000000000000888, -3.499999999999999112 ) ) ;
#5278=CARTESIAN_POINT ( 'NONE',  ( -2.298097038856279362, 6.875000000000000000, -5.798097038856278473 ) ) ;
#5280=CARTESIAN_POINT ( 'NONE',  ( 2.651650429449552870, 0.1250000000000001110, -6.151650429449555091 ) ) ;
#5284=CARTESIAN_POINT ( 'NONE',  ( 3.249999999999999556, 13.75000000000000000, -3.500000000000000000 ) ) ;
#5289=AXIS2_PLACEMENT_3D ( 'NONE', #5577, #10292, #15029 ) ;
#5292=LINE ( 'NONE', #1810, #7133 ) ;
#5296=CARTESIAN_POINT ( 'NONE',  ( -3.749999999999999556, 12.75000000000000178, -3.499999999999999112 ) ) ;
#5297=CARTESIAN_POINT ( 'NONE',  ( 3.249999999999999556, 11.25000000000000178, -3.500000000000000000 ) ) ;
#5298=CARTESIAN_POINT ( 'NONE',  ( 3.249999999999999556, 14.25000000000000178, -3.500000000000000000 ) ) ;
#5300=CARTESIAN_POINT ( 'NONE',  ( 2.298097038856279362, 9.875000000000000000, -1.201902961143720860 ) ) ;
#5309=CARTESIAN_POINT ( 'NONE',  ( 1.346194077712558057, 4.562500000000000888, -6.750000000000000000 ) ) ;
#5311=CARTESIAN_POINT ( 'NONE',  ( 1.553300858899108849, 12.93750000000000000, 0.2499999999999993616 ) ) ;
#5314=CARTESIAN_POINT ( 'NONE',  ( 2.651650429449552870, 1.625000000000000222, -6.151650429449554203 ) ) ;
#5321=CARTESIAN_POINT ( 'NONE',  ( -2.298097038856278473, 9.125000000000000000, -1.201902961143720416 ) ) ;
#5323=CARTESIAN_POINT ( 'NONE',  ( 0.000000000000000000, 2.500000000000000000, -0.2500000000000002220 ) ) ;
#5324=CARTESIAN_POINT ( 'NONE',  ( 1.346194077712561166, 10.43750000000000178, -0.2500000000000011102 ) ) ;
#5328=CARTESIAN_POINT ( 'NONE',  ( 0.000000000000000000, 5.000000000000000000, -0.2500000000000002220 ) ) ;
#5329=CARTESIAN_POINT ( 'NONE',  ( -1.553300858899107073, 3.937500000000000444, -7.249999999999999112 ) ) ;
#5330=CARTESIAN_POINT ( 'NONE',  ( -1.553300858899107073, 11.43750000000000000, -7.250000000000000000 ) ) ;
#5333=CARTESIAN_POINT ( 'NONE',  ( 3.750000000000000000, 11.31250000000000000, -1.946699141100892705 ) ) ;
#5338=CARTESIAN_POINT ( 'NONE',  ( 2.298097038856278473, 0.6250000000000000000, -5.798097038856279362 ) ) ;
#5340=CARTESIAN_POINT ( 'NONE',  ( 3.749999999999999556, 14.25000000000000178, -3.500000000000000444 ) ) ;
#5344=CARTESIAN_POINT ( 'NONE',  ( 2.651650429449553314, 10.37500000000000000, -0.8483495705504476847 ) ) ;
#5348=CARTESIAN_POINT ( 'NONE',  ( -2.298097038856279362, 8.875000000000000000, -5.798097038856278473 ) ) ;
#5351=CARTESIAN_POINT ( 'NONE',  ( -2.651650429449552870, 12.12500000000000000, -0.8483495705504462414 ) ) ;
#5354=CARTESIAN_POINT ( 'NONE',  ( -1.346194077712559389, 12.43750000000000000, -6.749999999999999112 ) ) ;
#5364=CARTESIAN_POINT ( 'NONE',  ( 1.553300858899108849, 1.937500000000000000, 0.2499999999999993616 ) ) ;
#5365=CARTESIAN_POINT ( 'NONE',  ( -3.249999999999999112, 12.68750000000000178, -2.153805922287440833 ) ) ;
#5366=CARTESIAN_POINT ( 'NONE',  ( 2.298097038856279362, 0.8750000000000000000, -1.201902961143720860 ) ) ;
#5369=CARTESIAN_POINT ( 'NONE',  ( -3.249999999999999556, 11.18749999999999822, -2.153805922287440833 ) ) ;
#5371=EDGE_CURVE ( 'NONE', #13242, #559, #697, .T. ) ;
#5379=ORIENTED_EDGE ( 'NONE', *, *, #7026, .T. ) ;
#5380=CARTESIAN_POINT ( 'NONE',  ( 1.346194077712558057, 6.562500000000000000, -6.750000000000000000 ) ) ;
#5382=CARTESIAN_POINT ( 'NONE',  ( 3.750000000000000000, 2.312500000000000000, -1.946699141100892705 ) ) ;
#5385=CARTESIAN_POINT ( 'NONE',  ( -2.651650429449552870, 1.125000000000000222, -0.8483495705504462414 ) ) ;
#5389=CARTESIAN_POINT ( 'NONE',  ( -1.553300858899106407, 1.062500000000000222, 0.2500000000000002220 ) ) ;
#5395=CARTESIAN_POINT ( 'NONE',  ( -3.249999999999999556, 2.750000000000000444, -3.500000000000000000 ) ) ;
#5396=CARTESIAN_POINT ( 'NONE',  ( -3.249999999999999112, 12.81250000000000178, -4.846194077712558723 ) ) ;
#5400=CARTESIAN_POINT ( 'NONE',  ( -1.553300858899107073, 4.937500000000000000, -7.249999999999999112 ) ) ;
#5401=CARTESIAN_POINT ( 'NONE',  ( 3.749999999999999112, 7.687500000000000000, -5.053300858899108405 ) ) ;
#5405=CARTESIAN_POINT ( 'NONE',  ( -1.553300858899107073, 11.93750000000000178, -7.249999999999999112 ) ) ;
#5413=CARTESIAN_POINT ( 'NONE',  ( 3.249999999999998224, 0.3125000000000002220, -2.153805922287439945 ) ) ;
#5420=CARTESIAN_POINT ( 'NONE',  ( -3.249999999999999112, 7.687500000000000000, -2.153805922287440833 ) ) ;
#5422=CARTESIAN_POINT ( 'NONE',  ( 1.553300858899108849, 14.93750000000000178, 0.2499999999999993616 ) ) ;
#5425=CARTESIAN_POINT ( 'NONE',  ( -3.249999999999999556, 12.25000000000000000, -3.499999999999999556 ) ) ;
#5430=CARTESIAN_POINT ( 'NONE',  ( 2.298097038856278473, 8.625000000000000000, -5.798097038856279362 ) ) ;
#5436=CARTESIAN_POINT ( 'NONE',  ( 3.750000000000000000, 1.750000000000000000, -3.500000000000000444 ) ) ;
#5437=CARTESIAN_POINT ( 'NONE',  ( -3.750000000000000000, 0.6875000000000000000, -1.946699141100893149 ) ) ;
#5438=CARTESIAN_POINT ( 'NONE',  ( 2.298097038856278029, 14.12500000000000000, -5.798097038856279362 ) ) ;
#5440=CARTESIAN_POINT ( 'NONE',  ( 3.249999999999999112, 9.812500000000000000, -2.153805922287439945 ) ) ;
#5446=DIRECTION ( 'NONE',  ( -1.000000000000000000, 0.000000000000000000, 0.000000000000000000 ) ) ;
#5457=CARTESIAN_POINT ( 'NONE',  ( -1.346194077712559389, 3.062500000000000000, -0.2500000000000002220 ) ) ;
#5459=CARTESIAN_POINT ( 'NONE',  ( 1.553300858899109516, 0.4375000000000000555, 0.2499999999999993616 ) ) ;
#5463=LINE ( 'NONE', #14913, #7005 ) ;
#5464=CARTESIAN_POINT ( 'NONE',  ( -3.750000000000000000, 4.250000000000000000, -3.499999999999999112 ) ) ;
#5468=CARTESIAN_POINT ( 'NONE',  ( 1.553300858899105963, 1.562500000000000000, -7.250000000000000000 ) ) ;
#5469=SHAPE_DEFINITION_REPRESENTATION ( #11752, #9314 ) ;
#5474=CARTESIAN_POINT ( 'NONE',  ( -3.249999999999999112, 4.812500000000000000, -4.846194077712558723 ) ) ;
#5479=CARTESIAN_POINT ( 'NONE',  ( 3.749999999999999112, 5.312500000000000000, -1.946699141100893149 ) ) ;
#5480=CARTESIAN_POINT ( 'NONE',  ( 2.651650429449553759, 12.87500000000000178, -0.8483495705504471296 ) ) ;
#5483=CARTESIAN_POINT ( 'NONE',  ( 1.346194077712560944, 7.937500000000000888, -0.2500000000000010547 ) ) ;
#5484=CARTESIAN_POINT ( 'NONE',  ( 3.749999999999999112, 12.18750000000000178, -5.053300858899108405 ) ) ;
#5492=CARTESIAN_POINT ( 'NONE',  ( 3.249999999999998224, 4.187500000000000888, -4.846194077712561388 ) ) ;
#5493=VERTEX_POINT ( 'NONE', #12972 ) ;
#5498=CARTESIAN_POINT ( 'NONE',  ( -3.980102097228897738E-16, 10.00000000000000000, -6.749999999999999112 ) ) ;
#5500=CARTESIAN_POINT ( 'NONE',  ( 0.000000000000000000, 15.00000000000000000, 0.2500000000000002220 ) ) ;
#5503=CARTESIAN_POINT ( 'NONE',  ( -3.249999999999999556, 11.31249999999999822, -4.846194077712557835 ) ) ;
#5506=CARTESIAN_POINT ( 'NONE',  ( -3.249999999999999556, 10.18750000000000000, -2.153805922287440833 ) ) ;
#5512=CARTESIAN_POINT ( 'NONE',  ( -3.750000000000000000, 14.81250000000000355, -5.053300858899105741 ) ) ;
#5514=CARTESIAN_POINT ( 'NONE',  ( -2.651650429449552870, 1.874999999999999778, -6.151650429449552426 ) ) ;
#5515=CARTESIAN_POINT ( 'NONE',  ( -3.249999999999999556, 0.1875000000000000278, -2.153805922287440833 ) ) ;
#5517=CARTESIAN_POINT ( 'NONE',  ( 3.249999999999998668, 12.68750000000000178, -4.846194077712560500 ) ) ;
#5530=CARTESIAN_POINT ( 'NONE',  ( 3.249999999999999112, 2.812500000000000000, -2.153805922287439945 ) ) ;
#5532=CARTESIAN_POINT ( 'NONE',  ( 3.749999999999999556, 2.249999999999999556, -3.500000000000000444 ) ) ;
#5537=CARTESIAN_POINT ( 'NONE',  ( -3.749999999999999556, 6.187500000000000888, -1.946699141100892927 ) ) ;
#5541=CARTESIAN_POINT ( 'NONE',  ( -1.553300858899106407, 3.062500000000000000, 0.2500000000000002220 ) ) ;
#5545=DIRECTION ( 'NONE',  ( 0.000000000000000000, 0.000000000000000000, 1.000000000000000000 ) ) ;
#5547=CARTESIAN_POINT ( 'NONE',  ( -3.980102097228897738E-16, 4.000000000000000000, -6.749999999999999112 ) ) ;
#5549=CARTESIAN_POINT ( 'NONE',  ( -1.553300858899107073, 10.93750000000000355, -7.249999999999999112 ) ) ;
#5551=CARTESIAN_POINT ( 'NONE',  ( 3.750000000000000000, 13.75000000000000000, -3.500000000000000444 ) ) ;
#5555=CARTESIAN_POINT ( 'NONE',  ( -3.249999999999999556, 0.7500000000000001110, -3.500000000000000000 ) ) ;
#5564=CARTESIAN_POINT ( 'NONE',  ( 0.000000000000000000, 4.499999999999999112, -0.2500000000000002220 ) ) ;
#5565=EDGE_LOOP ( 'NONE', ( #1109, #10058, #2763, #15297, #7614, #9528, #6051, #1928 ) ) ;
#5569=CARTESIAN_POINT ( 'NONE',  ( -3.980102097228897245E-16, 10.50000000000000000, -6.749999999999999112 ) ) ;
#5572=CARTESIAN_POINT ( 'NONE',  ( -1.346194077712559167, 11.93750000000000178, -6.749999999999999112 ) ) ;
#5574=CARTESIAN_POINT ( 'NONE',  ( 2.651650429449552870, 14.62500000000000000, -6.151650429449554203 ) ) ;
#5577=CARTESIAN_POINT ( 'NONE',  ( 0.000000000000000000, 3.061616997868383018E-17, 0.2500000000000002220 ) ) ;
#5579=LINE ( 'NONE', #4204, #2837 ) ;
#5580=CARTESIAN_POINT ( 'NONE',  ( -3.249999999999999556, 7.187500000000000000, -2.153805922287440833 ) ) ;
#5586=CARTESIAN_POINT ( 'NONE',  ( -2.651650429449553314, 0.3750000000000000555, -6.151650429449552426 ) ) ;
#5587=CARTESIAN_POINT ( 'NONE',  ( -2.298097038856279362, 13.87500000000000178, -5.798097038856278473 ) ) ;
#5590=CARTESIAN_POINT ( 'NONE',  ( 0.000000000000000000, 12.00000000000000000, -0.2500000000000002220 ) ) ;
#5592=CARTESIAN_POINT ( 'NONE',  ( -3.980102097228897245E-16, 7.500000000000000000, -6.749999999999999112 ) ) ;
#5600=CARTESIAN_POINT ( 'NONE',  ( 1.346194077712560944, 11.93750000000000000, -0.2500000000000011102 ) ) ;
#5603=CARTESIAN_POINT ( 'NONE',  ( 1.346194077712560944, 2.937500000000000444, -0.2500000000000010547 ) ) ;
#5605=CARTESIAN_POINT ( 'NONE',  ( -3.749999999999999556, 1.750000000000000222, -3.499999999999999112 ) ) ;
#5606=CARTESIAN_POINT ( 'NONE',  ( -3.249999999999999112, 6.687500000000000888, -2.153805922287440833 ) ) ;
#5611=CARTESIAN_POINT ( 'NONE',  ( -4.592425496802573972E-16, 6.500000000000000888, -7.249999999999999112 ) ) ;
#5618=CARTESIAN_POINT ( 'NONE',  ( -3.980102097228897738E-16, 7.000000000000000000, -6.749999999999999112 ) ) ;
#5620=CARTESIAN_POINT ( 'NONE',  ( 0.000000000000000000, 8.500000000000000000, 0.2499999999999998057 ) ) ;
#5621=CARTESIAN_POINT ( 'NONE',  ( 2.651650429449553759, 14.87500000000000178, -0.8483495705504471296 ) ) ;
#5625=CARTESIAN_POINT ( 'NONE',  ( -3.749999999999999556, 13.75000000000000000, -3.499999999999999112 ) ) ;
#5632=CARTESIAN_POINT ( 'NONE',  ( -3.980102097228897245E-16, 0.5000000000000000000, -6.749999999999999112 ) ) ;
#5636=CARTESIAN_POINT ( 'NONE',  ( 2.298097038856279362, 1.375000000000000000, -1.201902961143720860 ) ) ;
#5642=CARTESIAN_POINT ( 'NONE',  ( -1.346194077712558945, 10.56250000000000355, -0.2500000000000002220 ) ) ;
#5644=CARTESIAN_POINT ( 'NONE',  ( 3.750000000000000000, 2.312500000000000000, -1.946699141100892705 ) ) ;
#5650=CARTESIAN_POINT ( 'NONE',  ( -3.249999999999999556, 10.31250000000000000, -4.846194077712557835 ) ) ;
#5657=CARTESIAN_POINT ( 'NONE',  ( -3.750000000000000000, 2.250000000000000444, -3.499999999999999112 ) ) ;
#5658=CARTESIAN_POINT ( 'NONE',  ( 0.000000000000000000, 13.50000000000000355, -0.2500000000000002220 ) ) ;
#5661=CARTESIAN_POINT ( 'NONE',  ( 1.346194077712558057, 14.56250000000000000, -6.750000000000000000 ) ) ;
#5666=CARTESIAN_POINT ( 'NONE',  ( 1.346194077712560944, 2.937500000000000444, -0.2500000000000010547 ) ) ;
#5673=CARTESIAN_POINT ( 'NONE',  ( 1.346194077712558279, 12.56250000000000000, -6.750000000000000000 ) ) ;
#5676=CARTESIAN_POINT ( 'NONE',  ( 0.000000000000000000, 11.50000000000000000, 0.2500000000000002220 ) ) ;
#5678=CARTESIAN_POINT ( 'NONE',  ( -4.592425496802573972E-16, 1.000000000000000000, -7.250000000000000000 ) ) ;
#5679=CARTESIAN_POINT ( 'NONE',  ( -2.298097038856279362, 6.875000000000000000, -5.798097038856278473 ) ) ;
#5680=VERTEX_POINT ( 'NONE', #4218 ) ;
#5683=CARTESIAN_POINT ( 'NONE',  ( 2.298097038856278473, 2.625000000000000000, -5.798097038856279362 ) ) ;
#5685=CARTESIAN_POINT ( 'NONE',  ( 1.553300858899108849, 5.937500000000000000, 0.2499999999999993616 ) ) ;
#5689=VECTOR ( 'NONE', #12079, 1000.000000000000000 ) ;
#5696=CARTESIAN_POINT ( 'NONE',  ( 1.346194077712558279, 9.062500000000003553, -6.750000000000000888 ) ) ;
#5699=CARTESIAN_POINT ( 'NONE',  ( -2.651650429449552870, 8.875000000000000000, -6.151650429449552426 ) ) ;
#5700=CARTESIAN_POINT ( 'NONE',  ( 3.749999999999999112, 14.68750000000000178, -5.053300858899108405 ) ) ;
#5704=CARTESIAN_POINT ( 'NONE',  ( -2.651650429449553314, 13.87500000000000178, -6.151650429449552426 ) ) ;
#5710=PLANE ( 'NONE',  #2094 ) ;
#5711=CARTESIAN_POINT ( 'NONE',  ( 0.000000000000000000, 2.000000000000000000, -0.2500000000000002220 ) ) ;
#5714=CARTESIAN_POINT ( 'NONE',  ( 1.346194077712561166, 1.437500000000000000, -0.2500000000000011102 ) ) ;
#5720=CARTESIAN_POINT ( 'NONE',  ( 3.249999999999998224, 12.18750000000000178, -4.846194077712561388 ) ) ;
#5722=CARTESIAN_POINT ( 'NONE',  ( -0.3766621274091713767, 0.2975415354274087432, -7.146945437571386783 ) ) ;
#5723=CARTESIAN_POINT ( 'NONE',  ( 1.553300858899109516, 0.4375000000000000555, 0.2499999999999993616 ) ) ;
#5729=CARTESIAN_POINT ( 'NONE',  ( 2.298097038856279362, 6.875000000000000000, -1.201902961143720860 ) ) ;
#5731=DIRECTION ( 'NONE',  ( 0.000000000000000000, -1.000000000000000000, 0.000000000000000000 ) ) ;
#5734=ORIENTED_EDGE ( 'NONE', *, *, #7044, .T. ) ;
#5736=CARTESIAN_POINT ( 'NONE',  ( -3.749999999999999556, 6.187500000000000888, -1.946699141100892927 ) ) ;
#5737=CARTESIAN_POINT ( 'NONE',  ( -1.553300858899107073, 1.937500000000000222, -7.249999999999999112 ) ) ;
#5741=CARTESIAN_POINT ( 'NONE',  ( 1.346194077712560944, 14.93750000000000178, -0.2500000000000010547 ) ) ;
#5745=CARTESIAN_POINT ( 'NONE',  ( -3.249999999999999556, 2.187500000000000444, -2.153805922287440833 ) ) ;
#5753=CARTESIAN_POINT ( 'NONE',  ( -1.346194077712558945, 10.06250000000000000, -0.2500000000000002220 ) ) ;
#5756=CARTESIAN_POINT ( 'NONE',  ( 3.749999999999999556, 8.250000000000000000, -3.500000000000000444 ) ) ;
#5758=CARTESIAN_POINT ( 'NONE',  ( 1.553300858899105963, 7.062500000000000888, -7.250000000000000888 ) ) ;
#5759=CARTESIAN_POINT ( 'NONE',  ( -3.249999999999999112, 7.812500000000000000, -4.846194077712558723 ) ) ;
#5762=CARTESIAN_POINT ( 'NONE',  ( 1.346194077712560944, 2.937500000000000444, -0.2500000000000010547 ) ) ;
#5763=CARTESIAN_POINT ( 'NONE',  ( 3.749999999999999112, 7.812500000000000000, -1.946699141100892039 ) ) ;
#5773=CARTESIAN_POINT ( 'NONE',  ( 3.249999999999998224, 8.312500000000003553, -2.153805922287439945 ) ) ;
#5775=CARTESIAN_POINT ( 'NONE',  ( 3.749999999999998668, 10.18750000000000533, -5.053300858899108405 ) ) ;
#5776=CARTESIAN_POINT ( 'NONE',  ( -3.750000000000000000, 12.18750000000000000, -1.946699141100892927 ) ) ;
#5778=CARTESIAN_POINT ( 'NONE',  ( 3.249999999999999112, 11.81249999999999822, -2.153805922287439945 ) ) ;
#5781=CARTESIAN_POINT ( 'NONE',  ( 3.749999999999999112, 14.18750000000000178, -5.053300858899108405 ) ) ;
#5787=CARTESIAN_POINT ( 'NONE',  ( 3.249999999999999112, 4.812500000000000888, -2.153805922287439945 ) ) ;
#5790=CARTESIAN_POINT ( 'NONE',  ( -3.249999999999999112, 2.687500000000000888, -2.153805922287440833 ) ) ;
#5796=CARTESIAN_POINT ( 'NONE',  ( -1.346194077712559167, 13.93750000000000000, -6.749999999999999112 ) ) ;
#5798=CARTESIAN_POINT ( 'NONE',  ( 2.651650429449554203, 2.375000000000000000, -0.8483495705504471296 ) ) ;
#5803=CARTESIAN_POINT ( 'NONE',  ( -3.249999999999999556, 12.18750000000000000, -2.153805922287440833 ) ) ;
#5811=CARTESIAN_POINT ( 'NONE',  ( -1.553300858899106629, 5.062500000000001776, 0.2500000000000002220 ) ) ;
#5812=CARTESIAN_POINT ( 'NONE',  ( -1.553300858899106629, 2.562500000000000444, 0.2499999999999998335 ) ) ;
#5815=CARTESIAN_POINT ( 'NONE',  ( 2.298097038856279362, 13.87500000000000000, -1.201902961143720860 ) ) ;
#5818=CARTESIAN_POINT ( 'NONE',  ( -3.249999999999999556, 5.187500000000001776, -2.153805922287440833 ) ) ;
#5823=CARTESIAN_POINT ( 'NONE',  ( -3.980102097228897245E-16, 10.50000000000000000, -6.749999999999999112 ) ) ;
#5825=ADVANCED_FACE ( 'NONE', ( #1967 ), #10013, .F. ) ;
#5828=CARTESIAN_POINT ( 'NONE',  ( -1.553300858899106629, 7.562500000000000888, 0.2500000000000002220 ) ) ;
#5830=CARTESIAN_POINT ( 'NONE',  ( -3.980102097228897738E-16, 5.000000000000000000, -6.749999999999999112 ) ) ;
#5833=CARTESIAN_POINT ( 'NONE',  ( -3.249999999999999556, 4.187500000000000000, -2.153805922287440833 ) ) ;
#5835=CARTESIAN_POINT ( 'NONE',  ( -3.749999999999999556, 10.31250000000000000, -5.053300858899104853 ) ) ;
#5843=CARTESIAN_POINT ( 'NONE',  ( 2.298097038856279362, 5.375000000000000000, -1.201902961143720860 ) ) ;
#5845=CARTESIAN_POINT ( 'NONE',  ( 0.000000000000000000, 10.50000000000000000, 0.2499999999999998057 ) ) ;
#5849=CARTESIAN_POINT ( 'NONE',  ( -2.651650429449552870, 12.62500000000000000, -0.8483495705504463524 ) ) ;
#5856=CARTESIAN_POINT ( 'NONE',  ( 3.249999999999999112, 2.812500000000000000, -2.153805922287439945 ) ) ;
#5858=CARTESIAN_POINT ( 'NONE',  ( -3.980102097228897738E-16, 8.000000000000000000, -6.749999999999999112 ) ) ;
#5859=ORIENTED_EDGE ( 'NONE', *, *, #10082, .F. ) ;
#5863=CARTESIAN_POINT ( 'NONE',  ( 1.346194077712558057, 1.562500000000000000, -6.750000000000000000 ) ) ;
#5864=CARTESIAN_POINT ( 'NONE',  ( 0.000000000000000000, 11.50000000000000000, -0.2500000000000002220 ) ) ;
#5866=CARTESIAN_POINT ( 'NONE',  ( 2.651650429449552870, 3.125000000000000444, -6.151650429449555091 ) ) ;
#5871=CARTESIAN_POINT ( 'NONE',  ( 3.249999999999999556, 11.75000000000000000, -3.500000000000000000 ) ) ;
#5878=CARTESIAN_POINT ( 'NONE',  ( -4.592425496802573972E-16, 6.500000000000000888, -7.249999999999999112 ) ) ;
#5879=CARTESIAN_POINT ( 'NONE',  ( -2.651650429449552870, 3.875000000000000444, -6.151650429449552426 ) ) ;
#5883=CARTESIAN_POINT ( 'NONE',  ( 2.298097038856279362, 2.375000000000000000, -1.201902961143720860 ) ) ;
#5887=CARTESIAN_POINT ( 'NONE',  ( -3.980102097228897245E-16, 5.500000000000000000, -6.749999999999999112 ) ) ;
#5896=CARTESIAN_POINT ( 'NONE',  ( -0.3766621274091715987, 0.5000000000000000000, -0.1347136637304948981 ) ) ;
#5897=CARTESIAN_POINT ( 'NONE',  ( 3.749999999999999112, 5.187500000000001776, -5.053300858899108405 ) ) ;
#5898=CARTESIAN_POINT ( 'NONE',  ( -3.249999999999999556, 5.750000000000000888, -3.500000000000000000 ) ) ;
#5901=CARTESIAN_POINT ( 'NONE',  ( -3.249999999999999556, 1.250000000000000000, -3.499999999999999556 ) ) ;
#5916=CARTESIAN_POINT ( 'NONE',  ( -3.749999999999999556, 12.75000000000000178, -3.499999999999999112 ) ) ;
#5921=CARTESIAN_POINT ( 'NONE',  ( 1.346194077712558279, 3.062500000000000000, -6.750000000000000888 ) ) ;
#5930=CARTESIAN_POINT ( 'NONE',  ( -3.249999999999999556, 2.187500000000000444, -2.153805922287440833 ) ) ;
#5934=CARTESIAN_POINT ( 'NONE',  ( 1.346194077712561166, 6.437500000000000888, -0.2500000000000011102 ) ) ;
#5940=CARTESIAN_POINT ( 'NONE',  ( -3.249999999999999556, 1.312500000000000444, -4.846194077712557835 ) ) ;
#5941=CARTESIAN_POINT ( 'NONE',  ( -1.346194077712559167, 14.93750000000000000, -6.749999999999999112 ) ) ;
#5942=CARTESIAN_POINT ( 'NONE',  ( -3.750000000000000000, 7.250000000000000000, -3.499999999999999112 ) ) ;
#5944=CARTESIAN_POINT ( 'NONE',  ( 3.749999999999999112, 4.187500000000000888, -5.053300858899108405 ) ) ;
#5950=CARTESIAN_POINT ( 'NONE',  ( 1.346194077712558057, 12.56250000000000000, -6.750000000000000000 ) ) ;
#5958=CARTESIAN_POINT ( 'NONE',  ( -2.651650429449552870, 6.125000000000000000, -0.8483495705504462414 ) ) ;
#5959=CARTESIAN_POINT ( 'NONE',  ( 1.553300858899105963, 6.062500000000000000, -7.249999999999999112 ) ) ;
#5961=VERTEX_POINT ( 'NONE', #13779 ) ;
#5964=CARTESIAN_POINT ( 'NONE',  ( 1.346194077712561166, 1.437500000000000000, -0.2500000000000011102 ) ) ;
#5966=CARTESIAN_POINT ( 'NONE',  ( 0.000000000000000000, 0.2006112523677016646, 0.1491815183709511716 ) ) ;
#5968=CARTESIAN_POINT ( 'NONE',  ( 1.346194077712560944, 3.937500000000000000, -0.2500000000000010547 ) ) ;
#5974=CARTESIAN_POINT ( 'NONE',  ( -3.249999999999999556, 13.31250000000000000, -4.846194077712557835 ) ) ;
#5978=CARTESIAN_POINT ( 'NONE',  ( -4.592425496802573972E-16, 4.000000000000000888, -7.250000000000000000 ) ) ;
#5979=CARTESIAN_POINT ( 'NONE',  ( -3.980102097228897738E-16, 10.00000000000000000, -6.749999999999999112 ) ) ;
#5983=CARTESIAN_POINT ( 'NONE',  ( -3.249999999999999556, 4.312500000000000888, -4.846194077712557835 ) ) ;
#5995=CARTESIAN_POINT ( 'NONE',  ( 2.651650429449552870, 14.12500000000000000, -6.151650429449553314 ) ) ;
#5998=CARTESIAN_POINT ( 'NONE',  ( 0.000000000000000000, 3.500000000000000000, -0.2500000000000002220 ) ) ;
#6003=CARTESIAN_POINT ( 'NONE',  ( 0.3766621274091715987, 0.5000000000000000000, -7.146945437571387671 ) ) ;
#6007=CARTESIAN_POINT ( 'NONE',  ( 3.249999999999999556, 3.750000000000000000, -3.500000000000000000 ) ) ;
#6010=CARTESIAN_POINT ( 'NONE',  ( -3.249999999999999112, 7.687500000000000888, -2.153805922287440833 ) ) ;
#6017=CARTESIAN_POINT ( 'NONE',  ( -1.346194077712559389, 2.437500000000000444, -6.749999999999999112 ) ) ;
#6019=CARTESIAN_POINT ( 'NONE',  ( -2.651650429449552870, 2.875000000000000000, -6.151650429449552426 ) ) ;
#6020=CARTESIAN_POINT ( 'NONE',  ( 1.553300858899108849, 5.937500000000000000, 0.2499999999999993616 ) ) ;
#6022=CARTESIAN_POINT ( 'NONE',  ( 1.553300858899105963, 8.062500000000001776, -7.250000000000000888 ) ) ;
#6027=CARTESIAN_POINT ( 'NONE',  ( 1.346194077712560944, 13.93750000000000000, -0.2500000000000010547 ) ) ;
#6032=ORIENTED_EDGE ( 'NONE', *, *, #14541, .T. ) ;
#6033=CARTESIAN_POINT ( 'NONE',  ( -3.750000000000000000, 8.812500000000001776, -5.053300858899105741 ) ) ;
#6037=CARTESIAN_POINT ( 'NONE',  ( 3.750000000000000000, 5.750000000000000000, -3.500000000000000444 ) ) ;
#6038=CARTESIAN_POINT ( 'NONE',  ( -1.553300858899107073, 4.937500000000000000, -7.249999999999999112 ) ) ;
#6042=CARTESIAN_POINT ( 'NONE',  ( 3.249999999999999556, 6.250000000000000000, -3.500000000000000000 ) ) ;
#6046=CARTESIAN_POINT ( 'NONE',  ( 1.346194077712558057, 9.562500000000000000, -6.750000000000000000 ) ) ;
#6051=ORIENTED_EDGE ( 'NONE', *, *, #12707, .F. ) ;
#6052=FACE_OUTER_BOUND ( 'NONE', #143, .T. ) ;
#6053=CARTESIAN_POINT ( 'NONE',  ( 3.249999999999999112, 13.81250000000000000, -2.153805922287439945 ) ) ;
#6055=ORIENTED_EDGE ( 'NONE', *, *, #7781, .T. ) ;
#6056=CARTESIAN_POINT ( 'NONE',  ( -0.2511109529196363654, 0.2068841402060896395, 0.1491815183709511161 ) ) ;
#6058=CARTESIAN_POINT ( 'NONE',  ( -4.592425496802573972E-16, 7.000000000000000000, -7.250000000000000000 ) ) ;
#6059=CARTESIAN_POINT ( 'NONE',  ( 1.346194077712561166, 12.43750000000000000, -0.2500000000000011102 ) ) ;
#6060=VERTEX_POINT ( 'NONE', #2027 ) ;
#6062=CARTESIAN_POINT ( 'NONE',  ( -3.980102097228897245E-16, 5.500000000000000000, -6.749999999999999112 ) ) ;
#6070=CARTESIAN_POINT ( 'NONE',  ( 2.298097038856278473, 9.625000000000000000, -5.798097038856279362 ) ) ;
#6071=CARTESIAN_POINT ( 'NONE',  ( 2.298097038856279362, 13.37500000000000000, -1.201902961143720860 ) ) ;
#6074=CARTESIAN_POINT ( 'NONE',  ( -3.749999999999999556, 13.75000000000000000, -3.499999999999999112 ) ) ;
#6077=CARTESIAN_POINT ( 'NONE',  ( 3.249999999999999556, 4.250000000000000000, -3.500000000000000000 ) ) ;
#6085=CARTESIAN_POINT ( 'NONE',  ( -1.346194077712558945, 8.062500000000000000, -0.2500000000000002220 ) ) ;
#6087=CARTESIAN_POINT ( 'NONE',  ( 0.000000000000000000, 12.00000000000000000, -0.2500000000000002220 ) ) ;
#6088=CARTESIAN_POINT ( 'NONE',  ( -2.298097038856279362, 6.875000000000000000, -5.798097038856278473 ) ) ;
#6091=CARTESIAN_POINT ( 'NONE',  ( -0.3766621274091715432, -0.2054769798019681903, -0.1347136637304948981 ) ) ;
#6094=CARTESIAN_POINT ( 'NONE',  ( 1.346194077712558057, 0.5625000000000001110, -6.750000000000000000 ) ) ;
#6095=CARTESIAN_POINT ( 'NONE',  ( -2.651650429449552870, 1.625000000000000000, -0.8483495705504467965 ) ) ;
#6096=CARTESIAN_POINT ( 'NONE',  ( -2.651650429449553314, 6.375000000000000888, -6.151650429449552426 ) ) ;
#6098=CARTESIAN_POINT ( 'NONE',  ( 2.651650429449552870, 6.125000000000000000, -6.151650429449555091 ) ) ;
#6106=CARTESIAN_POINT ( 'NONE',  ( 3.249999999999999112, 10.81250000000000178, -2.153805922287439945 ) ) ;
#6109=ORIENTED_EDGE ( 'NONE', *, *, #367, .F. ) ;
#6111=CARTESIAN_POINT ( 'NONE',  ( -4.592425496802573972E-16, 8.999999999999998224, -7.250000000000000000 ) ) ;
#6115=CARTESIAN_POINT ( 'NONE',  ( -1.553300858899107295, 7.437500000000000888, -7.250000000000000000 ) ) ;
#6116=CARTESIAN_POINT ( 'NONE',  ( -3.750000000000000000, 4.687500000000000000, -1.946699141100893149 ) ) ;
#6119=CARTESIAN_POINT ( 'NONE',  ( -3.249999999999999556, 2.750000000000000444, -3.500000000000000000 ) ) ;
#6121=CARTESIAN_POINT ( 'NONE',  ( -3.749999999999999556, 8.312500000000000000, -5.053300858899104853 ) ) ;
#6125=CARTESIAN_POINT ( 'NONE',  ( -1.346194077712559389, 6.062500000000000000, -0.2500000000000002220 ) ) ;
#6131=VERTEX_POINT ( 'NONE', #13935 ) ;
#6132=DIRECTION ( 'NONE',  ( 0.000000000000000000, 0.000000000000000000, -1.000000000000000000 ) ) ;
#6137=CARTESIAN_POINT ( 'NONE',  ( 2.651650429449553314, 14.37500000000000000, -0.8483495705504476847 ) ) ;
#6138=CARTESIAN_POINT ( 'NONE',  ( -3.249999999999999556, 7.750000000000000888, -3.500000000000000000 ) ) ;
#6139=CARTESIAN_POINT ( 'NONE',  ( -1.346194077712559167, 9.937500000000001776, -6.749999999999999112 ) ) ;
#6142=CARTESIAN_POINT ( 'NONE',  ( -2.298097038856278473, 7.125000000000000000, -1.201902961143720416 ) ) ;
#6143=DIRECTION ( 'NONE',  ( -0.000000000000000000, -0.000000000000000000, 1.000000000000000000 ) ) ;
#6149=CARTESIAN_POINT ( 'NONE',  ( 2.298097038856278473, 1.625000000000000222, -5.798097038856279362 ) ) ;
#6151=CARTESIAN_POINT ( 'NONE',  ( 2.651650429449553314, 15.37500000000000178, -0.8483495705504476847 ) ) ;
#6154=CARTESIAN_POINT ( 'NONE',  ( -1.346194077712558945, 3.562500000000000888, -0.2500000000000002220 ) ) ;
#6163=CARTESIAN_POINT ( 'NONE',  ( 2.298097038856279362, 5.875000000000000000, -1.201902961143720860 ) ) ;
#6165=CARTESIAN_POINT ( 'NONE',  ( -3.980102097228897738E-16, 1.000000000000000000, -6.749999999999999112 ) ) ;
#6167=CARTESIAN_POINT ( 'NONE',  ( 3.249999999999998224, 6.187500000000001776, -4.846194077712561388 ) ) ;
#6174=CARTESIAN_POINT ( 'NONE',  ( -2.298097038856278918, 3.375000000000000000, -5.798097038856277585 ) ) ;
#6175=CARTESIAN_POINT ( 'NONE',  ( 2.298097038856278029, 15.12500000000000000, -5.798097038856279362 ) ) ;
#6177=CARTESIAN_POINT ( 'NONE',  ( 2.651650429449553759, 6.875000000000000000, -0.8483495705504471296 ) ) ;
#6179=CARTESIAN_POINT ( 'NONE',  ( 3.749999999999999556, 6.250000000000000888, -3.500000000000000444 ) ) ;
#6190=CARTESIAN_POINT ( 'NONE',  ( 0.3766621274091721538, 0.2615998065109338411, -7.070313984750484337 ) ) ;
#6191=ORIENTED_EDGE ( 'NONE', *, *, #8081, .F. ) ;
#6192=CARTESIAN_POINT ( 'NONE',  ( 3.749999999999999112, 8.187500000000000000, -5.053300858899108405 ) ) ;
#6196=CARTESIAN_POINT ( 'NONE',  ( 1.553300858899108849, 8.937500000000001776, 0.2499999999999993616 ) ) ;
#6197=CARTESIAN_POINT ( 'NONE',  ( 2.651650429449553314, 7.375000000000000000, -0.8483495705504476847 ) ) ;
#6201=CARTESIAN_POINT ( 'NONE',  ( 3.249999999999998224, 4.312500000000000000, -2.153805922287439945 ) ) ;
#6204=CARTESIAN_POINT ( 'NONE',  ( -4.592425496802573972E-16, 11.50000000000000000, -7.249999999999999112 ) ) ;
#6208=CARTESIAN_POINT ( 'NONE',  ( -1.346194077712559389, 6.437500000000000888, -6.749999999999999112 ) ) ;
#6215=CARTESIAN_POINT ( 'NONE',  ( 3.249999999999999112, 14.81250000000000178, -2.153805922287439945 ) ) ;
#6220=CARTESIAN_POINT ( 'NONE',  ( 2.651650429449553314, 11.37500000000000178, -0.8483495705504476847 ) ) ;
#6221=CARTESIAN_POINT ( 'NONE',  ( 3.249999999999998224, 11.31250000000000355, -2.153805922287439945 ) ) ;
#6222=CARTESIAN_POINT ( 'NONE',  ( 3.249999999999998224, 10.31250000000000000, -2.153805922287439945 ) ) ;
#6225=CARTESIAN_POINT ( 'NONE',  ( -3.249999999999999556, 6.312500000000000888, -4.846194077712557835 ) ) ;
#6231=LINE ( 'NONE', #5075, #6702 ) ;
#6235=CARTESIAN_POINT ( 'NONE',  ( -3.980102097228897245E-16, 2.500000000000000000, -6.749999999999999112 ) ) ;
#6236=CARTESIAN_POINT ( 'NONE',  ( 3.749999999999998668, 13.68750000000000000, -5.053300858899107517 ) ) ;
#6238=CARTESIAN_POINT ( 'NONE',  ( 2.651650429449552870, 12.12500000000000000, -6.151650429449553314 ) ) ;
#6242=CARTESIAN_POINT ( 'NONE',  ( 3.249999999999999556, 8.750000000000000000, -3.500000000000000000 ) ) ;
#6250=CARTESIAN_POINT ( 'NONE',  ( -2.298097038856278473, 5.125000000000000000, -1.201902961143720416 ) ) ;
#6253=CARTESIAN_POINT ( 'NONE',  ( -1.346194077712559389, 12.43750000000000000, -6.749999999999999112 ) ) ;
#6254=CARTESIAN_POINT ( 'NONE',  ( -3.249999999999999112, 10.81250000000000000, -4.846194077712558723 ) ) ;
#6256=CARTESIAN_POINT ( 'NONE',  ( -2.298097038856278473, 0.1250000000000000000, -1.201902961143720416 ) ) ;
#6258=CARTESIAN_POINT ( 'NONE',  ( 3.249999999999999112, 5.812500000000000000, -2.153805922287439945 ) ) ;
#6259=CARTESIAN_POINT ( 'NONE',  ( 0.000000000000000000, 1.500000000000000222, 0.2499999999999998057 ) ) ;
#6260=CARTESIAN_POINT ( 'NONE',  ( 1.553300858899108849, 3.937500000000000000, 0.2499999999999993616 ) ) ;
#6262=CARTESIAN_POINT ( 'NONE',  ( -1.553300858899107073, 6.937500000000001776, -7.249999999999999112 ) ) ;
#6273=CARTESIAN_POINT ( 'NONE',  ( -4.592425496802573972E-16, 14.00000000000000000, -7.250000000000000000 ) ) ;
#6275=FACE_OUTER_BOUND ( 'NONE', #14362, .T. ) ;
#6277=CARTESIAN_POINT ( 'NONE',  ( 0.000000000000000000, 11.00000000000000000, 0.2500000000000002220 ) ) ;
#6279=CARTESIAN_POINT ( 'NONE',  ( 3.749999999999999112, 9.312500000000001776, -1.946699141100893149 ) ) ;
#6281=ORIENTED_EDGE ( 'NONE', *, *, #2808, .F. ) ;
#6282=CARTESIAN_POINT ( 'NONE',  ( -3.249999999999999556, 4.750000000000000000, -3.500000000000000000 ) ) ;
#6283=CARTESIAN_POINT ( 'NONE',  ( -1.553300858899106629, 9.062499999999998224, 0.2500000000000002220 ) ) ;
#6286=CARTESIAN_POINT ( 'NONE',  ( -1.346194077712559389, 8.437500000000000000, -6.749999999999999112 ) ) ;
#6290=EDGE_CURVE ( 'NONE', #5680, #11692, #2067, .T. ) ;
#6298=CARTESIAN_POINT ( 'NONE',  ( 2.651650429449552870, 13.12500000000000178, -6.151650429449553314 ) ) ;
#6299=CARTESIAN_POINT ( 'NONE',  ( -3.980102097228897738E-16, 12.00000000000000178, -6.749999999999999112 ) ) ;
#6300=CARTESIAN_POINT ( 'NONE',  ( 3.249999999999998224, 12.18750000000000178, -4.846194077712561388 ) ) ;
#6303=CARTESIAN_POINT ( 'NONE',  ( -2.298097038856278473, 8.125000000000000000, -1.201902961143720416 ) ) ;
#6315=CARTESIAN_POINT ( 'NONE',  ( -2.298097038856278473, 0.1250000000000000000, -1.201902961143720416 ) ) ;
#6316=CARTESIAN_POINT ( 'NONE',  ( 0.000000000000000000, 14.00000000000000000, 0.2500000000000002220 ) ) ;
#6317=ORIENTED_EDGE ( 'NONE', *, *, #2197, .F. ) ;
#6318=LINE ( 'NONE', #1526, #9205 ) ;
#6319=CARTESIAN_POINT ( 'NONE',  ( 3.749999999999998668, 2.687500000000000888, -5.053300858899107517 ) ) ;
#6328=CARTESIAN_POINT ( 'NONE',  ( -2.298097038856278473, 7.125000000000000000, -1.201902961143720416 ) ) ;
#6330=CARTESIAN_POINT ( 'NONE',  ( -1.346194077712559389, 13.43749999999999822, -6.749999999999999112 ) ) ;
#6331=CARTESIAN_POINT ( 'NONE',  ( 1.346194077712558279, 12.06250000000000000, -6.750000000000000888 ) ) ;
#6336=CARTESIAN_POINT ( 'NONE',  ( 2.298097038856279362, 3.875000000000000000, -1.201902961143720860 ) ) ;
#6337=CARTESIAN_POINT ( 'NONE',  ( 1.553300858899105963, 7.062499999999999112, -7.249999999999999112 ) ) ;
#6338=CARTESIAN_POINT ( 'NONE',  ( 1.553300858899105963, 7.562500000000000000, -7.250000000000000000 ) ) ;
#6340=CARTESIAN_POINT ( 'NONE',  ( 3.750000000000000000, 6.312500000000000000, -1.946699141100892705 ) ) ;
#6349=CARTESIAN_POINT ( 'NONE',  ( 2.651650429449552870, 12.12500000000000000, -6.151650429449555091 ) ) ;
#6353=CARTESIAN_POINT ( 'NONE',  ( -2.651650429449553314, 9.375000000000000000, -6.151650429449552426 ) ) ;
#6354=CARTESIAN_POINT ( 'NONE',  ( -3.750000000000000000, 8.812500000000001776, -5.053300858899105741 ) ) ;
#6358=CARTESIAN_POINT ( 'NONE',  ( 2.298097038856279362, 7.375000000000000000, -1.201902961143720860 ) ) ;
#6359=CARTESIAN_POINT ( 'NONE',  ( 2.651650429449552870, 9.625000000000000000, -6.151650429449554203 ) ) ;
#6362=CARTESIAN_POINT ( 'NONE',  ( 3.249999999999999112, 8.812500000000000000, -2.153805922287439945 ) ) ;
#6371=CARTESIAN_POINT ( 'NONE',  ( -1.553300858899107073, 10.93750000000000355, -7.249999999999999112 ) ) ;
#6372=CARTESIAN_POINT ( 'NONE',  ( -1.346194077712559167, 10.93750000000000355, -6.749999999999999112 ) ) ;
#6373=CARTESIAN_POINT ( 'NONE',  ( 2.298097038856279362, 14.37500000000000000, -1.201902961143720860 ) ) ;
#6375=CARTESIAN_POINT ( 'NONE',  ( -3.249999999999999556, 7.312500000000000888, -4.846194077712557835 ) ) ;
#6384=CARTESIAN_POINT ( 'NONE',  ( 0.000000000000000000, 9.000000000000001776, -0.2500000000000002220 ) ) ;
#6385=CARTESIAN_POINT ( 'NONE',  ( -3.249999999999999556, 13.75000000000000000, -3.500000000000000000 ) ) ;
#6386=CARTESIAN_POINT ( 'NONE',  ( -3.749999999999999556, -0.2499999999999998890, -3.499999999999999112 ) ) ;
#6389=CARTESIAN_POINT ( 'NONE',  ( 1.553300858899105963, 1.562500000000000000, -7.250000000000000888 ) ) ;
#6393=CARTESIAN_POINT ( 'NONE',  ( -2.651650429449553314, 2.375000000000000000, -6.151650429449552426 ) ) ;
#6395=CARTESIAN_POINT ( 'NONE',  ( 0.3766621274091715987, -0.2500000000000000000, -0.1347136637304948981 ) ) ;
#6398=CARTESIAN_POINT ( 'NONE',  ( 0.000000000000000000, 7.000000000000000000, -0.2500000000000002220 ) ) ;
#6399=PLANE ( 'NONE',  #11851 ) ;
#6400=CARTESIAN_POINT ( 'NONE',  ( -1.346194077712559389, 14.43750000000000000, -6.749999999999999112 ) ) ;
#6401=CARTESIAN_POINT ( 'NONE',  ( 3.249999999999998224, 9.312500000000000000, -2.153805922287439945 ) ) ;
#6404=CARTESIAN_POINT ( 'NONE',  ( -2.298097038856278918, 6.375000000000000888, -5.798097038856277585 ) ) ;
#6405=CARTESIAN_POINT ( 'NONE',  ( -1.553300858899107073, 5.937500000000000000, -7.249999999999999112 ) ) ;
#6407=CARTESIAN_POINT ( 'NONE',  ( 0.000000000000000000, 11.00000000000000000, 0.2500000000000002220 ) ) ;
#6411=CARTESIAN_POINT ( 'NONE',  ( -3.750000000000000000, 10.68750000000000178, -1.946699141100893149 ) ) ;
#6420=CARTESIAN_POINT ( 'NONE',  ( 1.553300858899105963, 13.06249999999999822, -7.250000000000000888 ) ) ;
#6424=CARTESIAN_POINT ( 'NONE',  ( 3.749999999999999112, 7.812500000000000000, -1.946699141100892039 ) ) ;
#6425=CARTESIAN_POINT ( 'NONE',  ( 3.749999999999998668, 10.18750000000000533, -5.053300858899108405 ) ) ;
#6428=CARTESIAN_POINT ( 'NONE',  ( 3.249999999999999556, 9.250000000000001776, -3.500000000000000000 ) ) ;
#6429=CARTESIAN_POINT ( 'NONE',  ( -3.750000000000000000, -0.3124999999999999445, -1.946699141100893149 ) ) ;
#6434=CARTESIAN_POINT ( 'NONE',  ( -1.346194077712559389, 13.43749999999999822, -6.749999999999999112 ) ) ;
#6445=CARTESIAN_POINT ( 'NONE',  ( -3.749999999999999556, 13.75000000000000000, -3.499999999999999112 ) ) ;
#6446=CARTESIAN_POINT ( 'NONE',  ( -3.980102097228897738E-16, 11.00000000000000178, -6.749999999999999112 ) ) ;
#6447=CARTESIAN_POINT ( 'NONE',  ( -3.249999999999999112, 12.68750000000000000, -2.153805922287440833 ) ) ;
#6448=ORIENTED_EDGE ( 'NONE', *, *, #10082, .T. ) ;
#6450=CARTESIAN_POINT ( 'NONE',  ( 3.249999999999999556, 9.750000000000000000, -3.500000000000000000 ) ) ;
#6459=CARTESIAN_POINT ( 'NONE',  ( 3.249999999999999112, 3.812500000000000000, -2.153805922287439945 ) ) ;
#6460=CARTESIAN_POINT ( 'NONE',  ( -1.553300858899107295, 13.43749999999999822, -7.250000000000000000 ) ) ;
#6465=CARTESIAN_POINT ( 'NONE',  ( -1.553300858899106629, 1.062500000000000222, 0.2500000000000002220 ) ) ;
#6468=CARTESIAN_POINT ( 'NONE',  ( 0.000000000000000000, 3.061616997868383018E-17, 0.2500000000000002220 ) ) ;
#6470=FACE_OUTER_BOUND ( 'NONE', #4072, .T. ) ;
#6475=CARTESIAN_POINT ( 'NONE',  ( 2.298097038856279362, 10.87500000000000178, -1.201902961143720860 ) ) ;
#6478=CARTESIAN_POINT ( 'NONE',  ( 1.346194077712561166, 2.437500000000000444, -0.2500000000000011102 ) ) ;
#6479=CARTESIAN_POINT ( 'NONE',  ( 2.298097038856279362, 12.37500000000000178, -1.201902961143720860 ) ) ;
#6483=CARTESIAN_POINT ( 'NONE',  ( 3.249999999999999556, 3.750000000000000000, -3.500000000000000000 ) ) ;
#6484=CARTESIAN_POINT ( 'NONE',  ( -2.651650429449552870, 6.625000000000000000, -0.8483495705504467965 ) ) ;
#6485=CARTESIAN_POINT ( 'NONE',  ( -2.651650429449553314, 11.37500000000000000, -6.151650429449552426 ) ) ;
#6488=CARTESIAN_POINT ( 'NONE',  ( -2.651650429449553314, 8.874999999999996447, -6.151650429449552426 ) ) ;
#6502=CARTESIAN_POINT ( 'NONE',  ( 1.553300858899109516, 13.43750000000000178, 0.2499999999999993616 ) ) ;
#6506=CARTESIAN_POINT ( 'NONE',  ( -3.750000000000000000, 6.687500000000000888, -1.946699141100893149 ) ) ;
#6508=CARTESIAN_POINT ( 'NONE',  ( 2.298097038856278029, 8.125000000000000000, -5.798097038856279362 ) ) ;
#6511=CARTESIAN_POINT ( 'NONE',  ( -3.749999999999999556, 12.31250000000000000, -5.053300858899104853 ) ) ;
#6515=CARTESIAN_POINT ( 'NONE',  ( -3.249999999999999556, 12.31250000000000000, -4.846194077712557835 ) ) ;
#6526=CARTESIAN_POINT ( 'NONE',  ( 2.651650429449552870, 15.12500000000000000, -6.151650429449553314 ) ) ;
#6527=CARTESIAN_POINT ( 'NONE',  ( 3.249999999999998224, 10.18750000000000533, -4.846194077712561388 ) ) ;
#6529=CARTESIAN_POINT ( 'NONE',  ( 1.346194077712561166, 13.43750000000000178, -0.2500000000000011102 ) ) ;
#6531=CARTESIAN_POINT ( 'NONE',  ( -3.249999999999999556, 10.31250000000000000, -4.846194077712557835 ) ) ;
#6540=CARTESIAN_POINT ( 'NONE',  ( -3.249999999999999556, 6.250000000000000000, -3.499999999999999556 ) ) ;
#6542=CARTESIAN_POINT ( 'NONE',  ( -2.651650429449553314, 1.874999999999999778, -6.151650429449552426 ) ) ;
#6546=CARTESIAN_POINT ( 'NONE',  ( -1.553300858899107295, 0.4375000000000000555, -7.250000000000000000 ) ) ;
#6549=CARTESIAN_POINT ( 'NONE',  ( 2.651650429449552870, 1.625000000000000222, -6.151650429449554203 ) ) ;
#6555=CARTESIAN_POINT ( 'NONE',  ( -2.298097038856279362, 2.875000000000000000, -5.798097038856278473 ) ) ;
#6556=CARTESIAN_POINT ( 'NONE',  ( -2.298097038856279362, 12.87500000000000000, -5.798097038856278473 ) ) ;
#6558=( BOUNDED_SURFACE ( )  B_SPLINE_SURFACE ( 3, 2, ( 
 ( #753, #3297, #6256, #6700, #10972, #4383, #14545, #3941, #13812, #3212, #7931, #12650, #6776, #8642, #11491, #908, #5176, #15287, #12804, #11637, #5901, #2209, #6917, #8151, #4610, #3368, #14120, #14273, #12880, #10485, #2141, #9472, #10409, #15220, #6996, #3521, #4536, #14199, #10705, #3672, #12730, #3602, #5683, #1199, #13031, #10624, #11854, #5762, #8229, #6845, #2366, #1055, #4835, #9320, #11783, #8303, #9249, #122, #14042, #12959, #3440, #2292, #11712, #1130, #11559, #7063, #7131, #5833, #10554, #5983, #975, #4679, #9393, #47, #4757, #2438, #15141, #1278, #13973, #8079, #9547, #9705, #277, #197, #14353, #3835, #4991, #10942, #6062, #7297, #14438, #10780, #5071, #12010, #1359, #8458, #9784, #9619, #1593, #3752, #12089, #6225, #12253, #1436, #8536, #1663, #5227, #7458, #2674, #11020, #2598, #437, #8376, #358, #6142, #10856, #506, #6375, #11088, #13269, #9934, #7374, #8612, #4907, #14516, #14670, #13189, #12174, #3915, #1514, #6303, #13346, #2756, #5145, #8696, #2520, #13105, #2835, #9856, #7216, #11935, #14589, #3993, #13431, #7536, #12320, #736, #2903, #12478, #10305, #12632, #588, #10012, #14896, #14972, #7606, #6450, #5440, #5300, #2044, #4366, #11244, #6606, #2975, #13795, #6531, #7686, #1819, #10161, #6756, #4293, #11395, #14819, #8997, #10085, #889, #663, #12398, #14747, #5369, #4216, #8922, #13573, #13725, #13650, #3124, #3052, #4147, #3193, #7838, #11468, #12552, #5590, #7763, #8775, #1895, #1964, #7906, #8845, #11315, #9075, #6679, #815, #5517, #10239, #4073, #11166, #13507, #1737, #8131, #3273, #3583, #1035, #15043, #4739, #9453, #14179, #10535, #1111, #4436, #13013, #6977, #5815, #11693, #10460, #3419, #15121, #14098, #3502, #4514, #15268, #956, #8209, #5661, #12858, #6895, #2416, #7986, #8283, #5741, #9147 ),
 ( #7112, #13874, #11833, #4659, #4590, #12706, #24, #2120, #9223, #7046, #8059, #2272, #9368, #11615, #1258, #5964, #12940, #6825, #15198, #11541, #10383, #2348, #9297, #11761, #14022, #12784, #13951, #3348, #1181, #2191, #5883, #10603, #9599, #3891, #178, #4887, #6119, #2578, #1339, #12068, #12232, #10832, #8435, #103, #7432, #8354, #13168, #4966, #1487, #2497, #12151, #8673, #1643, #10685, #1569, #3652, #14494, #10996, #8591, #9836, #3729, #6201, #4816, #335, #14327, #2811, #7278, #9764, #6282, #7194, #13406, #11991, #10918, #1414, #251, #9682, #14413, #9529, #5049, #5121, #3812, #8515, #3968, #14250, #13249, #2653, #7355, #13324, #2729, #13082, #413, #11914, #6042, #14568, #7513, #10761, #13485, #12301, #1798, #2953, #8901, #4047, #5278, #13553, #8754, #3032, #9988, #14649, #14726, #7742, #6358, #11294, #11148, #13777, #7662, #5420, #1945, #2884, #4348, #567, #12459, #12377, #6508, #11224, #8826, #11070, #1877, #794, #642, #4125, #14953, #9916, #14800, #13631, #5348, #715, #10064, #7584, #8977, #1714, #6428, #4273, #4194, #6583, #10138, #14876, #13707, #3106, #7817, #12529, #6658, #11371, #5498, #10219, #9055, #3172, #7885, #12609, #487, #5202, #3251, #5642, #939, #3480, #10516, #9351, #8189, #6878, #6734, #14004, #4570, #3330, #11593, #6954, #3402, #3557, #5864, #869, #4720, #9279, #1012, #11447, #2329, #5572, #11523, #14076, #10358, #5720, #8111, #13932, #9431, #14157, #10440, #8263, #2174, #10287, #10583, #12838, #8039, #15251, #9202, #15099, #760, #7028, #1090, #13853, #2251, #2100, #4494, #4642, #6807, #12765, #15177, #11672, #7963, #5796, #2024, #12915, #11741, #15023, #1161, #4414, #9123, #12685, #3787, #4793, #9744, #10976, #3944, #12992, #3868, #5941, #1464, #13302, #6175, #12130, #8570, #10664, #10895, #2705, #311 ),
 ( #4864, #12043, #7405, #9506, #393, #7170, #14388, #9576, #14303, #13144, #155, #2396, #8494, #1546, #3703, #11890, #6259, #1232, #6095, #4941, #8412, #7332, #2554, #80, #5025, #14230, #3632, #14472, #7255, #11972, #8334, #13059, #1392, #10810, #226, #2473, #1313, #9657, #6019, #13225, #10740, #2630, #5102, #9816, #14549, #7092, #11813, #12284, #7565, #10114, #1856, #695, #14855, #13536, #13382, #5329, #11201, #9965, #2935, #13611, #10041, #10197, #12506, #7490, #11344, #623, #7639, #2788, #8953, #12209, #2866, #5400, #1694, #12355, #14778, #5255, #772, #5479, #1775, #14930, #8806, #1624, #1925, #4175, #14705, #6561, #542, #6405, #6637, #13685, #7720, #5180, #8879, #8730, #11124, #11274, #13463, #4105, #6484, #3013, #14628, #12434, #8646, #4253, #3082, #6337, #7796, #11051, #467, #9890, #4025, #11425, #1068, #2305, #10564, #4327, #15231, #13912, #988, #2155, #2223, #3229, #13984, #7942, #8091, #9030, #7864, #8167, #5620, #13755, #9334, #14055, #3455, #15154, #5699, #3150, #7007, #11571, #10419, #4551, #15074, #8019, #4395, #3380, #12817, #6859, #12895, #12662, #10334, #11722, #1142, #6933, #3310, #11650, #13825, #5775, #12583, #9259, #2078, #6790, #5845, #1999, #6712, #919, #847, #4471, #10498, #5549, #4622, #10265, #14997, #9103, #11503, #9181, #12744, #11869, #12971, #1208, #291, #9409, #3848, #9722, #9483, #4693, #14134, #14369, #6238, #10718, #10791, #8242, #11946, #3534, #8390, #15300, #8547, #11793, #5916, #206, #10871, #2375, #7073, #1370, #10641, #13283, #5005, #7145, #2531, #14207, #14453, #2450, #3610, #13040, #6074, #2685, #4919, #7309, #131, #9634, #5995, #12106, #1291, #8314, #59, #4842, #9555, #14280, #3680, #3767, #13122, #8472, #7232, #4768, #7384, #13204, #1527, #2609, #12024, #1445, #6151, #8709, #14762 ),
 ( #12336, #10957, #607, #450, #3068, #2850, #10026, #6546, #2768, #8940, #5159, #1756, #7550, #12268, #11102, #13446, #376, #6465, #5385, #1676, #9872, #4235, #14528, #4087, #2919, #6389, #5314, #523, #3926, #13591, #12189, #13362, #8863, #5238, #9947, #7471, #1607, #14686, #8790, #13521, #8624, #14607, #7620, #6319, #11180, #4008, #11033, #4161, #2994, #7702, #12414, #1838, #11258, #680, #10100, #14837, #13668, #7780, #12495, #5084, #1912, #9797, #7932, #909, #11560, #3298, #8154, #10488, #5464, #9321, #13901, #11492, #11332, #6919, #10181, #831, #13974, #14987, #10324, #8008, #3214, #14044, #3441, #15063, #12882, #6777, #14915, #15221, #12732, #12652, #15144, #13813, #4384, #4611, #11640, #5685, #3139, #9171, #6701, #5537, #4539, #11414, #10256, #2064, #5611, #12571, #2143, #6625, #4459, #9092, #755, #3369, #4313, #6846, #976, #10410, #13741, #8080, #9017, #7853, #1985, #12805, #9250, #2210, #1057, #5763, #12069, #5122, #11784, #9837, #2293, #5050, #1415, #6121, #9917, #488, #5203, #14415, #14650, #3813, #2730, #9396, #336, #4050, #3522, #6283, #9765, #12960, #1570, #8517, #15288, #8230, #2813, #11713, #6359, #12233, #10834, #6997, #1132, #10999, #8756, #13251, #13327, #10555, #14495, #5835, #10919, #4681, #11071, #14122, #2367, #7435, #13408, #7065, #253, #3892, #4968, #9683, #7514, #2655, #8592, #7356, #1645, #1489, #6204, #12153, #414, #14569, #3969, #8675, #8903, #14878, #4197, #10289, #5351, #1800, #9990, #6511, #13633, #11226, #7664, #3108, #14802, #13709, #3034, #4126, #7888, #7819, #6736, #12533, #11451, #12461, #2885, #645, #1947, #12611, #14728, #7745, #9057, #1879, #10140, #11296, #11373, #12379, #6660, #10066, #798, #13486, #1715, #2026, #6586, #7586, #3175, #871, #5574, #8980, #4275, #12302, #15026, #5422, #5500 ),
 ( #10222, #717, #14955, #6429, #4349, #2955, #4416, #13778, #11149, #568, #5280, #8827, #13554, #10518, #1015, #5723, #9282, #11596, #9127, #15253, #3561, #10442, #8041, #2399, #12688, #2253, #1093, #15180, #3482, #4572, #2102, #11743, #10362, #11525, #7030, #14006, #3404, #941, #15102, #8113, #12841, #11675, #6809, #12767, #6958, #5644, #5798, #2176, #4496, #9204, #4644, #13934, #2332, #3332, #6880, #9353, #10585, #1163, #5866, #3, #14079, #13855, #8191, #12918, #4722, #9434, #14160, #8266, #10668, #12995, #7965, #11816, #7095, #1236, #3254, #5944, #84, #14306, #12133, #13148, #8497, #12046, #1395, #12212, #7493, #13231, #1627, #4945, #8337, #13386, #10898, #10813, #13306, #11975, #2557, #8652, #5105, #3872, #1317, #7335, #4867, #3707, #2708, #9579, #8415, #229, #6098, #10743, #6179, #6340, #9660, #7260, #9509, #1549, #2477, #14392, #3790, #314, #11894, #6262, #2791, #11054, #4796, #10979, #13062, #8573, #9820, #7411, #3948, #2633, #5028, #14233, #14552, #3635, #7173, #9747, #14475, #6022, #158, #1466, #396, #7725, #11206, #4180, #546, #14861, #4257, #13617, #4332, #4109, #6488, #9036, #12590, #8959, #10047, #3086, #9970, #7801, #471, #3018, #14709, #8810, #7868, #13760, #3156, #12362, #2007, #1780, #700, #7569, #12439, #6718, #1698, #13689, #1860, #11130, #12514, #628, #13467, #6411, #778, #9895, #5184, #10202, #13540, #14631, #4030, #1930, #8734, #5333, #11279, #2870, #6567, #12288, #8885, #5259, #2939, #7644, #14783, #5405, #11350, #10120, #6642, #5484, #14936, #4700, #11726, #3314, #13988, #10338, #5849, #13917, #15080, #9185, #8097, #9413, #6937, #3460, #6863, #12822, #2161, #8247, #8025, #4475, #7947, #12749, #11576, #993, #5625, #1073, #5704, #11655, #10423, #2082, #10568, #5781, #14138, #10502, #3538, #15159, #852 ),
 ( #2230, #12666, #4627, #6795, #4555, #9264, #12899, #9338, #8171, #2310, #3385, #15236, #14061, #12975, #7011, #1146, #11509, #15304, #2379, #11430, #5555, #10270, #15003, #4399, #9108, #925, #13831, #3234, #3853, #4922, #8550, #13126, #7077, #10722, #13209, #14456, #8318, #8393, #294, #2536, #10795, #1375, #7313, #11873, #3771, #1297, #2612, #11797, #4772, #13286, #14284, #1211, #2689, #7388, #12110, #8475, #9638, #5921, #10647, #14372, #12027, #1449, #7238, #209, #5998, #6154, #10875, #5009, #63, #3684, #11950, #9487, #14212, #9726, #3614, #13044, #6077, #2454, #7150, #136, #4848, #9559, #13028, #3599, #8300, #2206, #2434, #6913, #5830, #12726, #3436, #7128, #6841, #9387, #8147, #972, #4676, #11634, #3292, #11556, #5898, #15059, #9469, #43, #15138, #10320, #4453, #14117, #11849, #1052, #1127, #13894, #2288, #9167, #14039, #5606, #14195, #2137, #5679, #10551, #1196, #8004, #10406, #6993, #4533, #9244, #10620, #12800, #12877, #13970, #4753, #8076, #3365, #5759, #11709, #10481, #15284, #12956, #15216, #4607, #9317, #3518, #8226, #2363, #7060, #11779, #12007, #13186, #3831, #14270, #194, #8455, #3669, #13266, #4904, #9544, #1355, #2671, #2517, #9780, #7212, #9616, #14347, #2751, #14512, #8609, #7455, #6139, #5979, #7371, #8532, #2593, #10853, #6222, #12086, #2832, #5142, #118, #3988, #1510, #272, #10702, #1590, #4832, #10777, #13343, #3749, #4987, #10938, #7294, #8693, #13428, #9702, #7533, #1433, #8372, #9853, #355, #14435, #3912, #5068, #12172, #14586, #6300, #11017, #13101, #432, #6059, #1275, #11931, #1735, #6447, #7683, #4144, #2901, #13648, #13793, #12396, #10010, #1660, #8995, #9932, #14744, #6529, #3050, #4071, #13723, #10237, #3191, #12250, #3122, #5222, #734, #12550, #5438, #11391, #5298, #7761, #6373, #1893, #11164 ),
 ( #586, #8843, #8919, #5515, #12475, #4291, #1817, #6603, #2971, #9072, #13570, #11242, #8772, #661, #5366, #10083, #14817, #11312, #4214, #10158, #14893, #4364, #14970, #11086, #7836, #504, #1961, #6677, #13505, #813, #14667, #7603, #12317, #4665, #6981, #5745, #4520, #15273, #106, #9303, #11621, #3276, #10607, #11544, #1038, #8135, #9373, #5666, #31, #11839, #4819, #13881, #4742, #6828, #2352, #14183, #7050, #13018, #6900, #14105, #7989, #3505, #3353, #5968, #10467, #12944, #9457, #10391, #1263, #8064, #8213, #15201, #4594, #14026, #3423, #12713, #11765, #8289, #12864, #12788, #7116, #2125, #11697, #5818, #2276, #1185, #1116, #959, #5887, #15125, #9227, #3587, #10538, #2420, #13956, #2193, #10688, #6125, #12072, #7198, #8441, #1420, #11917, #6208, #13172, #2503, #9604, #10923, #10766, #2735, #181, #2581, #7282, #11004, #7441, #1573, #418, #14419, #14258, #340, #1496, #10839, #3817, #14498, #5055, #11074, #13414, #8358, #12237, #9768, #8521, #3657, #9841, #13086, #3734, #6286, #11995, #13254, #3897, #258, #1649, #6362, #2659, #491, #9686, #1343, #4971, #12157, #7360, #8596, #2817, #14572, #13330, #6046, #5128, #14333, #3974, #8679, #4893, #7518, #9532, #12384, #11153, #6591, #6741, #650, #2958, #9921, #1950, #2889, #7669, #14805, #11300, #12306, #6663, #3180, #11454, #5208, #11378, #13491, #8983, #5503, #13712, #4352, #13559, #721, #14653, #10146, #9996, #12615, #1805, #4278, #802, #1719, #7891, #14732, #5425, #6515, #11229, #5354, #10070, #4057, #14881, #14958, #4201, #4131, #13781, #8760, #13636, #12464, #8907, #3111, #3038, #7591, #7822, #6434, #573, #12538, #7748, #1882, #5284, #8831, #10225, #9060, #2029, #13859, #15308, #8251, #3257, #13047, #4705, #9132, #1149, #2458, #2106, #9562, #7015, #9417, #14141, #2540, #14287 ) ),
 .UNSPECIFIED., .T., .F., .T. ) 
 B_SPLINE_SURFACE_WITH_KNOTS ( ( 4, 3, 4 ),
 ( 3, 2, 2, 2, 2, 2, 2, 2, 2, 2, 2, 2, 2, 2, 2, 2, 2, 2, 2, 2, 2, 2, 2, 2, 2, 2, 2, 2, 2, 2, 2, 2, 2, 2, 2, 2, 2, 2, 2, 2, 2, 2, 2, 2, 2, 2, 2, 2, 2, 2, 2, 2, 2, 2, 2, 2, 2, 2, 2, 2, 2, 2, 2, 2, 2, 2, 2, 2, 2, 2, 2, 2, 2, 2, 2, 2, 2, 2, 2, 2, 2, 2, 2, 2, 2, 2, 2, 2, 2, 2, 2, 2, 2, 2, 2, 2, 2, 2, 2, 2, 2, 2, 2, 2, 2, 2, 2, 2, 2, 2, 2, 2, 2, 2, 2, 2, 2, 2, 2, 2, 3 ),
 ( 0.000000000000000000, 0.5000000000000000000, 1.000000000000000000 ),
 ( 0.000000000000000000, 0.008333333333333333218, 0.01666666666666666644, 0.02500000000000000139, 0.03333333333333333287, 0.04166666666666666435, 0.05000000000000000278, 0.05833333333333333426, 0.06666666666666666574, 0.07499999999999999722, 0.08333333333333332871, 0.09166666666666666019, 0.1000000000000000056, 0.1083333333333333370, 0.1166666666666666685, 0.1250000000000000000, 0.1333333333333333315, 0.1416666666666666630, 0.1499999999999999944, 0.1583333333333333259, 0.1666666666666666574, 0.1749999999999999889, 0.1833333333333333204, 0.1916666666666666519, 0.2000000000000000111, 0.2083333333333333426, 0.2166666666666666741, 0.2250000000000000056, 0.2333333333333333370, 0.2416666666666666685, 0.2500000000000000000, 0.2583333333333333037, 0.2666666666666666630, 0.2750000000000000222, 0.2833333333333333259, 0.2916666666666666852, 0.2999999999999999889, 0.3083333333333333481, 0.3166666666666666519, 0.3250000000000000111, 0.3333333333333333148, 0.3416666666666666741, 0.3499999999999999778, 0.3583333333333333370, 0.3666666666666666408, 0.3750000000000000000, 0.3833333333333333037, 0.3916666666666666630, 0.4000000000000000222, 0.4083333333333333259, 0.4166666666666666852, 0.4249999999999999889, 0.4333333333333333481, 0.4416666666666666519, 0.4500000000000000111, 0.4583333333333333148, 0.4666666666666666741, 0.4749999999999999778, 0.4833333333333333370, 0.4916666666666666408, 0.5000000000000000000, 0.5083333333333333037, 0.5166666666666666075, 0.5250000000000000222, 0.5333333333333333259, 0.5416666666666666297, 0.5500000000000000444, 0.5583333333333333481, 0.5666666666666666519, 0.5749999999999999556, 0.5833333333333333703, 0.5916666666666666741, 0.5999999999999999778, 0.6083333333333332815, 0.6166666666666666963, 0.6250000000000000000, 0.6333333333333333037, 0.6416666666666666075, 0.6500000000000000222, 0.6583333333333333259, 0.6666666666666666297, 0.6750000000000000444, 0.6833333333333333481, 0.6916666666666666519, 0.6999999999999999556, 0.7083333333333333703, 0.7166666666666666741, 0.7249999999999999778, 0.7333333333333332815, 0.7416666666666666963, 0.7500000000000000000, 0.7583333333333333037, 0.7666666666666666075, 0.7750000000000000222, 0.7833333333333333259, 0.7916666666666666297, 0.8000000000000000444, 0.8083333333333333481, 0.8166666666666666519, 0.8249999999999999556, 0.8333333333333333703, 0.8416666666666666741, 0.8499999999999999778, 0.8583333333333332815, 0.8666666666666666963, 0.8750000000000000000, 0.8833333333333333037, 0.8916666666666666075, 0.9000000000000000222, 0.9083333333333333259, 0.9166666666666666297, 0.9249999999999999334, 0.9333333333333333481, 0.9416666666666666519, 0.9499999999999999556, 0.9583333333333333703, 0.9666666666666666741, 0.9749999999999999778, 0.9833333333333332815, 0.9916666666666666963, 1.000000000000000000 ),
 .UNSPECIFIED. ) 
 GEOMETRIC_REPRESENTATION_ITEM ( )  RATIONAL_B_SPLINE_SURFACE ( (
 ( 1.000000000000000000, 0.9238795325112867385, 1.000000000000000000, 0.9238795325112867385, 1.000000000000000000, 0.9238795325112867385, 1.000000000000000000, 0.9238795325112867385, 1.000000000000000000, 0.9238795325112867385, 1.000000000000000000, 0.9238795325112867385, 1.000000000000000000, 0.9238795325112867385, 1.000000000000000000, 0.9238795325112867385, 1.000000000000000000, 0.9238795325112867385, 1.000000000000000000, 0.9238795325112867385, 1.000000000000000000, 0.9238795325112867385, 1.000000000000000000, 0.9238795325112867385, 1.000000000000000000, 0.9238795325112867385, 1.000000000000000000, 0.9238795325112867385, 1.000000000000000000, 0.9238795325112867385, 1.000000000000000000, 0.9238795325112867385, 1.000000000000000000, 0.9238795325112867385, 1.000000000000000000, 0.9238795325112867385, 1.000000000000000000, 0.9238795325112867385, 1.000000000000000000, 0.9238795325112867385, 1.000000000000000000, 0.9238795325112867385, 1.000000000000000000, 0.9238795325112867385, 1.000000000000000000, 0.9238795325112867385, 1.000000000000000000, 0.9238795325112867385, 1.000000000000000000, 0.9238795325112867385, 1.000000000000000000, 0.9238795325112867385, 1.000000000000000000, 0.9238795325112867385, 1.000000000000000000, 0.9238795325112867385, 1.000000000000000000, 0.9238795325112867385, 1.000000000000000000, 0.9238795325112867385, 1.000000000000000000, 0.9238795325112867385, 1.000000000000000000, 0.9238795325112867385, 1.000000000000000000, 0.9238795325112867385, 1.000000000000000000, 0.9238795325112867385, 1.000000000000000000, 0.9238795325112867385, 1.000000000000000000, 0.9238795325112867385, 1.000000000000000000, 0.9238795325112867385, 1.000000000000000000, 0.9238795325112867385, 1.000000000000000000, 0.9238795325112867385, 1.000000000000000000, 0.9238795325112867385, 1.000000000000000000, 0.9238795325112867385, 1.000000000000000000, 0.9238795325112867385, 1.000000000000000000, 0.9238795325112867385, 1.000000000000000000, 0.9238795325112867385, 1.000000000000000000, 0.9238795325112867385, 1.000000000000000000, 0.9238795325112867385, 1.000000000000000000, 0.9238795325112867385, 1.000000000000000000, 0.9238795325112867385, 1.000000000000000000, 0.9238795325112867385, 1.000000000000000000, 0.9238795325112867385, 1.000000000000000000, 0.9238795325112867385, 1.000000000000000000, 0.9238795325112867385, 1.000000000000000000, 0.9238795325112867385, 1.000000000000000000, 0.9238795325112867385, 1.000000000000000000, 0.9238795325112867385, 1.000000000000000000, 0.9238795325112867385, 1.000000000000000000, 0.9238795325112867385, 1.000000000000000000, 0.9238795325112867385, 1.000000000000000000, 0.9238795325112867385, 1.000000000000000000, 0.9238795325112867385, 1.000000000000000000, 0.9238795325112867385, 1.000000000000000000, 0.9238795325112867385, 1.000000000000000000, 0.9238795325112867385, 1.000000000000000000, 0.9238795325112867385, 1.000000000000000000, 0.9238795325112867385, 1.000000000000000000, 0.9238795325112867385, 1.000000000000000000, 0.9238795325112867385, 1.000000000000000000, 0.9238795325112867385, 1.000000000000000000, 0.9238795325112867385, 1.000000000000000000, 0.9238795325112867385, 1.000000000000000000, 0.9238795325112867385, 1.000000000000000000, 0.9238795325112867385, 1.000000000000000000, 0.9238795325112867385, 1.000000000000000000, 0.9238795325112867385, 1.000000000000000000, 0.9238795325112867385, 1.000000000000000000, 0.9238795325112867385, 1.000000000000000000, 0.9238795325112867385, 1.000000000000000000, 0.9238795325112867385, 1.000000000000000000, 0.9238795325112867385, 1.000000000000000000, 0.9238795325112867385, 1.000000000000000000, 0.9238795325112867385, 1.000000000000000000, 0.9238795325112867385, 1.000000000000000000, 0.9238795325112867385, 1.000000000000000000, 0.9238795325112867385, 1.000000000000000000, 0.9238795325112867385, 1.000000000000000000, 0.9238795325112867385, 1.000000000000000000, 0.9238795325112867385, 1.000000000000000000, 0.9238795325112867385, 1.000000000000000000, 0.9238795325112867385, 1.000000000000000000, 0.9238795325112867385, 1.000000000000000000, 0.9238795325112867385, 1.000000000000000000, 0.9238795325112867385, 1.000000000000000000, 0.9238795325112867385, 1.000000000000000000, 0.9238795325112867385, 1.000000000000000000, 0.9238795325112867385, 1.000000000000000000, 0.9238795325112867385, 1.000000000000000000, 0.9238795325112867385, 1.000000000000000000, 0.9238795325112867385, 1.000000000000000000, 0.9238795325112867385, 1.000000000000000000, 0.9238795325112867385, 1.000000000000000000, 0.9238795325112867385, 1.000000000000000000, 0.9238795325112867385, 1.000000000000000000, 0.9238795325112867385, 1.000000000000000000, 0.9238795325112867385, 1.000000000000000000, 0.9238795325112867385, 1.000000000000000000, 0.9238795325112867385, 1.000000000000000000, 0.9238795325112867385, 1.000000000000000000, 0.9238795325112867385, 1.000000000000000000, 0.9238795325112867385, 1.000000000000000000, 0.9238795325112867385, 1.000000000000000000, 0.9238795325112867385, 1.000000000000000000, 0.9238795325112867385, 1.000000000000000000, 0.9238795325112867385, 1.000000000000000000, 0.9238795325112867385, 1.000000000000000000, 0.9238795325112867385, 1.000000000000000000, 0.9238795325112867385, 1.000000000000000000, 0.9238795325112867385, 1.000000000000000000, 0.9238795325112867385, 1.000000000000000000, 0.9238795325112867385, 1.000000000000000000, 0.9238795325112867385, 1.000000000000000000),
 ( 0.3333333333333333703, 0.3079598441704289313, 0.3333333333333333703, 0.3079598441704289313, 0.3333333333333333703, 0.3079598441704289313, 0.3333333333333333703, 0.3079598441704289313, 0.3333333333333333703, 0.3079598441704289313, 0.3333333333333333703, 0.3079598441704289313, 0.3333333333333333703, 0.3079598441704289313, 0.3333333333333333703, 0.3079598441704289313, 0.3333333333333333703, 0.3079598441704289313, 0.3333333333333333703, 0.3079598441704289313, 0.3333333333333333703, 0.3079598441704289313, 0.3333333333333333703, 0.3079598441704289313, 0.3333333333333333703, 0.3079598441704289313, 0.3333333333333333703, 0.3079598441704289313, 0.3333333333333333703, 0.3079598441704289313, 0.3333333333333333703, 0.3079598441704289313, 0.3333333333333333703, 0.3079598441704289313, 0.3333333333333333703, 0.3079598441704289313, 0.3333333333333333703, 0.3079598441704289313, 0.3333333333333333703, 0.3079598441704289313, 0.3333333333333333703, 0.3079598441704289313, 0.3333333333333333703, 0.3079598441704289313, 0.3333333333333333703, 0.3079598441704289313, 0.3333333333333333703, 0.3079598441704289313, 0.3333333333333333703, 0.3079598441704289313, 0.3333333333333333703, 0.3079598441704289313, 0.3333333333333333703, 0.3079598441704289313, 0.3333333333333333703, 0.3079598441704289313, 0.3333333333333333703, 0.3079598441704289313, 0.3333333333333333703, 0.3079598441704289313, 0.3333333333333333703, 0.3079598441704289313, 0.3333333333333333703, 0.3079598441704289313, 0.3333333333333333703, 0.3079598441704289313, 0.3333333333333333703, 0.3079598441704289313, 0.3333333333333333703, 0.3079598441704289313, 0.3333333333333333703, 0.3079598441704289313, 0.3333333333333333703, 0.3079598441704289313, 0.3333333333333333703, 0.3079598441704289313, 0.3333333333333333703, 0.3079598441704289313, 0.3333333333333333703, 0.3079598441704289313, 0.3333333333333333703, 0.3079598441704289313, 0.3333333333333333703, 0.3079598441704289313, 0.3333333333333333703, 0.3079598441704289313, 0.3333333333333333703, 0.3079598441704289313, 0.3333333333333333703, 0.3079598441704289313, 0.3333333333333333703, 0.3079598441704289313, 0.3333333333333333703, 0.3079598441704289313, 0.3333333333333333703, 0.3079598441704289313, 0.3333333333333333703, 0.3079598441704289313, 0.3333333333333333703, 0.3079598441704289313, 0.3333333333333333703, 0.3079598441704289313, 0.3333333333333333703, 0.3079598441704289313, 0.3333333333333333703, 0.3079598441704289313, 0.3333333333333333703, 0.3079598441704289313, 0.3333333333333333703, 0.3079598441704289313, 0.3333333333333333703, 0.3079598441704289313, 0.3333333333333333703, 0.3079598441704289313, 0.3333333333333333703, 0.3079598441704289313, 0.3333333333333333703, 0.3079598441704289313, 0.3333333333333333703, 0.3079598441704289313, 0.3333333333333333703, 0.3079598441704289313, 0.3333333333333333703, 0.3079598441704289313, 0.3333333333333333703, 0.3079598441704289313, 0.3333333333333333703, 0.3079598441704289313, 0.3333333333333333703, 0.3079598441704289313, 0.3333333333333333703, 0.3079598441704289313, 0.3333333333333333703, 0.3079598441704289313, 0.3333333333333333703, 0.3079598441704289313, 0.3333333333333333703, 0.3079598441704289313, 0.3333333333333333703, 0.3079598441704289313, 0.3333333333333333703, 0.3079598441704289313, 0.3333333333333333703, 0.3079598441704289313, 0.3333333333333333703, 0.3079598441704289313, 0.3333333333333333703, 0.3079598441704289313, 0.3333333333333333703, 0.3079598441704289313, 0.3333333333333333703, 0.3079598441704289313, 0.3333333333333333703, 0.3079598441704289313, 0.3333333333333333703, 0.3079598441704289313, 0.3333333333333333703, 0.3079598441704289313, 0.3333333333333333703, 0.3079598441704289313, 0.3333333333333333703, 0.3079598441704289313, 0.3333333333333333703, 0.3079598441704289313, 0.3333333333333333703, 0.3079598441704289313, 0.3333333333333333703, 0.3079598441704289313, 0.3333333333333333703, 0.3079598441704289313, 0.3333333333333333703, 0.3079598441704289313, 0.3333333333333333703, 0.3079598441704289313, 0.3333333333333333703, 0.3079598441704289313, 0.3333333333333333703, 0.3079598441704289313, 0.3333333333333333703, 0.3079598441704289313, 0.3333333333333333703, 0.3079598441704289313, 0.3333333333333333703, 0.3079598441704289313, 0.3333333333333333703, 0.3079598441704289313, 0.3333333333333333703, 0.3079598441704289313, 0.3333333333333333703, 0.3079598441704289313, 0.3333333333333333703, 0.3079598441704289313, 0.3333333333333333703, 0.3079598441704289313, 0.3333333333333333703, 0.3079598441704289313, 0.3333333333333333703, 0.3079598441704289313, 0.3333333333333333703, 0.3079598441704289313, 0.3333333333333333703, 0.3079598441704289313, 0.3333333333333333703, 0.3079598441704289313, 0.3333333333333333703, 0.3079598441704289313, 0.3333333333333333703, 0.3079598441704289313, 0.3333333333333333703, 0.3079598441704289313, 0.3333333333333333703, 0.3079598441704289313, 0.3333333333333333703, 0.3079598441704289313, 0.3333333333333333703, 0.3079598441704289313, 0.3333333333333333703, 0.3079598441704289313, 0.3333333333333333703, 0.3079598441704289313, 0.3333333333333333703, 0.3079598441704289313, 0.3333333333333333703, 0.3079598441704289313, 0.3333333333333333703, 0.3079598441704289313, 0.3333333333333333703, 0.3079598441704289313, 0.3333333333333333703, 0.3079598441704289313, 0.3333333333333333703, 0.3079598441704289313, 0.3333333333333333703, 0.3079598441704289313, 0.3333333333333333703, 0.3079598441704289313, 0.3333333333333333703, 0.3079598441704289313, 0.3333333333333333703, 0.3079598441704289313, 0.3333333333333333703),
 ( 0.3333333333333333703, 0.3079598441704289313, 0.3333333333333333703, 0.3079598441704289313, 0.3333333333333333703, 0.3079598441704289313, 0.3333333333333333703, 0.3079598441704289313, 0.3333333333333333703, 0.3079598441704289313, 0.3333333333333333703, 0.3079598441704289313, 0.3333333333333333703, 0.3079598441704289313, 0.3333333333333333703, 0.3079598441704289313, 0.3333333333333333703, 0.3079598441704289313, 0.3333333333333333703, 0.3079598441704289313, 0.3333333333333333703, 0.3079598441704289313, 0.3333333333333333703, 0.3079598441704289313, 0.3333333333333333703, 0.3079598441704289313, 0.3333333333333333703, 0.3079598441704289313, 0.3333333333333333703, 0.3079598441704289313, 0.3333333333333333703, 0.3079598441704289313, 0.3333333333333333703, 0.3079598441704289313, 0.3333333333333333703, 0.3079598441704289313, 0.3333333333333333703, 0.3079598441704289313, 0.3333333333333333703, 0.3079598441704289313, 0.3333333333333333703, 0.3079598441704289313, 0.3333333333333333703, 0.3079598441704289313, 0.3333333333333333703, 0.3079598441704289313, 0.3333333333333333703, 0.3079598441704289313, 0.3333333333333333703, 0.3079598441704289313, 0.3333333333333333703, 0.3079598441704289313, 0.3333333333333333703, 0.3079598441704289313, 0.3333333333333333703, 0.3079598441704289313, 0.3333333333333333703, 0.3079598441704289313, 0.3333333333333333703, 0.3079598441704289313, 0.3333333333333333703, 0.3079598441704289313, 0.3333333333333333703, 0.3079598441704289313, 0.3333333333333333703, 0.3079598441704289313, 0.3333333333333333703, 0.3079598441704289313, 0.3333333333333333703, 0.3079598441704289313, 0.3333333333333333703, 0.3079598441704289313, 0.3333333333333333703, 0.3079598441704289313, 0.3333333333333333703, 0.3079598441704289313, 0.3333333333333333703, 0.3079598441704289313, 0.3333333333333333703, 0.3079598441704289313, 0.3333333333333333703, 0.3079598441704289313, 0.3333333333333333703, 0.3079598441704289313, 0.3333333333333333703, 0.3079598441704289313, 0.3333333333333333703, 0.3079598441704289313, 0.3333333333333333703, 0.3079598441704289313, 0.3333333333333333703, 0.3079598441704289313, 0.3333333333333333703, 0.3079598441704289313, 0.3333333333333333703, 0.3079598441704289313, 0.3333333333333333703, 0.3079598441704289313, 0.3333333333333333703, 0.3079598441704289313, 0.3333333333333333703, 0.3079598441704289313, 0.3333333333333333703, 0.3079598441704289313, 0.3333333333333333703, 0.3079598441704289313, 0.3333333333333333703, 0.3079598441704289313, 0.3333333333333333703, 0.3079598441704289313, 0.3333333333333333703, 0.3079598441704289313, 0.3333333333333333703, 0.3079598441704289313, 0.3333333333333333703, 0.3079598441704289313, 0.3333333333333333703, 0.3079598441704289313, 0.3333333333333333703, 0.3079598441704289313, 0.3333333333333333703, 0.3079598441704289313, 0.3333333333333333703, 0.3079598441704289313, 0.3333333333333333703, 0.3079598441704289313, 0.3333333333333333703, 0.3079598441704289313, 0.3333333333333333703, 0.3079598441704289313, 0.3333333333333333703, 0.3079598441704289313, 0.3333333333333333703, 0.3079598441704289313, 0.3333333333333333703, 0.3079598441704289313, 0.3333333333333333703, 0.3079598441704289313, 0.3333333333333333703, 0.3079598441704289313, 0.3333333333333333703, 0.3079598441704289313, 0.3333333333333333703, 0.3079598441704289313, 0.3333333333333333703, 0.3079598441704289313, 0.3333333333333333703, 0.3079598441704289313, 0.3333333333333333703, 0.3079598441704289313, 0.3333333333333333703, 0.3079598441704289313, 0.3333333333333333703, 0.3079598441704289313, 0.3333333333333333703, 0.3079598441704289313, 0.3333333333333333703, 0.3079598441704289313, 0.3333333333333333703, 0.3079598441704289313, 0.3333333333333333703, 0.3079598441704289313, 0.3333333333333333703, 0.3079598441704289313, 0.3333333333333333703, 0.3079598441704289313, 0.3333333333333333703, 0.3079598441704289313, 0.3333333333333333703, 0.3079598441704289313, 0.3333333333333333703, 0.3079598441704289313, 0.3333333333333333703, 0.3079598441704289313, 0.3333333333333333703, 0.3079598441704289313, 0.3333333333333333703, 0.3079598441704289313, 0.3333333333333333703, 0.3079598441704289313, 0.3333333333333333703, 0.3079598441704289313, 0.3333333333333333703, 0.3079598441704289313, 0.3333333333333333703, 0.3079598441704289313, 0.3333333333333333703, 0.3079598441704289313, 0.3333333333333333703, 0.3079598441704289313, 0.3333333333333333703, 0.3079598441704289313, 0.3333333333333333703, 0.3079598441704289313, 0.3333333333333333703, 0.3079598441704289313, 0.3333333333333333703, 0.3079598441704289313, 0.3333333333333333703, 0.3079598441704289313, 0.3333333333333333703, 0.3079598441704289313, 0.3333333333333333703, 0.3079598441704289313, 0.3333333333333333703, 0.3079598441704289313, 0.3333333333333333703, 0.3079598441704289313, 0.3333333333333333703, 0.3079598441704289313, 0.3333333333333333703, 0.3079598441704289313, 0.3333333333333333703, 0.3079598441704289313, 0.3333333333333333703, 0.3079598441704289313, 0.3333333333333333703, 0.3079598441704289313, 0.3333333333333333703, 0.3079598441704289313, 0.3333333333333333703, 0.3079598441704289313, 0.3333333333333333703, 0.3079598441704289313, 0.3333333333333333703, 0.3079598441704289313, 0.3333333333333333703, 0.3079598441704289313, 0.3333333333333333703, 0.3079598441704289313, 0.3333333333333333703, 0.3079598441704289313, 0.3333333333333333703, 0.3079598441704289313, 0.3333333333333333703, 0.3079598441704289313, 0.3333333333333333703, 0.3079598441704289313, 0.3333333333333333703, 0.3079598441704289313, 0.3333333333333333703),
 ( 1.000000000000000000, 0.9238795325112867385, 1.000000000000000000, 0.9238795325112867385, 1.000000000000000000, 0.9238795325112867385, 1.000000000000000000, 0.9238795325112867385, 1.000000000000000000, 0.9238795325112867385, 1.000000000000000000, 0.9238795325112867385, 1.000000000000000000, 0.9238795325112867385, 1.000000000000000000, 0.9238795325112867385, 1.000000000000000000, 0.9238795325112867385, 1.000000000000000000, 0.9238795325112867385, 1.000000000000000000, 0.9238795325112867385, 1.000000000000000000, 0.9238795325112867385, 1.000000000000000000, 0.9238795325112867385, 1.000000000000000000, 0.9238795325112867385, 1.000000000000000000, 0.9238795325112867385, 1.000000000000000000, 0.9238795325112867385, 1.000000000000000000, 0.9238795325112867385, 1.000000000000000000, 0.9238795325112867385, 1.000000000000000000, 0.9238795325112867385, 1.000000000000000000, 0.9238795325112867385, 1.000000000000000000, 0.9238795325112867385, 1.000000000000000000, 0.9238795325112867385, 1.000000000000000000, 0.9238795325112867385, 1.000000000000000000, 0.9238795325112867385, 1.000000000000000000, 0.9238795325112867385, 1.000000000000000000, 0.9238795325112867385, 1.000000000000000000, 0.9238795325112867385, 1.000000000000000000, 0.9238795325112867385, 1.000000000000000000, 0.9238795325112867385, 1.000000000000000000, 0.9238795325112867385, 1.000000000000000000, 0.9238795325112867385, 1.000000000000000000, 0.9238795325112867385, 1.000000000000000000, 0.9238795325112867385, 1.000000000000000000, 0.9238795325112867385, 1.000000000000000000, 0.9238795325112867385, 1.000000000000000000, 0.9238795325112867385, 1.000000000000000000, 0.9238795325112867385, 1.000000000000000000, 0.9238795325112867385, 1.000000000000000000, 0.9238795325112867385, 1.000000000000000000, 0.9238795325112867385, 1.000000000000000000, 0.9238795325112867385, 1.000000000000000000, 0.9238795325112867385, 1.000000000000000000, 0.9238795325112867385, 1.000000000000000000, 0.9238795325112867385, 1.000000000000000000, 0.9238795325112867385, 1.000000000000000000, 0.9238795325112867385, 1.000000000000000000, 0.9238795325112867385, 1.000000000000000000, 0.9238795325112867385, 1.000000000000000000, 0.9238795325112867385, 1.000000000000000000, 0.9238795325112867385, 1.000000000000000000, 0.9238795325112867385, 1.000000000000000000, 0.9238795325112867385, 1.000000000000000000, 0.9238795325112867385, 1.000000000000000000, 0.9238795325112867385, 1.000000000000000000, 0.9238795325112867385, 1.000000000000000000, 0.9238795325112867385, 1.000000000000000000, 0.9238795325112867385, 1.000000000000000000, 0.9238795325112867385, 1.000000000000000000, 0.9238795325112867385, 1.000000000000000000, 0.9238795325112867385, 1.000000000000000000, 0.9238795325112867385, 1.000000000000000000, 0.9238795325112867385, 1.000000000000000000, 0.9238795325112867385, 1.000000000000000000, 0.9238795325112867385, 1.000000000000000000, 0.9238795325112867385, 1.000000000000000000, 0.9238795325112867385, 1.000000000000000000, 0.9238795325112867385, 1.000000000000000000, 0.9238795325112867385, 1.000000000000000000, 0.9238795325112867385, 1.000000000000000000, 0.9238795325112867385, 1.000000000000000000, 0.9238795325112867385, 1.000000000000000000, 0.9238795325112867385, 1.000000000000000000, 0.9238795325112867385, 1.000000000000000000, 0.9238795325112867385, 1.000000000000000000, 0.9238795325112867385, 1.000000000000000000, 0.9238795325112867385, 1.000000000000000000, 0.9238795325112867385, 1.000000000000000000, 0.9238795325112867385, 1.000000000000000000, 0.9238795325112867385, 1.000000000000000000, 0.9238795325112867385, 1.000000000000000000, 0.9238795325112867385, 1.000000000000000000, 0.9238795325112867385, 1.000000000000000000, 0.9238795325112867385, 1.000000000000000000, 0.9238795325112867385, 1.000000000000000000, 0.9238795325112867385, 1.000000000000000000, 0.9238795325112867385, 1.000000000000000000, 0.9238795325112867385, 1.000000000000000000, 0.9238795325112867385, 1.000000000000000000, 0.9238795325112867385, 1.000000000000000000, 0.9238795325112867385, 1.000000000000000000, 0.9238795325112867385, 1.000000000000000000, 0.9238795325112867385, 1.000000000000000000, 0.9238795325112867385, 1.000000000000000000, 0.9238795325112867385, 1.000000000000000000, 0.9238795325112867385, 1.000000000000000000, 0.9238795325112867385, 1.000000000000000000, 0.9238795325112867385, 1.000000000000000000, 0.9238795325112867385, 1.000000000000000000, 0.9238795325112867385, 1.000000000000000000, 0.9238795325112867385, 1.000000000000000000, 0.9238795325112867385, 1.000000000000000000, 0.9238795325112867385, 1.000000000000000000, 0.9238795325112867385, 1.000000000000000000, 0.9238795325112867385, 1.000000000000000000, 0.9238795325112867385, 1.000000000000000000, 0.9238795325112867385, 1.000000000000000000, 0.9238795325112867385, 1.000000000000000000, 0.9238795325112867385, 1.000000000000000000, 0.9238795325112867385, 1.000000000000000000, 0.9238795325112867385, 1.000000000000000000, 0.9238795325112867385, 1.000000000000000000, 0.9238795325112867385, 1.000000000000000000, 0.9238795325112867385, 1.000000000000000000, 0.9238795325112867385, 1.000000000000000000, 0.9238795325112867385, 1.000000000000000000, 0.9238795325112867385, 1.000000000000000000, 0.9238795325112867385, 1.000000000000000000, 0.9238795325112867385, 1.000000000000000000, 0.9238795325112867385, 1.000000000000000000, 0.9238795325112867385, 1.000000000000000000),
 ( 0.3333333333333333703, 0.3079598441704289313, 0.3333333333333333703, 0.3079598441704289313, 0.3333333333333333703, 0.3079598441704289313, 0.3333333333333333703, 0.3079598441704289313, 0.3333333333333333703, 0.3079598441704289313, 0.3333333333333333703, 0.3079598441704289313, 0.3333333333333333703, 0.3079598441704289313, 0.3333333333333333703, 0.3079598441704289313, 0.3333333333333333703, 0.3079598441704289313, 0.3333333333333333703, 0.3079598441704289313, 0.3333333333333333703, 0.3079598441704289313, 0.3333333333333333703, 0.3079598441704289313, 0.3333333333333333703, 0.3079598441704289313, 0.3333333333333333703, 0.3079598441704289313, 0.3333333333333333703, 0.3079598441704289313, 0.3333333333333333703, 0.3079598441704289313, 0.3333333333333333703, 0.3079598441704289313, 0.3333333333333333703, 0.3079598441704289313, 0.3333333333333333703, 0.3079598441704289313, 0.3333333333333333703, 0.3079598441704289313, 0.3333333333333333703, 0.3079598441704289313, 0.3333333333333333703, 0.3079598441704289313, 0.3333333333333333703, 0.3079598441704289313, 0.3333333333333333703, 0.3079598441704289313, 0.3333333333333333703, 0.3079598441704289313, 0.3333333333333333703, 0.3079598441704289313, 0.3333333333333333703, 0.3079598441704289313, 0.3333333333333333703, 0.3079598441704289313, 0.3333333333333333703, 0.3079598441704289313, 0.3333333333333333703, 0.3079598441704289313, 0.3333333333333333703, 0.3079598441704289313, 0.3333333333333333703, 0.3079598441704289313, 0.3333333333333333703, 0.3079598441704289313, 0.3333333333333333703, 0.3079598441704289313, 0.3333333333333333703, 0.3079598441704289313, 0.3333333333333333703, 0.3079598441704289313, 0.3333333333333333703, 0.3079598441704289313, 0.3333333333333333703, 0.3079598441704289313, 0.3333333333333333703, 0.3079598441704289313, 0.3333333333333333703, 0.3079598441704289313, 0.3333333333333333703, 0.3079598441704289313, 0.3333333333333333703, 0.3079598441704289313, 0.3333333333333333703, 0.3079598441704289313, 0.3333333333333333703, 0.3079598441704289313, 0.3333333333333333703, 0.3079598441704289313, 0.3333333333333333703, 0.3079598441704289313, 0.3333333333333333703, 0.3079598441704289313, 0.3333333333333333703, 0.3079598441704289313, 0.3333333333333333703, 0.3079598441704289313, 0.3333333333333333703, 0.3079598441704289313, 0.3333333333333333703, 0.3079598441704289313, 0.3333333333333333703, 0.3079598441704289313, 0.3333333333333333703, 0.3079598441704289313, 0.3333333333333333703, 0.3079598441704289313, 0.3333333333333333703, 0.3079598441704289313, 0.3333333333333333703, 0.3079598441704289313, 0.3333333333333333703, 0.3079598441704289313, 0.3333333333333333703, 0.3079598441704289313, 0.3333333333333333703, 0.3079598441704289313, 0.3333333333333333703, 0.3079598441704289313, 0.3333333333333333703, 0.3079598441704289313, 0.3333333333333333703, 0.3079598441704289313, 0.3333333333333333703, 0.3079598441704289313, 0.3333333333333333703, 0.3079598441704289313, 0.3333333333333333703, 0.3079598441704289313, 0.3333333333333333703, 0.3079598441704289313, 0.3333333333333333703, 0.3079598441704289313, 0.3333333333333333703, 0.3079598441704289313, 0.3333333333333333703, 0.3079598441704289313, 0.3333333333333333703, 0.3079598441704289313, 0.3333333333333333703, 0.3079598441704289313, 0.3333333333333333703, 0.3079598441704289313, 0.3333333333333333703, 0.3079598441704289313, 0.3333333333333333703, 0.3079598441704289313, 0.3333333333333333703, 0.3079598441704289313, 0.3333333333333333703, 0.3079598441704289313, 0.3333333333333333703, 0.3079598441704289313, 0.3333333333333333703, 0.3079598441704289313, 0.3333333333333333703, 0.3079598441704289313, 0.3333333333333333703, 0.3079598441704289313, 0.3333333333333333703, 0.3079598441704289313, 0.3333333333333333703, 0.3079598441704289313, 0.3333333333333333703, 0.3079598441704289313, 0.3333333333333333703, 0.3079598441704289313, 0.3333333333333333703, 0.3079598441704289313, 0.3333333333333333703, 0.3079598441704289313, 0.3333333333333333703, 0.3079598441704289313, 0.3333333333333333703, 0.3079598441704289313, 0.3333333333333333703, 0.3079598441704289313, 0.3333333333333333703, 0.3079598441704289313, 0.3333333333333333703, 0.3079598441704289313, 0.3333333333333333703, 0.3079598441704289313, 0.3333333333333333703, 0.3079598441704289313, 0.3333333333333333703, 0.3079598441704289313, 0.3333333333333333703, 0.3079598441704289313, 0.3333333333333333703, 0.3079598441704289313, 0.3333333333333333703, 0.3079598441704289313, 0.3333333333333333703, 0.3079598441704289313, 0.3333333333333333703, 0.3079598441704289313, 0.3333333333333333703, 0.3079598441704289313, 0.3333333333333333703, 0.3079598441704289313, 0.3333333333333333703, 0.3079598441704289313, 0.3333333333333333703, 0.3079598441704289313, 0.3333333333333333703, 0.3079598441704289313, 0.3333333333333333703, 0.3079598441704289313, 0.3333333333333333703, 0.3079598441704289313, 0.3333333333333333703, 0.3079598441704289313, 0.3333333333333333703, 0.3079598441704289313, 0.3333333333333333703, 0.3079598441704289313, 0.3333333333333333703, 0.3079598441704289313, 0.3333333333333333703, 0.3079598441704289313, 0.3333333333333333703, 0.3079598441704289313, 0.3333333333333333703, 0.3079598441704289313, 0.3333333333333333703, 0.3079598441704289313, 0.3333333333333333703, 0.3079598441704289313, 0.3333333333333333703, 0.3079598441704289313, 0.3333333333333333703, 0.3079598441704289313, 0.3333333333333333703, 0.3079598441704289313, 0.3333333333333333703, 0.3079598441704289313, 0.3333333333333333703, 0.3079598441704289313, 0.3333333333333333703),
 ( 0.3333333333333333703, 0.3079598441704289313, 0.3333333333333333703, 0.3079598441704289313, 0.3333333333333333703, 0.3079598441704289313, 0.3333333333333333703, 0.3079598441704289313, 0.3333333333333333703, 0.3079598441704289313, 0.3333333333333333703, 0.3079598441704289313, 0.3333333333333333703, 0.3079598441704289313, 0.3333333333333333703, 0.3079598441704289313, 0.3333333333333333703, 0.3079598441704289313, 0.3333333333333333703, 0.3079598441704289313, 0.3333333333333333703, 0.3079598441704289313, 0.3333333333333333703, 0.3079598441704289313, 0.3333333333333333703, 0.3079598441704289313, 0.3333333333333333703, 0.3079598441704289313, 0.3333333333333333703, 0.3079598441704289313, 0.3333333333333333703, 0.3079598441704289313, 0.3333333333333333703, 0.3079598441704289313, 0.3333333333333333703, 0.3079598441704289313, 0.3333333333333333703, 0.3079598441704289313, 0.3333333333333333703, 0.3079598441704289313, 0.3333333333333333703, 0.3079598441704289313, 0.3333333333333333703, 0.3079598441704289313, 0.3333333333333333703, 0.3079598441704289313, 0.3333333333333333703, 0.3079598441704289313, 0.3333333333333333703, 0.3079598441704289313, 0.3333333333333333703, 0.3079598441704289313, 0.3333333333333333703, 0.3079598441704289313, 0.3333333333333333703, 0.3079598441704289313, 0.3333333333333333703, 0.3079598441704289313, 0.3333333333333333703, 0.3079598441704289313, 0.3333333333333333703, 0.3079598441704289313, 0.3333333333333333703, 0.3079598441704289313, 0.3333333333333333703, 0.3079598441704289313, 0.3333333333333333703, 0.3079598441704289313, 0.3333333333333333703, 0.3079598441704289313, 0.3333333333333333703, 0.3079598441704289313, 0.3333333333333333703, 0.3079598441704289313, 0.3333333333333333703, 0.3079598441704289313, 0.3333333333333333703, 0.3079598441704289313, 0.3333333333333333703, 0.3079598441704289313, 0.3333333333333333703, 0.3079598441704289313, 0.3333333333333333703, 0.3079598441704289313, 0.3333333333333333703, 0.3079598441704289313, 0.3333333333333333703, 0.3079598441704289313, 0.3333333333333333703, 0.3079598441704289313, 0.3333333333333333703, 0.3079598441704289313, 0.3333333333333333703, 0.3079598441704289313, 0.3333333333333333703, 0.3079598441704289313, 0.3333333333333333703, 0.3079598441704289313, 0.3333333333333333703, 0.3079598441704289313, 0.3333333333333333703, 0.3079598441704289313, 0.3333333333333333703, 0.3079598441704289313, 0.3333333333333333703, 0.3079598441704289313, 0.3333333333333333703, 0.3079598441704289313, 0.3333333333333333703, 0.3079598441704289313, 0.3333333333333333703, 0.3079598441704289313, 0.3333333333333333703, 0.3079598441704289313, 0.3333333333333333703, 0.3079598441704289313, 0.3333333333333333703, 0.3079598441704289313, 0.3333333333333333703, 0.3079598441704289313, 0.3333333333333333703, 0.3079598441704289313, 0.3333333333333333703, 0.3079598441704289313, 0.3333333333333333703, 0.3079598441704289313, 0.3333333333333333703, 0.3079598441704289313, 0.3333333333333333703, 0.3079598441704289313, 0.3333333333333333703, 0.3079598441704289313, 0.3333333333333333703, 0.3079598441704289313, 0.3333333333333333703, 0.3079598441704289313, 0.3333333333333333703, 0.3079598441704289313, 0.3333333333333333703, 0.3079598441704289313, 0.3333333333333333703, 0.3079598441704289313, 0.3333333333333333703, 0.3079598441704289313, 0.3333333333333333703, 0.3079598441704289313, 0.3333333333333333703, 0.3079598441704289313, 0.3333333333333333703, 0.3079598441704289313, 0.3333333333333333703, 0.3079598441704289313, 0.3333333333333333703, 0.3079598441704289313, 0.3333333333333333703, 0.3079598441704289313, 0.3333333333333333703, 0.3079598441704289313, 0.3333333333333333703, 0.3079598441704289313, 0.3333333333333333703, 0.3079598441704289313, 0.3333333333333333703, 0.3079598441704289313, 0.3333333333333333703, 0.3079598441704289313, 0.3333333333333333703, 0.3079598441704289313, 0.3333333333333333703, 0.3079598441704289313, 0.3333333333333333703, 0.3079598441704289313, 0.3333333333333333703, 0.3079598441704289313, 0.3333333333333333703, 0.3079598441704289313, 0.3333333333333333703, 0.3079598441704289313, 0.3333333333333333703, 0.3079598441704289313, 0.3333333333333333703, 0.3079598441704289313, 0.3333333333333333703, 0.3079598441704289313, 0.3333333333333333703, 0.3079598441704289313, 0.3333333333333333703, 0.3079598441704289313, 0.3333333333333333703, 0.3079598441704289313, 0.3333333333333333703, 0.3079598441704289313, 0.3333333333333333703, 0.3079598441704289313, 0.3333333333333333703, 0.3079598441704289313, 0.3333333333333333703, 0.3079598441704289313, 0.3333333333333333703, 0.3079598441704289313, 0.3333333333333333703, 0.3079598441704289313, 0.3333333333333333703, 0.3079598441704289313, 0.3333333333333333703, 0.3079598441704289313, 0.3333333333333333703, 0.3079598441704289313, 0.3333333333333333703, 0.3079598441704289313, 0.3333333333333333703, 0.3079598441704289313, 0.3333333333333333703, 0.3079598441704289313, 0.3333333333333333703, 0.3079598441704289313, 0.3333333333333333703, 0.3079598441704289313, 0.3333333333333333703, 0.3079598441704289313, 0.3333333333333333703, 0.3079598441704289313, 0.3333333333333333703, 0.3079598441704289313, 0.3333333333333333703, 0.3079598441704289313, 0.3333333333333333703, 0.3079598441704289313, 0.3333333333333333703, 0.3079598441704289313, 0.3333333333333333703, 0.3079598441704289313, 0.3333333333333333703, 0.3079598441704289313, 0.3333333333333333703, 0.3079598441704289313, 0.3333333333333333703, 0.3079598441704289313, 0.3333333333333333703, 0.3079598441704289313, 0.3333333333333333703),
 ( 1.000000000000000000, 0.9238795325112867385, 1.000000000000000000, 0.9238795325112867385, 1.000000000000000000, 0.9238795325112867385, 1.000000000000000000, 0.9238795325112867385, 1.000000000000000000, 0.9238795325112867385, 1.000000000000000000, 0.9238795325112867385, 1.000000000000000000, 0.9238795325112867385, 1.000000000000000000, 0.9238795325112867385, 1.000000000000000000, 0.9238795325112867385, 1.000000000000000000, 0.9238795325112867385, 1.000000000000000000, 0.9238795325112867385, 1.000000000000000000, 0.9238795325112867385, 1.000000000000000000, 0.9238795325112867385, 1.000000000000000000, 0.9238795325112867385, 1.000000000000000000, 0.9238795325112867385, 1.000000000000000000, 0.9238795325112867385, 1.000000000000000000, 0.9238795325112867385, 1.000000000000000000, 0.9238795325112867385, 1.000000000000000000, 0.9238795325112867385, 1.000000000000000000, 0.9238795325112867385, 1.000000000000000000, 0.9238795325112867385, 1.000000000000000000, 0.9238795325112867385, 1.000000000000000000, 0.9238795325112867385, 1.000000000000000000, 0.9238795325112867385, 1.000000000000000000, 0.9238795325112867385, 1.000000000000000000, 0.9238795325112867385, 1.000000000000000000, 0.9238795325112867385, 1.000000000000000000, 0.9238795325112867385, 1.000000000000000000, 0.9238795325112867385, 1.000000000000000000, 0.9238795325112867385, 1.000000000000000000, 0.9238795325112867385, 1.000000000000000000, 0.9238795325112867385, 1.000000000000000000, 0.9238795325112867385, 1.000000000000000000, 0.9238795325112867385, 1.000000000000000000, 0.9238795325112867385, 1.000000000000000000, 0.9238795325112867385, 1.000000000000000000, 0.9238795325112867385, 1.000000000000000000, 0.9238795325112867385, 1.000000000000000000, 0.9238795325112867385, 1.000000000000000000, 0.9238795325112867385, 1.000000000000000000, 0.9238795325112867385, 1.000000000000000000, 0.9238795325112867385, 1.000000000000000000, 0.9238795325112867385, 1.000000000000000000, 0.9238795325112867385, 1.000000000000000000, 0.9238795325112867385, 1.000000000000000000, 0.9238795325112867385, 1.000000000000000000, 0.9238795325112867385, 1.000000000000000000, 0.9238795325112867385, 1.000000000000000000, 0.9238795325112867385, 1.000000000000000000, 0.9238795325112867385, 1.000000000000000000, 0.9238795325112867385, 1.000000000000000000, 0.9238795325112867385, 1.000000000000000000, 0.9238795325112867385, 1.000000000000000000, 0.9238795325112867385, 1.000000000000000000, 0.9238795325112867385, 1.000000000000000000, 0.9238795325112867385, 1.000000000000000000, 0.9238795325112867385, 1.000000000000000000, 0.9238795325112867385, 1.000000000000000000, 0.9238795325112867385, 1.000000000000000000, 0.9238795325112867385, 1.000000000000000000, 0.9238795325112867385, 1.000000000000000000, 0.9238795325112867385, 1.000000000000000000, 0.9238795325112867385, 1.000000000000000000, 0.9238795325112867385, 1.000000000000000000, 0.9238795325112867385, 1.000000000000000000, 0.9238795325112867385, 1.000000000000000000, 0.9238795325112867385, 1.000000000000000000, 0.9238795325112867385, 1.000000000000000000, 0.9238795325112867385, 1.000000000000000000, 0.9238795325112867385, 1.000000000000000000, 0.9238795325112867385, 1.000000000000000000, 0.9238795325112867385, 1.000000000000000000, 0.9238795325112867385, 1.000000000000000000, 0.9238795325112867385, 1.000000000000000000, 0.9238795325112867385, 1.000000000000000000, 0.9238795325112867385, 1.000000000000000000, 0.9238795325112867385, 1.000000000000000000, 0.9238795325112867385, 1.000000000000000000, 0.9238795325112867385, 1.000000000000000000, 0.9238795325112867385, 1.000000000000000000, 0.9238795325112867385, 1.000000000000000000, 0.9238795325112867385, 1.000000000000000000, 0.9238795325112867385, 1.000000000000000000, 0.9238795325112867385, 1.000000000000000000, 0.9238795325112867385, 1.000000000000000000, 0.9238795325112867385, 1.000000000000000000, 0.9238795325112867385, 1.000000000000000000, 0.9238795325112867385, 1.000000000000000000, 0.9238795325112867385, 1.000000000000000000, 0.9238795325112867385, 1.000000000000000000, 0.9238795325112867385, 1.000000000000000000, 0.9238795325112867385, 1.000000000000000000, 0.9238795325112867385, 1.000000000000000000, 0.9238795325112867385, 1.000000000000000000, 0.9238795325112867385, 1.000000000000000000, 0.9238795325112867385, 1.000000000000000000, 0.9238795325112867385, 1.000000000000000000, 0.9238795325112867385, 1.000000000000000000, 0.9238795325112867385, 1.000000000000000000, 0.9238795325112867385, 1.000000000000000000, 0.9238795325112867385, 1.000000000000000000, 0.9238795325112867385, 1.000000000000000000, 0.9238795325112867385, 1.000000000000000000, 0.9238795325112867385, 1.000000000000000000, 0.9238795325112867385, 1.000000000000000000, 0.9238795325112867385, 1.000000000000000000, 0.9238795325112867385, 1.000000000000000000, 0.9238795325112867385, 1.000000000000000000, 0.9238795325112867385, 1.000000000000000000, 0.9238795325112867385, 1.000000000000000000, 0.9238795325112867385, 1.000000000000000000, 0.9238795325112867385, 1.000000000000000000, 0.9238795325112867385, 1.000000000000000000, 0.9238795325112867385, 1.000000000000000000, 0.9238795325112867385, 1.000000000000000000, 0.9238795325112867385, 1.000000000000000000, 0.9238795325112867385, 1.000000000000000000, 0.9238795325112867385, 1.000000000000000000, 0.9238795325112867385, 1.000000000000000000, 0.9238795325112867385, 1.000000000000000000) ) ) 
 REPRESENTATION_ITEM ( '' )  SURFACE ( )  );
#6560=CARTESIAN_POINT ( 'NONE',  ( 1.346194077712560944, 6.937500000000000000, -0.2500000000000010547 ) ) ;
#6561=CARTESIAN_POINT ( 'NONE',  ( -3.750000000000000000, 5.812500000000000888, -5.053300858899105741 ) ) ;
#6562=CARTESIAN_POINT ( 'NONE',  ( 3.749999999999999556, 9.812500000000000000, -1.946699141100892261 ) ) ;
#6565=ORIENTED_EDGE ( 'NONE', *, *, #10523, .F. ) ;
#6567=CARTESIAN_POINT ( 'NONE',  ( 0.000000000000000000, 11.50000000000000000, 0.2500000000000002220 ) ) ;
#6573=CARTESIAN_POINT ( 'NONE',  ( 1.346194077712560944, 0.9375000000000000000, -0.2500000000000011102 ) ) ;
#6575=CARTESIAN_POINT ( 'NONE',  ( -3.980102097228897738E-16, 1.084202172485504434E-16, -6.749999999999999112 ) ) ;
#6580=CARTESIAN_POINT ( 'NONE',  ( -3.249999999999999556, 10.25000000000000000, -3.499999999999999556 ) ) ;
#6583=CARTESIAN_POINT ( 'NONE',  ( 1.346194077712561166, 9.437500000000003553, -0.2500000000000011102 ) ) ;
#6586=CARTESIAN_POINT ( 'NONE',  ( -2.651650429449553314, 14.37500000000000000, -6.151650429449552426 ) ) ;
#6591=CARTESIAN_POINT ( 'NONE',  ( -3.249999999999999556, 10.18750000000000000, -2.153805922287440833 ) ) ;
#6595=CARTESIAN_POINT ( 'NONE',  ( -3.249999999999999556, 8.312500000000000000, -4.846194077712557835 ) ) ;
#6601=CARTESIAN_POINT ( 'NONE',  ( -4.592425496802573972E-16, 0.5000000000000000000, -7.249999999999999112 ) ) ;
#6602=CARTESIAN_POINT ( 'NONE',  ( -1.553300858899106629, 0.5625000000000001110, 0.2499999999999998335 ) ) ;
#6603=CARTESIAN_POINT ( 'NONE',  ( -1.346194077712559389, 0.4375000000000000555, -6.749999999999999112 ) ) ;
#6604=ORIENTED_EDGE ( 'NONE', *, *, #438, .F. ) ;
#6606=CARTESIAN_POINT ( 'NONE',  ( -2.298097038856278473, 10.12500000000000000, -1.201902961143720416 ) ) ;
#6619=CARTESIAN_POINT ( 'NONE',  ( -3.249999999999999556, 4.187500000000000000, -2.153805922287440833 ) ) ;
#6621=CARTESIAN_POINT ( 'NONE',  ( -3.750000000000000000, 1.687500000000000222, -1.946699141100893149 ) ) ;
#6624=FACE_OUTER_BOUND ( 'NONE', #13810, .T. ) ;
#6625=CARTESIAN_POINT ( 'NONE',  ( 3.749999999999998668, 6.687500000000000888, -5.053300858899107517 ) ) ;
#6628=CARTESIAN_POINT ( 'NONE',  ( -2.651650429449552870, 2.125000000000000000, -0.8483495705504462414 ) ) ;
#6633=CARTESIAN_POINT ( 'NONE',  ( 1.346194077712561166, 4.437499999999999112, -0.2500000000000011102 ) ) ;
#6637=CARTESIAN_POINT ( 'NONE',  ( -4.592425496802573972E-16, 5.999999999999999112, -7.250000000000000000 ) ) ;
#6638=CARTESIAN_POINT ( 'NONE',  ( 2.651650429449552870, 9.625000000000000000, -6.151650429449554203 ) ) ;
#6642=CARTESIAN_POINT ( 'NONE',  ( 2.651650429449552870, 12.12500000000000000, -6.151650429449555091 ) ) ;
#6651=CARTESIAN_POINT ( 'NONE',  ( 1.346194077712558279, 2.062500000000000000, -6.750000000000000888 ) ) ;
#6658=CARTESIAN_POINT ( 'NONE',  ( -2.298097038856279362, 9.875000000000000000, -5.798097038856278473 ) ) ;
#6660=CARTESIAN_POINT ( 'NONE',  ( 0.000000000000000000, 14.00000000000000000, 0.2500000000000002220 ) ) ;
#6663=CARTESIAN_POINT ( 'NONE',  ( 2.298097038856279362, 10.87500000000000178, -1.201902961143720860 ) ) ;
#6667=CARTESIAN_POINT ( 'NONE',  ( -2.298097038856278473, 9.125000000000000000, -1.201902961143720416 ) ) ;
#6674=CARTESIAN_POINT ( 'NONE',  ( 3.750000000000000000, 0.7500000000000000000, -3.500000000000000444 ) ) ;
#6675=CARTESIAN_POINT ( 'NONE',  ( -4.592425496802573972E-16, 1.000000000000000000, -7.250000000000000000 ) ) ;
#6677=CARTESIAN_POINT ( 'NONE',  ( 3.249999999999998668, 1.687500000000000000, -4.846194077712560500 ) ) ;
#6679=CARTESIAN_POINT ( 'NONE',  ( 1.346194077712558057, 12.56250000000000000, -6.750000000000000000 ) ) ;
#6680=DIRECTION ( 'NONE',  ( -1.000000000000000000, -0.000000000000000000, -0.000000000000000000 ) ) ;
#6681=CARTESIAN_POINT ( 'NONE',  ( -0.3766621274091715987, 0.5000000000000000000, -7.146945437571387671 ) ) ;
#6692=AXIS2_PLACEMENT_3D ( 'NONE', #578, #2965, #8837 ) ;
#6693=CARTESIAN_POINT ( 'NONE',  ( -3.249999999999999556, 3.312500000000000000, -4.846194077712557835 ) ) ;
#6695=CARTESIAN_POINT ( 'NONE',  ( -3.749999999999999556, 3.750000000000000444, -3.499999999999999112 ) ) ;
#6700=CARTESIAN_POINT ( 'NONE',  ( -3.249999999999999556, 0.1875000000000000278, -2.153805922287440833 ) ) ;
#6701=CARTESIAN_POINT ( 'NONE',  ( -2.651650429449552870, 6.125000000000000000, -0.8483495705504462414 ) ) ;
#6702=VECTOR ( 'NONE', #9789, 1000.000000000000000 ) ;
#6705=CARTESIAN_POINT ( 'NONE',  ( -2.651650429449553314, 3.375000000000000000, -6.151650429449552426 ) ) ;
#6709=CARTESIAN_POINT ( 'NONE',  ( -1.346194077712559167, 3.937500000000000444, -6.749999999999999112 ) ) ;
#6710=( GEOMETRIC_REPRESENTATION_CONTEXT ( 3 ) GLOBAL_UNCERTAINTY_ASSIGNED_CONTEXT ( ( #13624 ) ) GLOBAL_UNIT_ASSIGNED_CONTEXT ( ( #892, #13171, #2419 ) ) REPRESENTATION_CONTEXT ( 'NONE', 'WORKASPACE' ) );
#6712=CARTESIAN_POINT ( 'NONE',  ( -2.651650429449552870, 10.62500000000000178, -0.8483495705504467965 ) ) ;
#6713=CARTESIAN_POINT ( 'NONE',  ( 3.749999999999999556, 13.81250000000000000, -1.946699141100892261 ) ) ;
#6717=CARTESIAN_POINT ( 'NONE',  ( 2.298097038856278473, 8.625000000000000000, -5.798097038856279362 ) ) ;
#6718=CARTESIAN_POINT ( 'NONE',  ( 3.749999999999999112, 10.18750000000000533, -5.053300858899108405 ) ) ;
#6723=ORIENTED_EDGE ( 'NONE', *, *, #6290, .T. ) ;
#6727=CARTESIAN_POINT ( 'NONE',  ( 1.346194077712561166, 2.437500000000000444, -0.2500000000000011102 ) ) ;
#6734=CARTESIAN_POINT ( 'NONE',  ( -3.980102097228897738E-16, 11.00000000000000178, -6.749999999999999112 ) ) ;
#6736=CARTESIAN_POINT ( 'NONE',  ( 0.000000000000000000, 13.00000000000000178, 0.2500000000000002220 ) ) ;
#6737=EDGE_CURVE ( 'NONE', #3762, #5120, #8310, .T. ) ;
#6741=CARTESIAN_POINT ( 'NONE',  ( -3.249999999999999556, 10.25000000000000000, -3.499999999999999556 ) ) ;
#6745=CARTESIAN_POINT ( 'NONE',  ( 1.346194077712560944, 7.937500000000000888, -0.2500000000000010547 ) ) ;
#6751=CARTESIAN_POINT ( 'NONE',  ( 3.749999999999998668, 2.687500000000000888, -5.053300858899107517 ) ) ;
#6753=CARTESIAN_POINT ( 'NONE',  ( -3.249999999999999556, 13.75000000000000000, -3.500000000000000000 ) ) ;
#6756=CARTESIAN_POINT ( 'NONE',  ( 1.346194077712558057, 10.56250000000000000, -6.750000000000000000 ) ) ;
#6768=CARTESIAN_POINT ( 'NONE',  ( -3.249999999999999556, 9.250000000000000000, -3.499999999999999556 ) ) ;
#6770=CARTESIAN_POINT ( 'NONE',  ( -2.298097038856278918, 4.375000000000000000, -5.798097038856277585 ) ) ;
#6772=CARTESIAN_POINT ( 'NONE',  ( 3.749999999999999112, 0.1875000000000000833, -5.053300858899108405 ) ) ;
#6776=CARTESIAN_POINT ( 'NONE',  ( 3.249999999999999556, 0.7500000000000000000, -3.500000000000000000 ) ) ;
#6777=CARTESIAN_POINT ( 'NONE',  ( -3.749999999999999556, 5.312500000000001776, -5.053300858899104853 ) ) ;
#6788=CARTESIAN_POINT ( 'NONE',  ( 3.249999999999999556, 9.250000000000001776, -3.500000000000000000 ) ) ;
#6790=CARTESIAN_POINT ( 'NONE',  ( 1.553300858899109071, 10.43750000000000178, 0.2499999999999989175 ) ) ;
#6791=CARTESIAN_POINT ( 'NONE',  ( 0.000000000000000000, 15.00000000000000000, 0.2500000000000002220 ) ) ;
#6794=CARTESIAN_POINT ( 'NONE',  ( 2.298097038856278473, 7.625000000000000000, -5.798097038856279362 ) ) ;
#6795=CARTESIAN_POINT ( 'NONE',  ( -3.249999999999999112, -0.3124999999999999445, -2.153805922287440833 ) ) ;
#6801=CARTESIAN_POINT ( 'NONE',  ( -3.249999999999999112, 1.687500000000000222, -2.153805922287440833 ) ) ;
#6807=CARTESIAN_POINT ( 'NONE',  ( -2.298097038856278029, 13.62500000000000000, -1.201902961143720638 ) ) ;
#6809=CARTESIAN_POINT ( 'NONE',  ( 2.651650429449552870, 2.125000000000000000, -6.151650429449555091 ) ) ;
#6814=CARTESIAN_POINT ( 'NONE',  ( -3.249999999999999556, 9.312499999999998224, -4.846194077712557835 ) ) ;
#6821=CARTESIAN_POINT ( 'NONE',  ( 3.749999999999999112, 0.8125000000000001110, -1.946699141100892039 ) ) ;
#6822=CARTESIAN_POINT ( 'NONE',  ( -1.346194077712559167, 13.93750000000000000, -6.749999999999999112 ) ) ;
#6825=CARTESIAN_POINT ( 'NONE',  ( -1.346194077712558945, 1.562500000000000222, -0.2500000000000002220 ) ) ;
#6828=CARTESIAN_POINT ( 'NONE',  ( -3.249999999999999556, 3.312500000000000000, -4.846194077712557835 ) ) ;
#6834=CARTESIAN_POINT ( 'NONE',  ( 1.346194077712560944, 10.93750000000000178, -0.2500000000000011102 ) ) ;
#6837=CARTESIAN_POINT ( 'NONE',  ( 1.553300858899109516, 11.43750000000000178, 0.2499999999999993616 ) ) ;
#6839=CARTESIAN_POINT ( 'NONE',  ( -1.553300858899106629, 0.5625000000000003331, 0.2500000000000002220 ) ) ;
#6840=CIRCLE ( 'NONE', #3627, 0.2500000000000002220 ) ;
#6841=CARTESIAN_POINT ( 'NONE',  ( 3.249999999999999556, 5.250000000000000000, -3.500000000000000000 ) ) ;
#6843=EDGE_CURVE ( 'NONE', #7860, #11175, #4306, .T. ) ;
#6845=CARTESIAN_POINT ( 'NONE',  ( -1.346194077712559389, 3.062500000000000000, -0.2500000000000002220 ) ) ;
#6846=CARTESIAN_POINT ( 'NONE',  ( -1.553300858899106629, 7.062500000000000000, 0.2500000000000002220 ) ) ;
#6855=CARTESIAN_POINT ( 'NONE',  ( -3.249999999999999556, 8.750000000000001776, -3.500000000000000000 ) ) ;
#6859=CARTESIAN_POINT ( 'NONE',  ( -1.553300858899106629, 9.562500000000000000, 0.2499999999999998335 ) ) ;
#6860=CARTESIAN_POINT ( 'NONE',  ( -1.553300858899107073, 13.43750000000000000, -7.250000000000000000 ) ) ;
#6863=CARTESIAN_POINT ( 'NONE',  ( 2.651650429449552870, 13.12499999999999822, -6.151650429449555091 ) ) ;
#6869=CARTESIAN_POINT ( 'NONE',  ( -3.249999999999999556, 4.187500000000000000, -2.153805922287440833 ) ) ;
#6871=CARTESIAN_POINT ( 'NONE',  ( -3.980102097228897738E-16, 2.000000000000000000, -6.749999999999999112 ) ) ;
#6878=CARTESIAN_POINT ( 'NONE',  ( -1.346194077712559167, 10.93750000000000355, -6.749999999999999112 ) ) ;
#6880=CARTESIAN_POINT ( 'NONE',  ( -2.651650429449553314, 2.875000000000000000, -6.151650429449552426 ) ) ;
#6885=CARTESIAN_POINT ( 'NONE',  ( 3.249999999999999112, 9.812500000000000000, -2.153805922287439945 ) ) ;
#6887=LINE ( 'NONE', #1026, #14077 ) ;
#6891=CARTESIAN_POINT ( 'NONE',  ( 1.553300858899105963, 6.562500000000000000, -7.250000000000000888 ) ) ;
#6892=CARTESIAN_POINT ( 'NONE',  ( 1.346194077712558279, 15.06250000000000178, -6.750000000000000888 ) ) ;
#6895=CARTESIAN_POINT ( 'NONE',  ( 3.249999999999998668, 14.68750000000000000, -4.846194077712560500 ) ) ;
#6900=CARTESIAN_POINT ( 'NONE',  ( 2.298097038856278473, 3.625000000000000000, -5.798097038856279362 ) ) ;
#6907=CARTESIAN_POINT ( 'NONE',  ( 3.249999999999999112, 12.81250000000000178, -2.153805922287439945 ) ) ;
#6910=CARTESIAN_POINT ( 'NONE',  ( 2.651650429449552870, 8.125000000000000000, -6.151650429449555091 ) ) ;
#6912=CARTESIAN_POINT ( 'NONE',  ( -1.553300858899106629, 6.562500000000000888, 0.2500000000000002220 ) ) ;
#6913=CARTESIAN_POINT ( 'NONE',  ( -1.346194077712559167, 4.937500000000000888, -6.749999999999999112 ) ) ;
#6917=CARTESIAN_POINT ( 'NONE',  ( -2.298097038856278918, 1.375000000000000000, -5.798097038856277585 ) ) ;
#6919=CARTESIAN_POINT ( 'NONE',  ( 1.553300858899105963, 4.562500000000000888, -7.250000000000000888 ) ) ;
#6930=CARTESIAN_POINT ( 'NONE',  ( 3.249999999999998224, 8.187500000000000000, -4.846194077712561388 ) ) ;
#6933=CARTESIAN_POINT ( 'NONE',  ( -1.553300858899107073, 9.937500000000001776, -7.249999999999999112 ) ) ;
#6934=CARTESIAN_POINT ( 'NONE',  ( 1.553300858899108849, 13.93750000000000000, 0.2499999999999993616 ) ) ;
#6937=CARTESIAN_POINT ( 'NONE',  ( -4.592425496802573972E-16, 13.00000000000000000, -7.250000000000000000 ) ) ;
#6946=CARTESIAN_POINT ( 'NONE',  ( 1.346194077712558279, 4.562500000000001776, -6.750000000000000000 ) ) ;
#6948=CARTESIAN_POINT ( 'NONE',  ( -3.249999999999999556, 3.750000000000000444, -3.500000000000000000 ) ) ;
#6954=CARTESIAN_POINT ( 'NONE',  ( 3.249999999999998224, 11.31250000000000355, -2.153805922287439945 ) ) ;
#6958=CARTESIAN_POINT ( 'NONE',  ( 3.749999999999999556, 2.249999999999999556, -3.500000000000000444 ) ) ;
#6966=CARTESIAN_POINT ( 'NONE',  ( -3.980102097228897245E-16, 14.50000000000000000, -6.749999999999999112 ) ) ;
#6972=CARTESIAN_POINT ( 'NONE',  ( -4.592425496802573972E-16, 4.500000000000000888, -7.249999999999999112 ) ) ;
#6973=CARTESIAN_POINT ( 'NONE',  ( -2.651650429449552870, 4.624999999999999112, -0.8483495705504467965 ) ) ;
#6977=CARTESIAN_POINT ( 'NONE',  ( 3.249999999999999112, 13.81250000000000000, -2.153805922287439945 ) ) ;
#6981=CARTESIAN_POINT ( 'NONE',  ( -2.298097038856278473, 2.125000000000000000, -1.201902961143720416 ) ) ;
#6988=CARTESIAN_POINT ( 'NONE',  ( -2.298097038856278473, 10.12500000000000000, -1.201902961143720416 ) ) ;
#6992=CARTESIAN_POINT ( 'NONE',  ( -2.651650429449553314, 4.875000000000000000, -6.151650429449552426 ) ) ;
#6993=CARTESIAN_POINT ( 'NONE',  ( 3.249999999999998224, 7.187500000000000888, -4.846194077712561388 ) ) ;
#6996=CARTESIAN_POINT ( 'NONE',  ( -2.298097038856278473, 2.125000000000000000, -1.201902961143720416 ) ) ;
#6997=CARTESIAN_POINT ( 'NONE',  ( 3.749999999999999112, 9.812500000000000000, -1.946699141100892039 ) ) ;
#7001=DIRECTION ( 'NONE',  ( -0.000000000000000000, -1.000000000000000000, -0.000000000000000000 ) ) ;
#7005=VECTOR ( 'NONE', #15062, 1000.000000000000000 ) ;
#7006=CARTESIAN_POINT ( 'NONE',  ( 2.298097038856278029, 7.124999999999999112, -5.798097038856279362 ) ) ;
#7007=CARTESIAN_POINT ( 'NONE',  ( -4.592425496802573972E-16, 8.999999999999998224, -7.250000000000000000 ) ) ;
#7011=CARTESIAN_POINT ( 'NONE',  ( 2.298097038856279362, 0.3750000000000001110, -1.201902961143720860 ) ) ;
#7015=CARTESIAN_POINT ( 'NONE',  ( 3.249999999999999556, 14.75000000000000178, -3.500000000000000000 ) ) ;
#7016=CARTESIAN_POINT ( 'NONE',  ( -0.3766621274091715987, -0.2500000000000000000, 0.1491815183709511716 ) ) ;
#7019=CARTESIAN_POINT ( 'NONE',  ( -1.346194077712558945, 1.062500000000000222, -0.2500000000000002220 ) ) ;
#7021=CARTESIAN_POINT ( 'NONE',  ( -1.346194077712558945, 8.562500000000000000, -0.2500000000000002220 ) ) ;
#7026=EDGE_CURVE ( 'NONE', #7860, #2992, #3597, .T. ) ;
#7027=CARTESIAN_POINT ( 'NONE',  ( -2.298097038856278473, 1.125000000000000222, -1.201902961143720416 ) ) ;
#7028=CARTESIAN_POINT ( 'NONE',  ( 3.249999999999998224, 13.18750000000000000, -4.846194077712561388 ) ) ;
#7030=CARTESIAN_POINT ( 'NONE',  ( -2.651650429449552870, 1.625000000000000000, -0.8483495705504463524 ) ) ;
#7034=CARTESIAN_POINT ( 'NONE',  ( -3.249999999999999556, 11.18749999999999822, -2.153805922287440833 ) ) ;
#7040=CARTESIAN_POINT ( 'NONE',  ( 2.651650429449553759, 3.875000000000000000, -0.8483495705504471296 ) ) ;
#7041=CARTESIAN_POINT ( 'NONE',  ( -3.750000000000000000, 2.687500000000000888, -1.946699141100893149 ) ) ;
#7044=EDGE_CURVE ( 'NONE', #7693, #4358, #7755, .T. ) ;
#7046=CARTESIAN_POINT ( 'NONE',  ( 1.346194077712558279, 1.062500000000000444, -6.750000000000000888 ) ) ;
#7050=CARTESIAN_POINT ( 'NONE',  ( -3.980102097228897245E-16, 3.500000000000000000, -6.749999999999999112 ) ) ;
#7055=CARTESIAN_POINT ( 'NONE',  ( 0.000000000000000000, 14.00000000000000000, -0.2500000000000002220 ) ) ;
#7059=CARTESIAN_POINT ( 'NONE',  ( 2.651650429449554203, 7.375000000000000000, -0.8483495705504471296 ) ) ;
#7060=CARTESIAN_POINT ( 'NONE',  ( 0.000000000000000000, 8.500000000000000000, -0.2500000000000002220 ) ) ;
#7063=CARTESIAN_POINT ( 'NONE',  ( -1.346194077712559389, 4.062500000000000000, -0.2500000000000002220 ) ) ;
#7065=CARTESIAN_POINT ( 'NONE',  ( 3.749999999999999112, 10.81250000000000178, -1.946699141100892039 ) ) ;
#7073=CARTESIAN_POINT ( 'NONE',  ( -4.592425496802573972E-16, 13.00000000000000000, -7.250000000000000000 ) ) ;
#7077=CARTESIAN_POINT ( 'NONE',  ( 0.000000000000000000, 1.500000000000000222, -0.2500000000000002220 ) ) ;
#7083=CARTESIAN_POINT ( 'NONE',  ( -2.298097038856278473, 1.125000000000000222, -1.201902961143720416 ) ) ;
#7086=CARTESIAN_POINT ( 'NONE',  ( 0.000000000000000000, 5.500000000000000888, -0.2500000000000002220 ) ) ;
#7092=CARTESIAN_POINT ( 'NONE',  ( 3.749999999999999112, 3.312500000000000000, -1.946699141100893149 ) ) ;
#7093=CARTESIAN_POINT ( 'NONE',  ( -3.750000000000000000, 4.187500000000000000, -1.946699141100892927 ) ) ;
#7095=CARTESIAN_POINT ( 'NONE',  ( -4.592425496802573972E-16, 4.000000000000000888, -7.250000000000000000 ) ) ;
#7099=CARTESIAN_POINT ( 'NONE',  ( 3.249999999999999556, 10.75000000000000000, -3.500000000000000000 ) ) ;
#7102=CARTESIAN_POINT ( 'NONE',  ( -1.346194077712559389, 12.06250000000000000, -0.2500000000000002220 ) ) ;
#7107=DIRECTION ( 'NONE',  ( 0.000000000000000000, -0.000000000000000000, -1.000000000000000000 ) ) ;
#7108=CARTESIAN_POINT ( 'NONE',  ( -1.553300858899106629, 6.062500000000000000, 0.2500000000000002220 ) ) ;
#7109=CARTESIAN_POINT ( 'NONE',  ( -3.750000000000000000, 5.687500000000000888, -1.946699141100893149 ) ) ;
#7112=CARTESIAN_POINT ( 'NONE',  ( 0.000000000000000000, 0.4999999999999999445, -0.2500000000000002220 ) ) ;
#7115=MANIFOLD_SOLID_BREP ( 'Saliente-Extruir1', #14998 ) ;
#7116=CARTESIAN_POINT ( 'NONE',  ( 0.000000000000000000, 5.000000000000000000, -0.2500000000000002220 ) ) ;
#7127=CARTESIAN_POINT ( 'NONE',  ( -3.750000000000000000, 6.687500000000000888, -1.946699141100893149 ) ) ;
#7128=CARTESIAN_POINT ( 'NONE',  ( 3.249999999999998224, 5.187500000000001776, -4.846194077712561388 ) ) ;
#7131=CARTESIAN_POINT ( 'NONE',  ( -2.298097038856278473, 4.125000000000000000, -1.201902961143720416 ) ) ;
#7133=VECTOR ( 'NONE', #1654, 1000.000000000000000 ) ;
#7140=EDGE_CURVE ( 'NONE', #2776, #6060, #1, .T. ) ;
#7142=ORIENTED_EDGE ( 'NONE', *, *, #10732, .T. ) ;
#7145=CARTESIAN_POINT ( 'NONE',  ( 3.749999999999999112, 13.31250000000000178, -1.946699141100893149 ) ) ;
#7150=CARTESIAN_POINT ( 'NONE',  ( 2.298097038856279362, 4.375000000000000888, -1.201902961143720860 ) ) ;
#7160=CARTESIAN_POINT ( 'NONE',  ( -3.249999999999999556, 3.312500000000000000, -4.846194077712557835 ) ) ;
#7163=CARTESIAN_POINT ( 'NONE',  ( 3.249999999999998224, 7.312500000000001776, -2.153805922287439945 ) ) ;
#7169=CARTESIAN_POINT ( 'NONE',  ( -2.298097038856278918, 2.375000000000000000, -5.798097038856277585 ) ) ;
#7170=CARTESIAN_POINT ( 'NONE',  ( -3.750000000000000000, 0.8124999999999997780, -5.053300858899105741 ) ) ;
#7171=CARTESIAN_POINT ( 'NONE',  ( -4.592425496802573972E-16, 6.500000000000000888, -7.249999999999999112 ) ) ;
#7173=CARTESIAN_POINT ( 'NONE',  ( -2.651650429449553314, 7.874999999999999112, -6.151650429449552426 ) ) ;
#7175=CARTESIAN_POINT ( 'NONE',  ( 0.000000000000000000, 1.530808498934191509E-17, 0.000000000000000000 ) ) ;
#7178=CARTESIAN_POINT ( 'NONE',  ( 3.249999999999999112, 13.81250000000000000, -2.153805922287439945 ) ) ;
#7182=CARTESIAN_POINT ( 'NONE',  ( 2.651650429449554203, 8.375000000000000000, -0.8483495705504471296 ) ) ;
#7186=CARTESIAN_POINT ( 'NONE',  ( -3.750000000000000000, 4.250000000000000000, -3.499999999999999112 ) ) ;
#7187=CARTESIAN_POINT ( 'NONE',  ( 3.749999999999999556, 2.249999999999999556, -3.500000000000000444 ) ) ;
#7192=B_SPLINE_CURVE_WITH_KNOTS ( 'NONE', 3,
 ( #10035, #9026, #4169, #8873 ),
 .UNSPECIFIED., .F., .F.,
 ( 4, 4 ),
 ( 0.000000000000000000, 0.0003777938110651892596 ),
 .UNSPECIFIED. ) ;
#7194=CARTESIAN_POINT ( 'NONE',  ( -3.249999999999999112, 4.812500000000000000, -4.846194077712558723 ) ) ;
#7198=CARTESIAN_POINT ( 'NONE',  ( -3.249999999999999556, 6.187500000000000888, -2.153805922287440833 ) ) ;
#7204=ORIENTED_EDGE ( 'NONE', *, *, #6737, .T. ) ;
#7206=CARTESIAN_POINT ( 'NONE',  ( -2.298097038856278918, 14.37500000000000000, -5.798097038856277585 ) ) ;
#7210=CARTESIAN_POINT ( 'NONE',  ( -2.651650429449552870, 6.625000000000000888, -0.8483495705504463524 ) ) ;
#7212=CARTESIAN_POINT ( 'NONE',  ( 0.000000000000000000, 9.500000000000000000, -0.2500000000000002220 ) ) ;
#7216=CARTESIAN_POINT ( 'NONE',  ( 3.249999999999998668, 8.687500000000000000, -4.846194077712560500 ) ) ;
#7229=VECTOR ( 'NONE', #11222, 1000.000000000000000 ) ;
#7232=CARTESIAN_POINT ( 'NONE',  ( -2.651650429449552870, 14.87500000000000355, -6.151650429449552426 ) ) ;
#7238=CARTESIAN_POINT ( 'NONE',  ( 2.298097038856279362, 3.375000000000000444, -1.201902961143720860 ) ) ;
#7246=CARTESIAN_POINT ( 'NONE',  ( 0.000000000000000000, 6.000000000000000000, -0.2500000000000002220 ) ) ;
#7248=CARTESIAN_POINT ( 'NONE',  ( 1.346194077712558057, 12.56250000000000000, -6.750000000000000000 ) ) ;
#7249=CARTESIAN_POINT ( 'NONE',  ( 2.298097038856279362, 6.375000000000000888, -1.201902961143720860 ) ) ;
#7253=CARTESIAN_POINT ( 'NONE',  ( 2.298097038856278473, 2.625000000000000000, -5.798097038856279362 ) ) ;
#7255=CARTESIAN_POINT ( 'NONE',  ( 3.749999999999999556, 2.249999999999999556, -3.500000000000000444 ) ) ;
#7257=CARTESIAN_POINT ( 'NONE',  ( -2.651650429449553314, 4.375000000000000000, -6.151650429449552426 ) ) ;
#7260=CARTESIAN_POINT ( 'NONE',  ( 1.553300858899109516, 6.437500000000000888, 0.2499999999999993616 ) ) ;
#7265=CARTESIAN_POINT ( 'NONE',  ( -2.298097038856278918, 13.37500000000000000, -5.798097038856277585 ) ) ;
#7269=CARTESIAN_POINT ( 'NONE',  ( -2.651650429449552870, 10.62500000000000000, -0.8483495705504463524 ) ) ;
#7273=CARTESIAN_POINT ( 'NONE',  ( -4.592425496802573972E-16, 10.50000000000000000, -7.249999999999999112 ) ) ;
#7274=CARTESIAN_POINT ( 'NONE',  ( -2.651650429449552870, 4.875000000000000000, -6.151650429449552426 ) ) ;
#7278=CARTESIAN_POINT ( 'NONE',  ( -2.298097038856278029, 4.624999999999999112, -1.201902961143720638 ) ) ;
#7282=CARTESIAN_POINT ( 'NONE',  ( 0.000000000000000000, 7.000000000000000000, -0.2500000000000002220 ) ) ;
#7288=CARTESIAN_POINT ( 'NONE',  ( 1.346194077712560944, 13.93750000000000000, -0.2500000000000011102 ) ) ;
#7292=CARTESIAN_POINT ( 'NONE',  ( 3.749999999999999112, 13.31250000000000178, -1.946699141100893149 ) ) ;
#7293=CARTESIAN_POINT ( 'NONE',  ( 3.249999999999998224, 6.187500000000001776, -4.846194077712561388 ) ) ;
#7294=CARTESIAN_POINT ( 'NONE',  ( 3.249999999999998224, 11.31250000000000000, -2.153805922287439945 ) ) ;
#7297=CARTESIAN_POINT ( 'NONE',  ( 1.346194077712558057, 5.562500000000000000, -6.750000000000000000 ) ) ;
#7306=CARTESIAN_POINT ( 'NONE',  ( -3.249999999999999556, 9.312499999999998224, -4.846194077712557835 ) ) ;
#7307=CARTESIAN_POINT ( 'NONE',  ( -2.298097038856278473, 2.125000000000000000, -1.201902961143720416 ) ) ;
#7309=CARTESIAN_POINT ( 'NONE',  ( -1.553300858899107073, 13.93750000000000000, -7.249999999999999112 ) ) ;
#7313=CARTESIAN_POINT ( 'NONE',  ( 2.298097038856278029, 2.125000000000000000, -5.798097038856279362 ) ) ;
#7317=FACE_OUTER_BOUND ( 'NONE', #2728, .T. ) ;
#7322=CARTESIAN_POINT ( 'NONE',  ( -2.298097038856278918, 5.375000000000000000, -5.798097038856277585 ) ) ;
#7325=CARTESIAN_POINT ( 'NONE',  ( 3.249999999999999112, 12.81250000000000000, -2.153805922287439945 ) ) ;
#7326=CARTESIAN_POINT ( 'NONE',  ( -2.298097038856278029, 6.625000000000000888, -1.201902961143720638 ) ) ;
#7332=CARTESIAN_POINT ( 'NONE',  ( -3.750000000000000000, 1.812499999999999778, -5.053300858899105741 ) ) ;
#7333=CARTESIAN_POINT ( 'NONE',  ( 2.651650429449553759, 3.875000000000000000, -0.8483495705504471296 ) ) ;
#7335=CARTESIAN_POINT ( 'NONE',  ( -3.750000000000000000, 5.687500000000000888, -1.946699141100893149 ) ) ;
#7339=CARTESIAN_POINT ( 'NONE',  ( 1.346194077712560944, 10.93750000000000000, -0.2500000000000010547 ) ) ;
#7344=CARTESIAN_POINT ( 'NONE',  ( 0.3766621274091715987, 0.2956834184403337451, -6.863050255469942407 ) ) ;
#7346=CARTESIAN_POINT ( 'NONE',  ( -2.651650429449552870, 9.624999999999998224, -0.8483495705504463524 ) ) ;
#7350=CARTESIAN_POINT ( 'NONE',  ( 1.553300858899108849, 7.937500000000000888, 0.2499999999999993616 ) ) ;
#7351=CARTESIAN_POINT ( 'NONE',  ( 2.651650429449553314, 9.374999999999998224, -0.8483495705504476847 ) ) ;
#7355=CARTESIAN_POINT ( 'NONE',  ( -2.298097038856279362, 5.875000000000000888, -5.798097038856278473 ) ) ;
#7356=CARTESIAN_POINT ( 'NONE',  ( -3.749999999999999556, 11.31249999999999822, -5.053300858899104853 ) ) ;
#7360=CARTESIAN_POINT ( 'NONE',  ( -3.249999999999999556, 9.250000000000000000, -3.499999999999999556 ) ) ;
#7365=CARTESIAN_POINT ( 'NONE',  ( -1.346194077712559167, 13.43750000000000000, -6.749999999999999112 ) ) ;
#7369=CARTESIAN_POINT ( 'NONE',  ( -3.750000000000000000, 11.68749999999999822, -1.946699141100893149 ) ) ;
#7370=CARTESIAN_POINT ( 'NONE',  ( -3.249999999999999112, 11.81250000000000178, -4.846194077712558723 ) ) ;
#7371=CARTESIAN_POINT ( 'NONE',  ( 1.346194077712558279, 10.06250000000000000, -6.750000000000000888 ) ) ;
#7374=CARTESIAN_POINT ( 'NONE',  ( 1.346194077712558057, 7.562500000000000000, -6.750000000000000000 ) ) ;
#7381=CARTESIAN_POINT ( 'NONE',  ( -2.298097038856278918, 2.375000000000000000, -5.798097038856277585 ) ) ;
#7382=CARTESIAN_POINT ( 'NONE',  ( -2.651650429449553314, 14.37500000000000000, -6.151650429449552426 ) ) ;
#7384=CARTESIAN_POINT ( 'NONE',  ( -4.592425496802573972E-16, 15.00000000000000178, -7.250000000000000000 ) ) ;
#7388=CARTESIAN_POINT ( 'NONE',  ( -3.249999999999999112, 2.812500000000000444, -4.846194077712558723 ) ) ;
#7396=CARTESIAN_POINT ( 'NONE',  ( -3.980102097228897245E-16, 6.500000000000000888, -6.749999999999999112 ) ) ;
#7398=CARTESIAN_POINT ( 'NONE',  ( 3.249999999999998668, 13.68750000000000000, -4.846194077712560500 ) ) ;
#7399=CARTESIAN_POINT ( 'NONE',  ( 2.298097038856278029, 11.12500000000000000, -5.798097038856279362 ) ) ;
#7404=CARTESIAN_POINT ( 'NONE',  ( 3.249999999999999112, 3.812500000000000000, -2.153805922287439945 ) ) ;
#7405=CARTESIAN_POINT ( 'NONE',  ( -2.651650429449552870, 0.6249999999999998890, -0.8483495705504467965 ) ) ;
#7408=CARTESIAN_POINT ( 'NONE',  ( 3.749999999999999112, 3.687500000000000444, -5.053300858899108405 ) ) ;
#7411=CARTESIAN_POINT ( 'NONE',  ( 1.553300858899109516, 7.437500000000000000, 0.2499999999999993616 ) ) ;
#7419=CIRCLE ( 'NONE', #6692, 0.2500000000000002220 ) ;
#7423=CARTESIAN_POINT ( 'NONE',  ( -3.749999999999999556, 13.75000000000000000, -3.499999999999999112 ) ) ;
#7427=CARTESIAN_POINT ( 'NONE',  ( 3.749999999999998668, 9.687500000000000000, -5.053300858899107517 ) ) ;
#7428=CARTESIAN_POINT ( 'NONE',  ( 1.553300858899105963, 8.062500000000001776, -7.249999999999999112 ) ) ;
#7432=CARTESIAN_POINT ( 'NONE',  ( 3.249999999999999556, 3.250000000000000000, -3.500000000000000000 ) ) ;
#7435=CARTESIAN_POINT ( 'NONE',  ( 3.749999999999998668, 10.68750000000000000, -5.053300858899107517 ) ) ;
#7437=ADVANCED_FACE ( 'NONE', ( #9523 ), #15116, .F. ) ;
#7441=CARTESIAN_POINT ( 'NONE',  ( -2.298097038856278473, 7.125000000000000000, -1.201902961143720416 ) ) ;
#7447=CARTESIAN_POINT ( 'NONE',  ( 0.3766621274091715987, 0.5000000000000000000, 0.1491815183709511716 ) ) ;
#7453=CARTESIAN_POINT ( 'NONE',  ( 1.553300858899109071, 12.43750000000000000, 0.2499999999999989175 ) ) ;
#7454=CARTESIAN_POINT ( 'NONE',  ( 2.298097038856278029, 12.12500000000000000, -5.798097038856279362 ) ) ;
#7455=CARTESIAN_POINT ( 'NONE',  ( -2.298097038856279362, 9.875000000000000000, -5.798097038856278473 ) ) ;
#7458=CARTESIAN_POINT ( 'NONE',  ( 3.249999999999998668, 6.687500000000000888, -4.846194077712560500 ) ) ;
#7467=CARTESIAN_POINT ( 'NONE',  ( 0.000000000000000000, 1.000000000000000000, -0.2500000000000002220 ) ) ;
#7468=CARTESIAN_POINT ( 'NONE',  ( 1.553300858899108849, 11.93750000000000000, 0.2499999999999993616 ) ) ;
#7471=CARTESIAN_POINT ( 'NONE',  ( -3.749999999999999556, 2.187500000000000444, -1.946699141100892927 ) ) ;
#7482=CARTESIAN_POINT ( 'NONE',  ( 3.249999999999999112, 7.812500000000000000, -2.153805922287439945 ) ) ;
#7484=CARTESIAN_POINT ( 'NONE',  ( -3.249999999999999556, 12.31250000000000000, -4.846194077712557835 ) ) ;
#7485=CARTESIAN_POINT ( 'NONE',  ( -2.298097038856279362, 10.87499999999999822, -5.798097038856278473 ) ) ;
#7489=CARTESIAN_POINT ( 'NONE',  ( -3.249999999999999556, 5.312500000000001776, -4.846194077712557835 ) ) ;
#7490=CARTESIAN_POINT ( 'NONE',  ( 1.553300858899109071, 4.437499999999999112, 0.2499999999999989175 ) ) ;
#7491=CARTESIAN_POINT ( 'NONE',  ( 3.749999999999999556, 7.812500000000000000, -1.946699141100892261 ) ) ;
#7493=CARTESIAN_POINT ( 'NONE',  ( -3.749999999999999556, 4.750000000000000888, -3.499999999999999112 ) ) ;
#7504=CARTESIAN_POINT ( 'NONE',  ( 3.249999999999999556, 0.2500000000000001110, -3.500000000000000000 ) ) ;
#7506=DIRECTION ( 'NONE',  ( 0.000000000000000000, 0.000000000000000000, 1.000000000000000000 ) ) ;
#7508=CARTESIAN_POINT ( 'NONE',  ( 2.651650429449552870, 9.625000000000000000, -6.151650429449554203 ) ) ;
#7510=CARTESIAN_POINT ( 'NONE',  ( 3.749999999999999556, 8.250000000000000000, -3.500000000000000444 ) ) ;
#7513=CARTESIAN_POINT ( 'NONE',  ( 2.298097038856279362, 6.374999999999999112, -1.201902961143720860 ) ) ;
#7514=CARTESIAN_POINT ( 'NONE',  ( -2.651650429449552870, 11.12500000000000000, -0.8483495705504462414 ) ) ;
#7518=CARTESIAN_POINT ( 'NONE',  ( 1.346194077712560944, 9.937499999999998224, -0.2500000000000010547 ) ) ;
#7530=CARTESIAN_POINT ( 'NONE',  ( -4.592425496802573972E-16, 14.00000000000000000, -7.250000000000000000 ) ) ;
#7531=CARTESIAN_POINT ( 'NONE',  ( 3.249999999999999556, 13.25000000000000178, -3.500000000000000000 ) ) ;
#7532=EDGE_CURVE ( 'NONE', #559, #1425, #4809, .T. ) ;
#7533=CARTESIAN_POINT ( 'NONE',  ( -1.346194077712558945, 11.56250000000000178, -0.2500000000000002220 ) ) ;
#7536=CARTESIAN_POINT ( 'NONE',  ( 0.000000000000000000, 9.000000000000001776, -0.2500000000000002220 ) ) ;
#7544=CARTESIAN_POINT ( 'NONE',  ( 1.346194077712558057, 1.562500000000000000, -6.750000000000000000 ) ) ;
#7545=CARTESIAN_POINT ( 'NONE',  ( -3.750000000000000000, -0.3124999999999999445, -1.946699141100893149 ) ) ;
#7550=CARTESIAN_POINT ( 'NONE',  ( 3.750000000000000000, 0.7500000000000000000, -3.500000000000000444 ) ) ;
#7553=CARTESIAN_POINT ( 'NONE',  ( 2.651650429449552870, 0.6250000000000000000, -6.151650429449554203 ) ) ;
#7558=CARTESIAN_POINT ( 'NONE',  ( 3.249999999999999556, 8.750000000000000000, -3.500000000000000000 ) ) ;
#7560=CARTESIAN_POINT ( 'NONE',  ( -3.249999999999999556, 14.31250000000000000, -4.846194077712557835 ) ) ;
#7561=CARTESIAN_POINT ( 'NONE',  ( 2.298097038856278029, 12.12500000000000000, -5.798097038856279362 ) ) ;
#7564=CARTESIAN_POINT ( 'NONE',  ( 2.298097038856278473, 6.625000000000000000, -5.798097038856279362 ) ) ;
#7565=CARTESIAN_POINT ( 'NONE',  ( 0.000000000000000000, 3.500000000000000000, 0.2499999999999998057 ) ) ;
#7566=CARTESIAN_POINT ( 'NONE',  ( -2.651650429449553314, 10.37500000000000000, -6.151650429449552426 ) ) ;
#7569=CARTESIAN_POINT ( 'NONE',  ( 1.553300858899105963, 10.06250000000000000, -7.250000000000000888 ) ) ;
#7575=DESIGN_CONTEXT ( 'detailed design', #15111, 'design' ) ;
#7577=CARTESIAN_POINT ( 'NONE',  ( -3.249999999999999556, 0.7500000000000001110, -3.500000000000000000 ) ) ;
#7581=CARTESIAN_POINT ( 'NONE',  ( 1.553300858899105963, 7.562500000000000000, -7.250000000000000888 ) ) ;
#7582=CARTESIAN_POINT ( 'NONE',  ( 2.651650429449552870, 10.12500000000000000, -6.151650429449553314 ) ) ;
#7584=CARTESIAN_POINT ( 'NONE',  ( 1.346194077712558279, 9.062500000000003553, -6.750000000000000888 ) ) ;
#7586=CARTESIAN_POINT ( 'NONE',  ( -1.553300858899107295, 14.43750000000000000, -7.250000000000000000 ) ) ;
#7591=CARTESIAN_POINT ( 'NONE',  ( -3.249999999999999556, 13.31250000000000000, -4.846194077712557835 ) ) ;
#7596=CARTESIAN_POINT ( 'NONE',  ( 0.000000000000000000, 15.00000000000000000, 0.000000000000000000 ) ) ;
#7599=CARTESIAN_POINT ( 'NONE',  ( -0.3766621274091715987, 0.2613176957160640579, -6.863050255469941519 ) ) ;
#7600=CARTESIAN_POINT ( 'NONE',  ( -3.750000000000000000, 13.68750000000000178, -1.946699141100893149 ) ) ;
#7601=CARTESIAN_POINT ( 'NONE',  ( -2.298097038856279362, 11.87500000000000000, -5.798097038856278473 ) ) ;
#7603=CARTESIAN_POINT ( 'NONE',  ( 1.346194077712560944, 1.937500000000000000, -0.2500000000000010547 ) ) ;
#7606=CARTESIAN_POINT ( 'NONE',  ( 3.249999999999998668, 9.687500000000000000, -4.846194077712560500 ) ) ;
#7614=ORIENTED_EDGE ( 'NONE', *, *, #6843, .T. ) ;
#7615=CARTESIAN_POINT ( 'NONE',  ( -3.249999999999999112, 13.68750000000000178, -2.153805922287440833 ) ) ;
#7616=CARTESIAN_POINT ( 'NONE',  ( -1.553300858899106629, -0.4374999999999998890, 0.2500000000000002220 ) ) ;
#7620=CARTESIAN_POINT ( 'NONE',  ( 2.651650429449552870, 2.625000000000000000, -6.151650429449554203 ) ) ;
#7624=CARTESIAN_POINT ( 'NONE',  ( -3.750000000000000000, 2.312500000000000888, -5.053300858899105741 ) ) ;
#7631=CARTESIAN_POINT ( 'NONE',  ( -3.249999999999999556, 10.18750000000000000, -2.153805922287440833 ) ) ;
#7633=CARTESIAN_POINT ( 'NONE',  ( -2.298097038856278029, 4.624999999999999112, -1.201902961143720638 ) ) ;
#7634=CARTESIAN_POINT ( 'NONE',  ( -2.298097038856278029, 12.62500000000000000, -1.201902961143720638 ) ) ;
#7638=CARTESIAN_POINT ( 'NONE',  ( 1.346194077712558057, 3.562500000000000444, -6.750000000000000000 ) ) ;
#7639=CARTESIAN_POINT ( 'NONE',  ( -2.651650429449552870, 4.624999999999999112, -0.8483495705504467965 ) ) ;
#7640=CARTESIAN_POINT ( 'NONE',  ( -3.750000000000000000, 9.312500000000000000, -5.053300858899105741 ) ) ;
#7644=CARTESIAN_POINT ( 'NONE',  ( -3.750000000000000000, 11.81250000000000178, -5.053300858899105741 ) ) ;
#7655=CARTESIAN_POINT ( 'NONE',  ( -2.651650429449552870, 12.62500000000000000, -0.8483495705504463524 ) ) ;
#7659=CARTESIAN_POINT ( 'NONE',  ( -2.651650429449552870, 8.625000000000000000, -0.8483495705504467965 ) ) ;
#7662=CARTESIAN_POINT ( 'NONE',  ( -2.298097038856278029, 7.625000000000000000, -1.201902961143720638 ) ) ;
#7664=CARTESIAN_POINT ( 'NONE',  ( -4.592425496802573972E-16, 12.50000000000000000, -7.249999999999999112 ) ) ;
#7669=CARTESIAN_POINT ( 'NONE',  ( 2.298097038856278473, 10.62500000000000000, -5.798097038856279362 ) ) ;
#7676=DIRECTION ( 'NONE',  ( -1.000000000000000000, -0.000000000000000000, -0.000000000000000000 ) ) ;
#7677=ORIENTED_EDGE ( 'NONE', *, *, #12902, .F. ) ;
#7681=CARTESIAN_POINT ( 'NONE',  ( -2.651650429449552870, 14.87500000000000355, -6.151650429449552426 ) ) ;
#7682=CARTESIAN_POINT ( 'NONE',  ( 3.249999999999998224, 12.31250000000000178, -2.153805922287439945 ) ) ;
#7683=CARTESIAN_POINT ( 'NONE',  ( -3.249999999999999556, 12.74999999999999822, -3.500000000000000000 ) ) ;
#7686=CARTESIAN_POINT ( 'NONE',  ( -2.298097038856278918, 10.37500000000000000, -5.798097038856277585 ) ) ;
#7693=VERTEX_POINT ( 'NONE', #14721 ) ;
#7695=CARTESIAN_POINT ( 'NONE',  ( 2.298097038856279362, 4.875000000000000000, -1.201902961143720860 ) ) ;
#7697=CARTESIAN_POINT ( 'NONE',  ( 3.750000000000000000, 12.75000000000000178, -3.500000000000000444 ) ) ;
#7702=CARTESIAN_POINT ( 'NONE',  ( -1.553300858899106629, 3.062500000000000000, 0.2500000000000002220 ) ) ;
#7705=CARTESIAN_POINT ( 'NONE',  ( 3.749999999999999112, 0.6875000000000000000, -5.053300858899108405 ) ) ;
#7712=CARTESIAN_POINT ( 'NONE',  ( -3.249999999999999112, 3.812500000000000000, -4.846194077712558723 ) ) ;
#7714=CARTESIAN_POINT ( 'NONE',  ( -1.346194077712559167, 10.93750000000000000, -6.749999999999999112 ) ) ;
#7719=CARTESIAN_POINT ( 'NONE',  ( -2.298097038856278473, 7.125000000000000000, -1.201902961143720416 ) ) ;
#7720=CARTESIAN_POINT ( 'NONE',  ( 2.651650429449552870, 6.125000000000000000, -6.151650429449553314 ) ) ;
#7721=CARTESIAN_POINT ( 'NONE',  ( -3.750000000000000000, 9.250000000000000000, -3.499999999999999112 ) ) ;
#7725=CARTESIAN_POINT ( 'NONE',  ( 3.750000000000000000, 8.312500000000003553, -1.946699141100892705 ) ) ;
#7731=CARTESIAN_POINT ( 'NONE',  ( 2.298097038856279362, 0.8750000000000000000, -1.201902961143720860 ) ) ;
#7733=CARTESIAN_POINT ( 'NONE',  ( -2.298097038856279362, -0.1249999999999999029, -5.798097038856278473 ) ) ;
#7742=CARTESIAN_POINT ( 'NONE',  ( 3.249999999999998224, 7.312500000000000000, -2.153805922287439945 ) ) ;
#7745=CARTESIAN_POINT ( 'NONE',  ( 1.553300858899105963, 13.56250000000000000, -7.250000000000000888 ) ) ;
#7748=CARTESIAN_POINT ( 'NONE',  ( 2.298097038856278473, 13.62500000000000000, -5.798097038856279362 ) ) ;
#7751=CARTESIAN_POINT ( 'NONE',  ( 3.249999999999999556, 6.750000000000000000, -3.500000000000000000 ) ) ;
#7755=B_SPLINE_CURVE_WITH_KNOTS ( 'NONE', 3,
 ( #13099, #6056, #4830, #4751 ),
 .UNSPECIFIED., .F., .F.,
 ( 4, 4 ),
 ( 0.000000000000000000, 0.0003766621653985018536 ),
 .UNSPECIFIED. ) ;
#7759=CARTESIAN_POINT ( 'NONE',  ( -1.553300858899106629, 0.06250000000000002776, 0.2500000000000002220 ) ) ;
#7760=CARTESIAN_POINT ( 'NONE',  ( -2.298097038856278029, 13.62500000000000000, -1.201902961143720638 ) ) ;
#7761=CARTESIAN_POINT ( 'NONE',  ( 3.249999999999998224, 14.31250000000000355, -2.153805922287439945 ) ) ;
#7763=CARTESIAN_POINT ( 'NONE',  ( -1.346194077712559389, 12.06250000000000000, -0.2500000000000002220 ) ) ;
#7767=CARTESIAN_POINT ( 'NONE',  ( -0.3766621274091715987, 0.5000000000000000000, -0.1347136637304948981 ) ) ;
#7774=CARTESIAN_POINT ( 'NONE',  ( -3.249999999999999556, 4.312500000000000888, -4.846194077712557835 ) ) ;
#7776=CARTESIAN_POINT ( 'NONE',  ( 2.651650429449554203, 3.375000000000000444, -0.8483495705504471296 ) ) ;
#7780=CARTESIAN_POINT ( 'NONE',  ( 1.553300858899105963, 3.562500000000000444, -7.250000000000000888 ) ) ;
#7781=EDGE_CURVE ( 'NONE', #2992, #14660, #12679, .T. ) ;
#7785=CARTESIAN_POINT ( 'NONE',  ( 2.651650429449553759, 0.8750000000000000000, -0.8483495705504471296 ) ) ;
#7789=CARTESIAN_POINT ( 'NONE',  ( -2.298097038856278473, 11.12500000000000000, -1.201902961143720416 ) ) ;
#7793=CARTESIAN_POINT ( 'NONE',  ( -1.346194077712558945, 3.562500000000000888, -0.2500000000000002220 ) ) ;
#7796=CARTESIAN_POINT ( 'NONE',  ( 2.651650429449552870, 7.124999999999999112, -6.151650429449553314 ) ) ;
#7797=CARTESIAN_POINT ( 'NONE',  ( -1.553300858899107073, 8.437500000000000000, -7.250000000000000000 ) ) ;
#7801=CARTESIAN_POINT ( 'NONE',  ( 3.750000000000000000, 9.312500000000000000, -1.946699141100892705 ) ) ;
#7810=CARTESIAN_POINT ( 'NONE',  ( -3.249999999999999112, 3.687500000000000444, -2.153805922287440833 ) ) ;
#7817=CARTESIAN_POINT ( 'NONE',  ( -3.249999999999999556, 9.750000000000000000, -3.500000000000000000 ) ) ;
#7819=CARTESIAN_POINT ( 'NONE',  ( 1.553300858899108849, 12.93750000000000000, 0.2499999999999993616 ) ) ;
#7822=CARTESIAN_POINT ( 'NONE',  ( -2.298097038856278918, 13.37500000000000000, -5.798097038856277585 ) ) ;
#7827=CARTESIAN_POINT ( 'NONE',  ( -1.346194077712559389, 9.437500000000000000, -6.749999999999999112 ) ) ;
#7834=CARTESIAN_POINT ( 'NONE',  ( 1.553300858899105963, 2.562500000000000444, -7.250000000000000888 ) ) ;
#7835=CARTESIAN_POINT ( 'NONE',  ( 0.000000000000000000, 15.50000000000000178, -0.2500000000000002220 ) ) ;
#7836=CARTESIAN_POINT ( 'NONE',  ( -3.980102097228897245E-16, 1.500000000000000000, -6.749999999999999112 ) ) ;
#7838=CARTESIAN_POINT ( 'NONE',  ( 3.249999999999999112, 11.81249999999999822, -2.153805922287439945 ) ) ;
#7841=PLANE ( 'NONE',  #3008 ) ;
#7848=CARTESIAN_POINT ( 'NONE',  ( -3.980102097228897245E-16, 6.500000000000000888, -6.749999999999999112 ) ) ;
#7850=CARTESIAN_POINT ( 'NONE',  ( -1.553300858899106629, 3.562500000000000888, 0.2500000000000002220 ) ) ;
#7853=CARTESIAN_POINT ( 'NONE',  ( -1.553300858899107295, 7.437500000000000888, -7.250000000000000000 ) ) ;
#7856=CARTESIAN_POINT ( 'NONE',  ( -3.750000000000000000, 3.187500000000000444, -1.946699141100892927 ) ) ;
#7860=VERTEX_POINT ( 'NONE', #1636 ) ;
#7861=CARTESIAN_POINT ( 'NONE',  ( -3.249999999999999112, 2.812500000000000444, -4.846194077712558723 ) ) ;
#7864=CARTESIAN_POINT ( 'NONE',  ( 2.651650429449553314, 8.375000000000000000, -0.8483495705504476847 ) ) ;
#7865=CARTESIAN_POINT ( 'NONE',  ( -1.553300858899106407, 13.06250000000000000, 0.2500000000000002220 ) ) ;
#7868=CARTESIAN_POINT ( 'NONE',  ( -2.651650429449552870, 9.624999999999998224, -0.8483495705504463524 ) ) ;
#7876=CARTESIAN_POINT ( 'NONE',  ( 3.249999999999999556, 3.250000000000000000, -3.500000000000000000 ) ) ;
#7885=CARTESIAN_POINT ( 'NONE',  ( 3.249999999999999556, 10.25000000000000178, -3.500000000000000000 ) ) ;
#7888=CARTESIAN_POINT ( 'NONE',  ( 2.651650429449553759, 12.87500000000000178, -0.8483495705504471296 ) ) ;
#7891=CARTESIAN_POINT ( 'NONE',  ( -2.298097038856278473, 12.12500000000000000, -1.201902961143720416 ) ) ;
#7894=PLANE ( 'NONE',  #4319 ) ;
#7895=CARTESIAN_POINT ( 'NONE',  ( 1.346194077712558057, 10.56250000000000000, -6.750000000000000000 ) ) ;
#7901=CARTESIAN_POINT ( 'NONE',  ( -4.592425496802573972E-16, 2.500000000000000000, -7.249999999999999112 ) ) ;
#7902=CARTESIAN_POINT ( 'NONE',  ( 2.651650429449552870, 1.124999999999999778, -6.151650429449553314 ) ) ;
#7904=ORIENTED_EDGE ( 'NONE', *, *, #10640, .T. ) ;
#7906=CARTESIAN_POINT ( 'NONE',  ( -3.249999999999999556, 12.31250000000000000, -4.846194077712557835 ) ) ;
#7907=ADVANCED_FACE ( 'NONE', ( #6275 ), #12373, .F. ) ;
#7909=AXIS2_PLACEMENT_3D ( 'NONE', #9610, #15207, #13022 ) ;
#7922=CARTESIAN_POINT ( 'NONE',  ( -2.298097038856278473, 11.12500000000000000, -1.201902961143720416 ) ) ;
#7926=CARTESIAN_POINT ( 'NONE',  ( 0.000000000000000000, 6.000000000000000000, -0.2500000000000002220 ) ) ;
#7928=CARTESIAN_POINT ( 'NONE',  ( -1.553300858899106629, 1.562500000000000222, 0.2500000000000002220 ) ) ;
#7931=CARTESIAN_POINT ( 'NONE',  ( 2.298097038856278473, 0.6250000000000000000, -5.798097038856279362 ) ) ;
#7932=CARTESIAN_POINT ( 'NONE',  ( 2.651650429449553759, 3.875000000000000000, -0.8483495705504471296 ) ) ;
#7940=CARTESIAN_POINT ( 'NONE',  ( 0.000000000000000000, 1.500000000000000222, -0.2500000000000002220 ) ) ;
#7942=CARTESIAN_POINT ( 'NONE',  ( 3.749999999999998668, 8.187500000000000000, -5.053300858899108405 ) ) ;
#7943=CARTESIAN_POINT ( 'NONE',  ( 2.651650429449552870, 14.62500000000000000, -6.151650429449554203 ) ) ;
#7947=CARTESIAN_POINT ( 'NONE',  ( 0.000000000000000000, 13.50000000000000178, 0.2500000000000002220 ) ) ;
#7954=CARTESIAN_POINT ( 'NONE',  ( -3.249999999999999556, 0.1874999999999999722, -2.153805922287440833 ) ) ;
#7956=CARTESIAN_POINT ( 'NONE',  ( -1.346194077712559167, 1.937500000000000222, -6.749999999999999112 ) ) ;
#7963=CARTESIAN_POINT ( 'NONE',  ( -2.298097038856279362, 13.87500000000000178, -5.798097038856278473 ) ) ;
#7965=CARTESIAN_POINT ( 'NONE',  ( -2.651650429449553314, 3.875000000000000444, -6.151650429449552426 ) ) ;
#7973=CARTESIAN_POINT ( 'NONE',  ( 3.249999999999999112, 8.812500000000000000, -2.153805922287439945 ) ) ;
#7980=CARTESIAN_POINT ( 'NONE',  ( -1.553300858899107295, 2.437500000000000444, -7.250000000000000000 ) ) ;
#7982=CARTESIAN_POINT ( 'NONE',  ( 3.249999999999998224, 14.31250000000000355, -2.153805922287439945 ) ) ;
#7986=CARTESIAN_POINT ( 'NONE',  ( 3.249999999999999112, 14.81250000000000000, -2.153805922287439945 ) ) ;
#7989=CARTESIAN_POINT ( 'NONE',  ( 3.249999999999999556, 3.750000000000000000, -3.500000000000000000 ) ) ;
#7999=CARTESIAN_POINT ( 'NONE',  ( -3.980102097228897245E-16, 12.50000000000000000, -6.749999999999999112 ) ) ;
#8002=CARTESIAN_POINT ( 'NONE',  ( -3.249999999999999556, 3.187500000000000000, -2.153805922287440833 ) ) ;
#8003=CARTESIAN_POINT ( 'NONE',  ( -2.651650429449552870, 1.625000000000000000, -0.8483495705504463524 ) ) ;
#8004=CARTESIAN_POINT ( 'NONE',  ( 1.346194077712558279, 7.062500000000000888, -6.750000000000000888 ) ) ;
#8008=CARTESIAN_POINT ( 'NONE',  ( 1.553300858899108849, 4.937500000000001776, 0.2499999999999993616 ) ) ;
#8016=CARTESIAN_POINT ( 'NONE',  ( 2.298097038856278029, 8.125000000000000000, -5.798097038856279362 ) ) ;
#8019=CARTESIAN_POINT ( 'NONE',  ( 3.749999999999999112, 9.312500000000001776, -1.946699141100893149 ) ) ;
#8024=CARTESIAN_POINT ( 'NONE',  ( -2.298097038856278473, 8.125000000000000000, -1.201902961143720416 ) ) ;
#8025=CARTESIAN_POINT ( 'NONE',  ( 2.651650429449554203, 13.37500000000000000, -0.8483495705504471296 ) ) ;
#8031=CARTESIAN_POINT ( 'NONE',  ( -1.346194077712559167, 0.4375000000000000000, -6.749999999999999112 ) ) ;
#8033=CARTESIAN_POINT ( 'NONE',  ( -2.298097038856278029, 3.625000000000000888, -1.201902961143720638 ) ) ;
#8039=CARTESIAN_POINT ( 'NONE',  ( -2.298097038856279362, 12.87500000000000178, -5.798097038856278473 ) ) ;
#8041=CARTESIAN_POINT ( 'NONE',  ( -2.651650429449553314, 0.8750000000000000000, -6.151650429449552426 ) ) ;
#8046=CARTESIAN_POINT ( 'NONE',  ( -2.298097038856278473, 8.125000000000000000, -1.201902961143720416 ) ) ;
#8052=CARTESIAN_POINT ( 'NONE',  ( -3.749999999999999556, 4.187500000000000000, -1.946699141100892927 ) ) ;
#8053=CARTESIAN_POINT ( 'NONE',  ( -1.553300858899106629, 1.562500000000000222, 0.2499999999999998335 ) ) ;
#8059=CARTESIAN_POINT ( 'NONE',  ( 2.298097038856278029, 1.124999999999999778, -5.798097038856279362 ) ) ;
#8064=CARTESIAN_POINT ( 'NONE',  ( -3.249999999999999556, 4.312500000000000888, -4.846194077712557835 ) ) ;
#8070=CARTESIAN_POINT ( 'NONE',  ( -1.346194077712558945, 9.062500000000000000, -0.2500000000000002220 ) ) ;
#8073=CARTESIAN_POINT ( 'NONE',  ( -3.749999999999999556, 9.750000000000000000, -3.499999999999999112 ) ) ;
#8075=CARTESIAN_POINT ( 'NONE',  ( 2.651650429449554203, 0.3750000000000001110, -0.8483495705504471296 ) ) ;
#8076=CARTESIAN_POINT ( 'NONE',  ( -3.249999999999999112, 7.687500000000000888, -2.153805922287440833 ) ) ;
#8079=CARTESIAN_POINT ( 'NONE',  ( 1.346194077712560944, 4.937500000000001776, -0.2500000000000010547 ) ) ;
#8080=CARTESIAN_POINT ( 'NONE',  ( -3.749999999999999556, 7.312500000000000888, -5.053300858899104853 ) ) ;
#8081=EDGE_CURVE ( 'NONE', #4358, #3762, #11663, .T. ) ;
#8086=CARTESIAN_POINT ( 'NONE',  ( 0.3766621274091715987, 0.5000000000000000000, 0.1491815183709511716 ) ) ;
#8088=CARTESIAN_POINT ( 'NONE',  ( 3.249999999999998224, 7.187500000000000888, -4.846194077712561388 ) ) ;
#8091=CARTESIAN_POINT ( 'NONE',  ( 3.749999999999999556, 8.250000000000000000, -3.500000000000000444 ) ) ;
#8093=CARTESIAN_POINT ( 'NONE',  ( 3.749999999999999556, 14.81250000000000178, -1.946699141100892261 ) ) ;
#8097=CARTESIAN_POINT ( 'NONE',  ( -2.651650429449553314, 12.87500000000000000, -6.151650429449552426 ) ) ;
#8103=CARTESIAN_POINT ( 'NONE',  ( 1.346194077712558279, 2.562500000000000444, -6.750000000000000000 ) ) ;
#8105=CARTESIAN_POINT ( 'NONE',  ( 3.249999999999999556, 1.250000000000000222, -3.500000000000000000 ) ) ;
#8111=CARTESIAN_POINT ( 'NONE',  ( 3.249999999999999556, 12.25000000000000000, -3.500000000000000000 ) ) ;
#8113=CARTESIAN_POINT ( 'NONE',  ( -1.553300858899107073, 1.937500000000000222, -7.249999999999999112 ) ) ;
#8119=CARTESIAN_POINT ( 'NONE',  ( -3.249999999999999556, 14.25000000000000000, -3.499999999999999556 ) ) ;
#8125=CARTESIAN_POINT ( 'NONE',  ( -1.553300858899107295, 3.437500000000000000, -7.250000000000000000 ) ) ;
#8126=CARTESIAN_POINT ( 'NONE',  ( 2.651650429449552870, 4.125000000000000000, -6.151650429449553314 ) ) ;
#8131=CARTESIAN_POINT ( 'NONE',  ( -1.346194077712559389, 13.06250000000000000, -0.2500000000000002220 ) ) ;
#8135=CARTESIAN_POINT ( 'NONE',  ( 3.249999999999999112, 2.812500000000000000, -2.153805922287439945 ) ) ;
#8141=CARTESIAN_POINT ( 'NONE',  ( 3.249999999999999556, 11.75000000000000000, -3.500000000000000000 ) ) ;
#8144=CARTESIAN_POINT ( 'NONE',  ( 3.749999999999999556, 9.249999999999998224, -3.500000000000000444 ) ) ;
#8146=CARTESIAN_POINT ( 'NONE',  ( 3.749999999999999112, 6.187500000000001776, -5.053300858899108405 ) ) ;
#8147=CARTESIAN_POINT ( 'NONE',  ( 2.298097038856279362, 5.375000000000000888, -1.201902961143720860 ) ) ;
#8151=CARTESIAN_POINT ( 'NONE',  ( -1.346194077712559389, 1.437500000000000000, -6.749999999999999112 ) ) ;
#8154=CARTESIAN_POINT ( 'NONE',  ( -2.651650429449552870, 4.125000000000000000, -0.8483495705504462414 ) ) ;
#8164=CARTESIAN_POINT ( 'NONE',  ( -2.298097038856279362, 5.875000000000000888, -5.798097038856278473 ) ) ;
#8167=CARTESIAN_POINT ( 'NONE',  ( 1.553300858899109071, 8.437500000000000000, 0.2499999999999989175 ) ) ;
#8168=CARTESIAN_POINT ( 'NONE',  ( -3.750000000000000000, 14.25000000000000000, -3.499999999999999112 ) ) ;
#8171=CARTESIAN_POINT ( 'NONE',  ( -3.980102097228897738E-16, 1.084202172485504434E-16, -6.749999999999999112 ) ) ;
#8179=FACE_OUTER_BOUND ( 'NONE', #8694, .T. ) ;
#8180=CARTESIAN_POINT ( 'NONE',  ( 0.000000000000000000, 4.000000000000000000, -0.2500000000000002220 ) ) ;
#8184=CARTESIAN_POINT ( 'NONE',  ( 2.298097038856279362, 8.375000000000000000, -1.201902961143720860 ) ) ;
#8188=CARTESIAN_POINT ( 'NONE',  ( 1.346194077712560944, 0.9374999999999998890, -0.2500000000000010547 ) ) ;
#8189=CARTESIAN_POINT ( 'NONE',  ( -2.298097038856279362, 10.87500000000000000, -5.798097038856278473 ) ) ;
#8191=CARTESIAN_POINT ( 'NONE',  ( 2.651650429449554203, 3.375000000000000444, -0.8483495705504471296 ) ) ;
#8196=CARTESIAN_POINT ( 'NONE',  ( -3.980102097228897245E-16, 11.50000000000000000, -6.749999999999999112 ) ) ;
#8203=CARTESIAN_POINT ( 'NONE',  ( -3.749999999999999556, 4.312500000000000888, -5.053300858899104853 ) ) ;
#8204=CARTESIAN_POINT ( 'NONE',  ( 2.651650429449552870, 6.125000000000000000, -6.151650429449553314 ) ) ;
#8209=CARTESIAN_POINT ( 'NONE',  ( -3.980102097228897245E-16, 14.50000000000000000, -6.749999999999999112 ) ) ;
#8213=CARTESIAN_POINT ( 'NONE',  ( -2.298097038856278918, 4.375000000000000000, -5.798097038856277585 ) ) ;
#8217=ORIENTED_EDGE ( 'NONE', *, *, #1681, .T. ) ;
#8220=CARTESIAN_POINT ( 'NONE',  ( -3.249999999999999556, 14.31250000000000000, -4.846194077712557835 ) ) ;
#8225=CARTESIAN_POINT ( 'NONE',  ( -3.749999999999999556, 7.750000000000000888, -3.499999999999999112 ) ) ;
#8226=CARTESIAN_POINT ( 'NONE',  ( 2.298097038856279362, 8.375000000000000000, -1.201902961143720860 ) ) ;
#8229=CARTESIAN_POINT ( 'NONE',  ( 0.000000000000000000, 3.000000000000000000, -0.2500000000000002220 ) ) ;
#8230=CARTESIAN_POINT ( 'NONE',  ( -1.553300858899107295, 9.437500000000000000, -7.250000000000000000 ) ) ;
#8240=CARTESIAN_POINT ( 'NONE',  ( -3.980102097228897738E-16, 8.999999999999998224, -6.749999999999999112 ) ) ;
#8242=CARTESIAN_POINT ( 'NONE',  ( 3.749999999999999112, 12.31250000000000178, -1.946699141100893149 ) ) ;
#8247=CARTESIAN_POINT ( 'NONE',  ( 3.750000000000000000, 13.31250000000000178, -1.946699141100892705 ) ) ;
#8251=CARTESIAN_POINT ( 'NONE',  ( -3.249999999999999556, 14.18750000000000000, -2.153805922287440833 ) ) ;
#8255=CARTESIAN_POINT ( 'NONE',  ( 1.346194077712560944, 1.937500000000000000, -0.2500000000000011102 ) ) ;
#8257=CARTESIAN_POINT ( 'NONE',  ( 3.249999999999999556, 5.250000000000000000, -3.500000000000000000 ) ) ;
#8262=CARTESIAN_POINT ( 'NONE',  ( 0.000000000000000000, 0.000000000000000000, -0.2500000000000002220 ) ) ;
#8263=CARTESIAN_POINT ( 'NONE',  ( -1.346194077712558945, 12.56250000000000355, -0.2500000000000002220 ) ) ;
#8264=CARTESIAN_POINT ( 'NONE',  ( -3.750000000000000000, 7.187500000000000000, -1.946699141100892927 ) ) ;
#8266=CARTESIAN_POINT ( 'NONE',  ( -3.750000000000000000, 3.687500000000000444, -1.946699141100893149 ) ) ;
#8272=CARTESIAN_POINT ( 'NONE',  ( 2.298097038856279362, 10.87500000000000178, -1.201902961143720860 ) ) ;
#8279=CARTESIAN_POINT ( 'NONE',  ( 2.651650429449553759, 5.875000000000000000, -0.8483495705504471296 ) ) ;
#8280=CARTESIAN_POINT ( 'NONE',  ( 1.553300858899109071, 5.437500000000000888, 0.2499999999999989175 ) ) ;
#8283=CARTESIAN_POINT ( 'NONE',  ( 2.298097038856279362, 14.87500000000000178, -1.201902961143720860 ) ) ;
#8289=CARTESIAN_POINT ( 'NONE',  ( 3.249999999999999112, 4.812500000000000888, -2.153805922287439945 ) ) ;
#8299=CARTESIAN_POINT ( 'NONE',  ( -1.553300858899107073, 5.937500000000002665, -7.249999999999999112 ) ) ;
#8300=CARTESIAN_POINT ( 'NONE',  ( -3.249999999999999556, 4.750000000000000888, -3.500000000000000000 ) ) ;
#8303=CARTESIAN_POINT ( 'NONE',  ( -1.346194077712559389, 3.437500000000000000, -6.749999999999999112 ) ) ;
#8310=( BOUNDED_CURVE ( )  B_SPLINE_CURVE ( 2, ( #6468, #10103, #12272, #11184, #4240, #1842, #2853, #3071, #10029, #758, #7553, #7705, #4164, #11335, #7785, #13366, #8866, #5389, #4011, #2922, #12192, #14840, #12498, #1610, #14612, #5468, #6549, #11261, #8713, #8944, #684, #13672, #5163, #1915, #6628, #11037, #1680, #7624, #6393, #11105, #9951, #14689, #4091, #8794, #14920, #836, #4316, #3142, #9020, #5541, #13745, #7856, #12574, #1988, #6705, #11417, #1547, #14304, #2397, #7408, #9507, #14231, #7333, #6260, #10741, #10977, #156, #7093, #10811, #12993, #7257, #5103, #12131, #10665, #4794, #9658, #9745, #11814, #1234, #227, #2631, #3633, #12044, #5026, #4865, #13228, #14389, #11891, #14473, #394, #8495, #1314, #8413, #10896, #9577, #6020, #14158, #3788, #1393, #11973, #8335, #13060, #6096, #3870, #7171, #4943, #8571, #1465, #2475, #13304, #6177, #3559, #3705, #312, #2706, #8264, #5942, #82, #13145, #2555, #9893, #6338, #469, #5401, #3083, #7491, #5181, #11345, #10042, #14779, #14629, #10115, #3015, #8880, #11052, #7797, #14857, #13686, #12210, #13537, #1625, #774, #1857, #4176, #4026, #11202, #8731, #13613, #7721, #7640, #4106, #12507, #8955, #12285, #6638, #12435, #8807, #6562, #13464, #11275, #9818, #1926, #2867, #14550, #696, #8649, #7566, #3945, #4254, #13383, #624, #11127, #2789, #14706, #1695, #2936, #6407, #543, #5256, #9966, #12359, #1776, #6485, #5330, #15232, #14999, #10198, #14932, #4552, #11723, #920, #989, #3151, #12818, #4472, #5776, #4328, #9335, #4624, #4396, #9031, #15075, #11572, #12584, #2224, #3456, #5480, #13756, #11651, #7865, #9260, #10499, #13985, #14057, #13826, #6860, #2002, #10420, #10266, #11505, #5551, #6713, #11426, #6934, #9182, #9104, #12745, #3230, #8168, #12896, #12663, #2306, #848, #3311, #7943, #5700, #13913, #8093, #5621, #2079, #6791 ),
 .UNSPECIFIED., .F., .F. ) 
 B_SPLINE_CURVE_WITH_KNOTS ( ( 3, 2, 2, 2, 2, 2, 2, 2, 2, 2, 2, 2, 2, 2, 2, 2, 2, 2, 2, 2, 2, 2, 2, 2, 2, 2, 2, 2, 2, 2, 2, 2, 2, 2, 2, 2, 2, 2, 2, 2, 2, 2, 2, 2, 2, 2, 2, 2, 2, 2, 2, 2, 2, 2, 2, 2, 2, 2, 2, 2, 2, 2, 2, 2, 2, 2, 2, 2, 2, 2, 2, 2, 2, 2, 2, 2, 2, 2, 2, 2, 2, 2, 2, 2, 2, 2, 2, 2, 2, 2, 2, 2, 2, 2, 2, 2, 2, 2, 2, 2, 2, 2, 2, 2, 2, 2, 2, 2, 2, 2, 2, 2, 2, 2, 2, 2, 2, 2, 2, 2, 3 ),
 ( 0.000000000000000000, 0.008333333333333333218, 0.01666666666666666644, 0.02500000000000000139, 0.03333333333333333287, 0.04166666666666666435, 0.05000000000000000278, 0.05833333333333333426, 0.06666666666666666574, 0.07499999999999999722, 0.08333333333333332871, 0.09166666666666666019, 0.1000000000000000056, 0.1083333333333333370, 0.1166666666666666685, 0.1250000000000000000, 0.1333333333333333315, 0.1416666666666666630, 0.1499999999999999944, 0.1583333333333333259, 0.1666666666666666574, 0.1749999999999999889, 0.1833333333333333204, 0.1916666666666666519, 0.2000000000000000111, 0.2083333333333333426, 0.2166666666666666741, 0.2250000000000000056, 0.2333333333333333370, 0.2416666666666666685, 0.2500000000000000000, 0.2583333333333333037, 0.2666666666666666630, 0.2750000000000000222, 0.2833333333333333259, 0.2916666666666666852, 0.2999999999999999889, 0.3083333333333333481, 0.3166666666666666519, 0.3250000000000000111, 0.3333333333333333148, 0.3416666666666666741, 0.3499999999999999778, 0.3583333333333333370, 0.3666666666666666408, 0.3750000000000000000, 0.3833333333333333037, 0.3916666666666666630, 0.4000000000000000222, 0.4083333333333333259, 0.4166666666666666852, 0.4249999999999999889, 0.4333333333333333481, 0.4416666666666666519, 0.4500000000000000111, 0.4583333333333333148, 0.4666666666666666741, 0.4749999999999999778, 0.4833333333333333370, 0.4916666666666666408, 0.5000000000000000000, 0.5083333333333333037, 0.5166666666666666075, 0.5250000000000000222, 0.5333333333333333259, 0.5416666666666666297, 0.5500000000000000444, 0.5583333333333333481, 0.5666666666666666519, 0.5749999999999999556, 0.5833333333333333703, 0.5916666666666666741, 0.5999999999999999778, 0.6083333333333332815, 0.6166666666666666963, 0.6250000000000000000, 0.6333333333333333037, 0.6416666666666666075, 0.6500000000000000222, 0.6583333333333333259, 0.6666666666666666297, 0.6750000000000000444, 0.6833333333333333481, 0.6916666666666666519, 0.6999999999999999556, 0.7083333333333333703, 0.7166666666666666741, 0.7249999999999999778, 0.7333333333333332815, 0.7416666666666666963, 0.7500000000000000000, 0.7583333333333333037, 0.7666666666666666075, 0.7750000000000000222, 0.7833333333333333259, 0.7916666666666666297, 0.8000000000000000444, 0.8083333333333333481, 0.8166666666666666519, 0.8249999999999999556, 0.8333333333333333703, 0.8416666666666666741, 0.8499999999999999778, 0.8583333333333332815, 0.8666666666666666963, 0.8750000000000000000, 0.8833333333333333037, 0.8916666666666666075, 0.9000000000000000222, 0.9083333333333333259, 0.9166666666666666297, 0.9249999999999999334, 0.9333333333333333481, 0.9416666666666666519, 0.9499999999999999556, 0.9583333333333333703, 0.9666666666666666741, 0.9749999999999999778, 0.9833333333333332815, 0.9916666666666666963, 1.000000000000000000 ),
 .UNSPECIFIED. ) 
 CURVE ( )  GEOMETRIC_REPRESENTATION_ITEM ( )  RATIONAL_B_SPLINE_CURVE ( ( 1.000000000000000000, 0.9238795325112867385, 1.000000000000000000, 0.9238795325112867385, 1.000000000000000000, 0.9238795325112867385, 1.000000000000000000, 0.9238795325112867385, 1.000000000000000000, 0.9238795325112867385, 1.000000000000000000, 0.9238795325112867385, 1.000000000000000000, 0.9238795325112867385, 1.000000000000000000, 0.9238795325112867385, 1.000000000000000000, 0.9238795325112867385, 1.000000000000000000, 0.9238795325112867385, 1.000000000000000000, 0.9238795325112867385, 1.000000000000000000, 0.9238795325112867385, 1.000000000000000000, 0.9238795325112867385, 1.000000000000000000, 0.9238795325112867385, 1.000000000000000000, 0.9238795325112867385, 1.000000000000000000, 0.9238795325112867385, 1.000000000000000000, 0.9238795325112867385, 1.000000000000000000, 0.9238795325112867385, 1.000000000000000000, 0.9238795325112867385, 1.000000000000000000, 0.9238795325112867385, 1.000000000000000000, 0.9238795325112867385, 1.000000000000000000, 0.9238795325112867385, 1.000000000000000000, 0.9238795325112867385, 1.000000000000000000, 0.9238795325112867385, 1.000000000000000000, 0.9238795325112867385, 1.000000000000000000, 0.9238795325112867385, 1.000000000000000000, 0.9238795325112867385, 1.000000000000000000, 0.9238795325112867385, 1.000000000000000000, 0.9238795325112867385, 1.000000000000000000, 0.9238795325112867385, 1.000000000000000000, 0.9238795325112867385, 1.000000000000000000, 0.9238795325112867385, 1.000000000000000000, 0.9238795325112867385, 1.000000000000000000, 0.9238795325112867385, 1.000000000000000000, 0.9238795325112867385, 1.000000000000000000, 0.9238795325112867385, 1.000000000000000000, 0.9238795325112867385, 1.000000000000000000, 0.9238795325112867385, 1.000000000000000000, 0.9238795325112867385, 1.000000000000000000, 0.9238795325112867385, 1.000000000000000000, 0.9238795325112867385, 1.000000000000000000, 0.9238795325112867385, 1.000000000000000000, 0.9238795325112867385, 1.000000000000000000, 0.9238795325112867385, 1.000000000000000000, 0.9238795325112867385, 1.000000000000000000, 0.9238795325112867385, 1.000000000000000000, 0.9238795325112867385, 1.000000000000000000, 0.9238795325112867385, 1.000000000000000000, 0.9238795325112867385, 1.000000000000000000, 0.9238795325112867385, 1.000000000000000000, 0.9238795325112867385, 1.000000000000000000, 0.9238795325112867385, 1.000000000000000000, 0.9238795325112867385, 1.000000000000000000, 0.9238795325112867385, 1.000000000000000000, 0.9238795325112867385, 1.000000000000000000, 0.9238795325112867385, 1.000000000000000000, 0.9238795325112867385, 1.000000000000000000, 0.9238795325112867385, 1.000000000000000000, 0.9238795325112867385, 1.000000000000000000, 0.9238795325112867385, 1.000000000000000000, 0.9238795325112867385, 1.000000000000000000, 0.9238795325112867385, 1.000000000000000000, 0.9238795325112867385, 1.000000000000000000, 0.9238795325112867385, 1.000000000000000000, 0.9238795325112867385, 1.000000000000000000, 0.9238795325112867385, 1.000000000000000000, 0.9238795325112867385, 1.000000000000000000, 0.9238795325112867385, 1.000000000000000000, 0.9238795325112867385, 1.000000000000000000, 0.9238795325112867385, 1.000000000000000000, 0.9238795325112867385, 1.000000000000000000, 0.9238795325112867385, 1.000000000000000000, 0.9238795325112867385, 1.000000000000000000, 0.9238795325112867385, 1.000000000000000000, 0.9238795325112867385, 1.000000000000000000, 0.9238795325112867385, 1.000000000000000000, 0.9238795325112867385, 1.000000000000000000, 0.9238795325112867385, 1.000000000000000000, 0.9238795325112867385, 1.000000000000000000, 0.9238795325112867385, 1.000000000000000000, 0.9238795325112867385, 1.000000000000000000, 0.9238795325112867385, 1.000000000000000000, 0.9238795325112867385, 1.000000000000000000, 0.9238795325112867385, 1.000000000000000000, 0.9238795325112867385, 1.000000000000000000, 0.9238795325112867385, 1.000000000000000000, 0.9238795325112867385, 1.000000000000000000, 0.9238795325112867385, 1.000000000000000000, 0.9238795325112867385, 1.000000000000000000, 0.9238795325112867385, 1.000000000000000000, 0.9238795325112867385, 1.000000000000000000, 0.9238795325112867385, 1.000000000000000000, 0.9238795325112867385, 1.000000000000000000, 0.9238795325112867385, 1.000000000000000000, 0.9238795325112867385, 1.000000000000000000, 0.9238795325112867385, 1.000000000000000000, 0.9238795325112867385, 1.000000000000000000, 0.9238795325112867385, 1.000000000000000000, 0.9238795325112867385, 1.000000000000000000, 0.9238795325112867385, 1.000000000000000000, 0.9238795325112867385, 1.000000000000000000, 0.9238795325112867385, 1.000000000000000000, 0.9238795325112867385, 1.000000000000000000, 0.9238795325112867385, 1.000000000000000000, 0.9238795325112867385, 1.000000000000000000, 0.9238795325112867385, 1.000000000000000000, 0.9238795325112867385, 1.000000000000000000, 0.9238795325112867385, 1.000000000000000000, 0.9238795325112867385, 1.000000000000000000, 0.9238795325112867385, 1.000000000000000000, 0.9238795325112867385, 1.000000000000000000, 0.9238795325112867385, 1.000000000000000000, 0.9238795325112867385, 1.000000000000000000, 0.9238795325112867385, 1.000000000000000000, 0.9238795325112867385, 1.000000000000000000, 0.9238795325112867385, 1.000000000000000000, 0.9238795325112867385, 1.000000000000000000, 0.9238795325112867385, 1.000000000000000000, 0.9238795325112867385, 1.000000000000000000, 0.9238795325112867385, 1.000000000000000000 ) ) 
 REPRESENTATION_ITEM ( '' )  );
#8314=CARTESIAN_POINT ( 'NONE',  ( 3.749999999999999112, 14.31250000000000355, -1.946699141100893149 ) ) ;
#8318=CARTESIAN_POINT ( 'NONE',  ( -3.249999999999999556, 1.750000000000000222, -3.500000000000000000 ) ) ;
#8325=CARTESIAN_POINT ( 'NONE',  ( 1.346194077712558279, 3.562500000000000000, -6.750000000000000000 ) ) ;
#8327=CARTESIAN_POINT ( 'NONE',  ( -3.980102097228897738E-16, 7.000000000000000000, -6.749999999999999112 ) ) ;
#8331=CARTESIAN_POINT ( 'NONE',  ( 0.000000000000000000, 15.00000000000000000, 0.000000000000000000 ) ) ;
#8334=CARTESIAN_POINT ( 'NONE',  ( 2.651650429449553314, 2.375000000000000000, -0.8483495705504476847 ) ) ;
#8335=CARTESIAN_POINT ( 'NONE',  ( -3.750000000000000000, 6.250000000000000000, -3.499999999999999112 ) ) ;
#8337=CARTESIAN_POINT ( 'NONE',  ( -4.592425496802573972E-16, 5.000000000000000000, -7.250000000000000000 ) ) ;
#8342=CARTESIAN_POINT ( 'NONE',  ( -3.249999999999999556, 12.25000000000000000, -3.499999999999999556 ) ) ;
#8350=CARTESIAN_POINT ( 'NONE',  ( -3.749999999999999556, 3.312500000000000000, -5.053300858899104853 ) ) ;
#8351=CARTESIAN_POINT ( 'NONE',  ( 0.000000000000000000, 2.500000000000000000, 0.2499999999999998057 ) ) ;
#8354=CARTESIAN_POINT ( 'NONE',  ( 3.249999999999998224, 3.312500000000000000, -2.153805922287439945 ) ) ;
#8358=CARTESIAN_POINT ( 'NONE',  ( 1.346194077712560944, 7.937500000000000888, -0.2500000000000010547 ) ) ;
#8365=CARTESIAN_POINT ( 'NONE',  ( 2.298097038856279362, 14.87500000000000178, -1.201902961143720860 ) ) ;
#8370=CARTESIAN_POINT ( 'NONE',  ( -3.750000000000000000, 5.687500000000000888, -1.946699141100893149 ) ) ;
#8372=CARTESIAN_POINT ( 'NONE',  ( -3.249999999999999112, 11.68749999999999822, -2.153805922287440833 ) ) ;
#8376=CARTESIAN_POINT ( 'NONE',  ( 0.000000000000000000, 7.000000000000000000, -0.2500000000000002220 ) ) ;
#8390=CARTESIAN_POINT ( 'NONE',  ( 0.000000000000000000, 12.50000000000000178, 0.2499999999999998057 ) ) ;
#8393=CARTESIAN_POINT ( 'NONE',  ( -3.249999999999999112, 1.812499999999999778, -4.846194077712558723 ) ) ;
#8397=AXIS2_PLACEMENT_3D ( 'NONE', #8086, #15226, #5545 ) ;
#8399=CARTESIAN_POINT ( 'NONE',  ( -0.3766621274091715987, -0.2500000000000000000, -7.146945437571387671 ) ) ;
#8402=CARTESIAN_POINT ( 'NONE',  ( -3.249999999999999556, 1.312500000000000222, -4.846194077712557835 ) ) ;
#8404=CARTESIAN_POINT ( 'NONE',  ( -1.346194077712558945, 0.5625000000000001110, -0.2500000000000002220 ) ) ;
#8406=CARTESIAN_POINT ( 'NONE',  ( -3.249999999999999112, 4.812500000000001776, -4.846194077712558723 ) ) ;
#8412=CARTESIAN_POINT ( 'NONE',  ( -3.749999999999999556, 1.750000000000000000, -3.499999999999999112 ) ) ;
#8413=CARTESIAN_POINT ( 'NONE',  ( 3.750000000000000000, 5.750000000000000000, -3.500000000000000444 ) ) ;
#8415=CARTESIAN_POINT ( 'NONE',  ( -4.592425496802573972E-16, 6.000000000000000888, -7.250000000000000000 ) ) ;
#8421=CARTESIAN_POINT ( 'NONE',  ( -1.346194077712559389, 11.43750000000000000, -6.749999999999999112 ) ) ;
#8425=PRODUCT ( 'SmallSpring', 'SmallSpring', '', ( #14690 ) ) ;
#8426=CARTESIAN_POINT ( 'NONE',  ( 1.553300858899105963, 10.06250000000000000, -7.250000000000000888 ) ) ;
#8430=CARTESIAN_POINT ( 'NONE',  ( -4.592425496802573972E-16, 9.500000000000000000, -7.249999999999999112 ) ) ;
#8431=CARTESIAN_POINT ( 'NONE',  ( -1.553300858899106629, 4.562500000000000000, 0.2499999999999998335 ) ) ;
#8432=CARTESIAN_POINT ( 'NONE',  ( 0.3766621274091715987, -0.2500000000000000000, 0.1491815183709511716 ) ) ;
#8435=CARTESIAN_POINT ( 'NONE',  ( 2.298097038856278029, 3.125000000000000444, -5.798097038856279362 ) ) ;
#8441=CARTESIAN_POINT ( 'NONE',  ( -3.249999999999999556, 6.250000000000000000, -3.499999999999999556 ) ) ;
#8446=ORIENTED_EDGE ( 'NONE', *, *, #367, .T. ) ;
#8448=CARTESIAN_POINT ( 'NONE',  ( 2.298097038856278473, 14.62500000000000000, -5.798097038856279362 ) ) ;
#8452=CARTESIAN_POINT ( 'NONE',  ( -1.553300858899106629, 5.562500000000001776, 0.2500000000000002220 ) ) ;
#8454=PRODUCT_DEFINITION ( 'UNKNOWN', '', #5003, #7575 ) ;
#8455=CARTESIAN_POINT ( 'NONE',  ( -1.346194077712559167, 8.937500000000000000, -6.749999999999999112 ) ) ;
#8458=CARTESIAN_POINT ( 'NONE',  ( 1.346194077712560944, 5.937500000000000000, -0.2500000000000010547 ) ) ;
#8468=CARTESIAN_POINT ( 'NONE',  ( -1.346194077712559389, 1.437500000000000000, -6.749999999999999112 ) ) ;
#8472=CARTESIAN_POINT ( 'NONE',  ( -3.750000000000000000, 14.81250000000000355, -5.053300858899105741 ) ) ;
#8475=CARTESIAN_POINT ( 'NONE',  ( -1.346194077712559167, 2.937500000000000444, -6.749999999999999112 ) ) ;
#8486=CARTESIAN_POINT ( 'NONE',  ( -1.346194077712558945, 7.062500000000000000, -0.2500000000000002220 ) ) ;
#8488=CARTESIAN_POINT ( 'NONE',  ( 2.298097038856278473, 12.62500000000000000, -5.798097038856279362 ) ) ;
#8489=CARTESIAN_POINT ( 'NONE',  ( 1.346194077712558279, 8.062500000000001776, -6.750000000000000888 ) ) ;
#8492=CARTESIAN_POINT ( 'NONE',  ( -3.249999999999999556, 0.1875000000000000278, -2.153805922287440833 ) ) ;
#8494=CARTESIAN_POINT ( 'NONE',  ( 3.749999999999999556, 1.249999999999999778, -3.500000000000000444 ) ) ;
#8495=CARTESIAN_POINT ( 'NONE',  ( 2.651650429449552870, 5.625000000000000000, -6.151650429449554203 ) ) ;
#8497=CARTESIAN_POINT ( 'NONE',  ( 0.000000000000000000, 4.499999999999999112, 0.2500000000000002220 ) ) ;
#8506=CARTESIAN_POINT ( 'NONE',  ( -1.553300858899106629, 9.562500000000000000, 0.2500000000000002220 ) ) ;
#8510=CARTESIAN_POINT ( 'NONE',  ( -3.750000000000000000, 7.250000000000000000, -3.499999999999999112 ) ) ;
#8511=CARTESIAN_POINT ( 'NONE',  ( -1.553300858899106629, 8.562500000000001776, 0.2499999999999998335 ) ) ;
#8515=CARTESIAN_POINT ( 'NONE',  ( -1.346194077712558945, 5.562500000000000000, -0.2500000000000002220 ) ) ;
#8517=CARTESIAN_POINT ( 'NONE',  ( -3.749999999999999556, 9.312499999999998224, -5.053300858899104853 ) ) ;
#8521=CARTESIAN_POINT ( 'NONE',  ( -2.298097038856278473, 8.125000000000000000, -1.201902961143720416 ) ) ;
#8526=CARTESIAN_POINT ( 'NONE',  ( 3.249999999999999556, 14.75000000000000178, -3.500000000000000000 ) ) ;
#8530=CARTESIAN_POINT ( 'NONE',  ( -3.750000000000000000, 12.68750000000000178, -1.946699141100893149 ) ) ;
#8531=CARTESIAN_POINT ( 'NONE',  ( 1.346194077712561166, 8.437500000000000000, -0.2500000000000011102 ) ) ;
#8532=CARTESIAN_POINT ( 'NONE',  ( 2.298097038856278029, 10.12500000000000000, -5.798097038856279362 ) ) ;
#8536=CARTESIAN_POINT ( 'NONE',  ( -3.980102097228897245E-16, 6.500000000000000888, -6.749999999999999112 ) ) ;
#8543=CARTESIAN_POINT ( 'NONE',  ( -1.346194077712559389, 0.06250000000000000000, -0.2500000000000002220 ) ) ;
#8544=CARTESIAN_POINT ( 'NONE',  ( 3.749999999999998668, 12.68750000000000178, -5.053300858899107517 ) ) ;
#8547=CARTESIAN_POINT ( 'NONE',  ( -2.651650429449552870, 12.62500000000000000, -0.8483495705504467965 ) ) ;
#8550=CARTESIAN_POINT ( 'NONE',  ( 2.298097038856279362, 1.375000000000000000, -1.201902961143720860 ) ) ;
#8558=CARTESIAN_POINT ( 'NONE',  ( 3.249999999999999556, 5.750000000000000000, -3.500000000000000000 ) ) ;
#8560=CARTESIAN_POINT ( 'NONE',  ( -3.249999999999999556, 14.25000000000000000, -3.499999999999999556 ) ) ;
#8562=CARTESIAN_POINT ( 'NONE',  ( -3.980102097228897738E-16, 8.999999999999998224, -6.749999999999999112 ) ) ;
#8569=CARTESIAN_POINT ( 'NONE',  ( -3.980102097228897245E-16, 4.500000000000000888, -6.749999999999999112 ) ) ;
#8570=CARTESIAN_POINT ( 'NONE',  ( 3.249999999999999556, 15.25000000000000355, -3.500000000000000000 ) ) ;
#8571=CARTESIAN_POINT ( 'NONE',  ( 2.651650429449552870, 6.625000000000000000, -6.151650429449554203 ) ) ;
#8573=CARTESIAN_POINT ( 'NONE',  ( 3.750000000000000000, 7.312500000000001776, -1.946699141100892705 ) ) ;
#8578=CARTESIAN_POINT ( 'NONE',  ( 3.249999999999999112, 14.81250000000000000, -2.153805922287439945 ) ) ;
#8582=CARTESIAN_POINT ( 'NONE',  ( 3.750000000000000000, 13.31250000000000178, -1.946699141100892705 ) ) ;
#8586=CARTESIAN_POINT ( 'NONE',  ( -1.553300858899106629, 10.06250000000000000, 0.2500000000000002220 ) ) ;
#8587=CARTESIAN_POINT ( 'NONE',  ( -1.553300858899107073, 6.937500000000001776, -7.249999999999999112 ) ) ;
#8591=CARTESIAN_POINT ( 'NONE',  ( 2.298097038856278029, 4.125000000000000000, -5.798097038856279362 ) ) ;
#8592=CARTESIAN_POINT ( 'NONE',  ( -3.750000000000000000, 11.25000000000000000, -3.499999999999999112 ) ) ;
#8596=CARTESIAN_POINT ( 'NONE',  ( -3.249999999999999556, 9.312499999999998224, -4.846194077712557835 ) ) ;
#8605=CARTESIAN_POINT ( 'NONE',  ( -0.2515148708112424081, 0.2743742620810324939, -6.863050255469944183 ) ) ;
#8606=CARTESIAN_POINT ( 'NONE',  ( 1.553300858899105963, 13.06250000000000178, -7.249999999999999112 ) ) ;
#8607=CARTESIAN_POINT ( 'NONE',  ( 3.249999999999998224, 11.18750000000000178, -4.846194077712561388 ) ) ;
#8609=CARTESIAN_POINT ( 'NONE',  ( -3.249999999999999112, 9.812500000000000000, -4.846194077712558723 ) ) ;
#8612=CARTESIAN_POINT ( 'NONE',  ( 2.298097038856278473, 7.625000000000000000, -5.798097038856279362 ) ) ;
#8619=CARTESIAN_POINT ( 'NONE',  ( 2.298097038856279362, 14.37500000000000000, -1.201902961143720860 ) ) ;
#8620=CARTESIAN_POINT ( 'NONE',  ( 0.000000000000000000, 15.00000000000000000, 0.2500000000000002220 ) ) ;
#8624=CARTESIAN_POINT ( 'NONE',  ( -4.592425496802573972E-16, 2.500000000000000000, -7.249999999999999112 ) ) ;
#8637=CARTESIAN_POINT ( 'NONE',  ( 2.298097038856278473, 5.625000000000000000, -5.798097038856279362 ) ) ;
#8639=CARTESIAN_POINT ( 'NONE',  ( 3.249999999999999112, 13.81250000000000000, -2.153805922287439945 ) ) ;
#8640=CARTESIAN_POINT ( 'NONE',  ( -2.298097038856278029, 10.62500000000000000, -1.201902961143720638 ) ) ;
#8642=CARTESIAN_POINT ( 'NONE',  ( 3.249999999999999112, 0.8125000000000001110, -2.153805922287439945 ) ) ;
#8645=CARTESIAN_POINT ( 'NONE',  ( -3.249999999999999556, 6.250000000000000000, -3.499999999999999556 ) ) ;
#8646=CARTESIAN_POINT ( 'NONE',  ( -2.651650429449552870, 6.875000000000000000, -6.151650429449552426 ) ) ;
#8649=CARTESIAN_POINT ( 'NONE',  ( -3.750000000000000000, 10.31250000000000000, -5.053300858899105741 ) ) ;
#8652=CARTESIAN_POINT ( 'NONE',  ( 1.553300858899109516, 5.437500000000000888, 0.2499999999999993616 ) ) ;
#8665=CARTESIAN_POINT ( 'NONE',  ( 2.651650429449554203, 14.37500000000000000, -0.8483495705504471296 ) ) ;
#8669=CARTESIAN_POINT ( 'NONE',  ( -2.651650429449552870, 8.125000000000000000, -0.8483495705504462414 ) ) ;
#8670=CARTESIAN_POINT ( 'NONE',  ( 1.553300858899105963, 7.062499999999999112, -7.249999999999999112 ) ) ;
#8673=CARTESIAN_POINT ( 'NONE',  ( -3.249999999999999112, 3.687500000000000444, -2.153805922287440833 ) ) ;
#8675=CARTESIAN_POINT ( 'NONE',  ( 3.749999999999999112, 11.81249999999999822, -1.946699141100892039 ) ) ;
#8679=CARTESIAN_POINT ( 'NONE',  ( 3.249999999999999112, 9.812500000000000000, -2.153805922287439945 ) ) ;
#8691=CARTESIAN_POINT ( 'NONE',  ( 3.749999999999998668, 11.18750000000000178, -5.053300858899108405 ) ) ;
#8692=CARTESIAN_POINT ( 'NONE',  ( -2.298097038856279362, 12.87500000000000178, -5.798097038856278473 ) ) ;
#8693=CARTESIAN_POINT ( 'NONE',  ( 2.298097038856279362, 11.37500000000000000, -1.201902961143720860 ) ) ;
#8694=EDGE_LOOP ( 'NONE', ( #13829, #6604, #7677, #4885 ) ) ;
#8696=CARTESIAN_POINT ( 'NONE',  ( -2.298097038856278918, 8.375000000000000000, -5.798097038856277585 ) ) ;
#8705=CARTESIAN_POINT ( 'NONE',  ( -3.249999999999999556, 0.2500000000000000000, -3.499999999999999556 ) ) ;
#8706=CARTESIAN_POINT ( 'NONE',  ( -2.651650429449552870, -0.3749999999999998890, -0.8483495705504463524 ) ) ;
#8709=CARTESIAN_POINT ( 'NONE',  ( 1.553300858899109071, 15.43750000000000178, 0.2499999999999989175 ) ) ;
#8713=CARTESIAN_POINT ( 'NONE',  ( 3.750000000000000000, 1.750000000000000000, -3.500000000000000444 ) ) ;
#8718=CARTESIAN_POINT ( 'NONE',  ( 1.346194077712558279, 8.562500000000000000, -6.750000000000000000 ) ) ;
#8722=CARTESIAN_POINT ( 'NONE',  ( 1.346194077712560944, 13.93750000000000000, -0.2500000000000010547 ) ) ;
#8723=CARTESIAN_POINT ( 'NONE',  ( 3.249999999999998224, 12.31250000000000178, -2.153805922287439945 ) ) ;
#8729=CARTESIAN_POINT ( 'NONE',  ( -1.346194077712559389, 6.437500000000000888, -6.749999999999999112 ) ) ;
#8730=CARTESIAN_POINT ( 'NONE',  ( 3.749999999999999112, 6.312500000000000000, -1.946699141100893149 ) ) ;
#8731=CARTESIAN_POINT ( 'NONE',  ( -2.651650429449552870, 9.125000000000000000, -0.8483495705504462414 ) ) ;
#8734=CARTESIAN_POINT ( 'NONE',  ( 3.749999999999999556, 11.25000000000000000, -3.500000000000000444 ) ) ;
#8743=CARTESIAN_POINT ( 'NONE',  ( -3.249999999999999112, 0.6875000000000000000, -2.153805922287440833 ) ) ;
#8747=CARTESIAN_POINT ( 'NONE',  ( -3.749999999999999556, 9.187500000000000000, -1.946699141100892927 ) ) ;
#8749=CARTESIAN_POINT ( 'NONE',  ( -1.553300858899106629, 6.562500000000000888, 0.2499999999999998335 ) ) ;
#8754=CARTESIAN_POINT ( 'NONE',  ( -3.980102097228897738E-16, 7.000000000000000000, -6.749999999999999112 ) ) ;
#8756=CARTESIAN_POINT ( 'NONE',  ( 0.000000000000000000, 10.00000000000000000, 0.2500000000000002220 ) ) ;
#8760=CARTESIAN_POINT ( 'NONE',  ( 1.346194077712560944, 12.93750000000000000, -0.2500000000000010547 ) ) ;
#8770=CARTESIAN_POINT ( 'NONE',  ( -4.592425496802573972E-16, 13.00000000000000000, -7.250000000000000000 ) ) ;
#8771=CARTESIAN_POINT ( 'NONE',  ( -3.249999999999999112, 10.81250000000000000, -4.846194077712558723 ) ) ;
#8772=CARTESIAN_POINT ( 'NONE',  ( 3.249999999999999556, 0.7500000000000000000, -3.500000000000000000 ) ) ;
#8773=ORIENTED_EDGE ( 'NONE', *, *, #10561, .F. ) ;
#8775=CARTESIAN_POINT ( 'NONE',  ( -2.298097038856278473, 12.12500000000000000, -1.201902961143720416 ) ) ;
#8786=CARTESIAN_POINT ( 'NONE',  ( 1.346194077712560944, 0.9374999999999998890, -0.2500000000000010547 ) ) ;
#8787=CARTESIAN_POINT ( 'NONE',  ( 0.000000000000000000, 13.00000000000000178, 0.2500000000000002220 ) ) ;
#8790=CARTESIAN_POINT ( 'NONE',  ( -2.651650429449553314, 2.375000000000000000, -6.151650429449552426 ) ) ;
#8794=CARTESIAN_POINT ( 'NONE',  ( 3.749999999999999112, 2.687500000000000444, -5.053300858899108405 ) ) ;
#8799=CARTESIAN_POINT ( 'NONE',  ( 2.298097038856279362, 9.875000000000000000, -1.201902961143720860 ) ) ;
#8801=CARTESIAN_POINT ( 'NONE',  ( 3.249999999999999556, 4.249999999999999112, -3.500000000000000000 ) ) ;
#8802=CARTESIAN_POINT ( 'NONE',  ( -1.346194077712559167, 11.93750000000000178, -6.749999999999999112 ) ) ;
#8805=CARTESIAN_POINT ( 'NONE',  ( 3.249999999999998668, 5.687500000000000000, -4.846194077712560500 ) ) ;
#8806=CARTESIAN_POINT ( 'NONE',  ( 0.000000000000000000, 5.500000000000000000, 0.2499999999999998057 ) ) ;
#8807=CARTESIAN_POINT ( 'NONE',  ( 3.750000000000000000, 9.750000000000000000, -3.500000000000000444 ) ) ;
#8810=CARTESIAN_POINT ( 'NONE',  ( -1.553300858899106629, 9.562500000000000000, 0.2500000000000002220 ) ) ;
#8813=EDGE_CURVE ( 'NONE', #11175, #9756, #6318, .T. ) ;
#8820=CARTESIAN_POINT ( 'NONE',  ( 0.000000000000000000, 13.50000000000000178, 0.2500000000000002220 ) ) ;
#8822=DIRECTION ( 'NONE',  ( -1.000000000000000000, 0.000000000000000000, 0.000000000000000000 ) ) ;
#8824=CARTESIAN_POINT ( 'NONE',  ( -3.750000000000000000, 7.687500000000000000, -1.946699141100893149 ) ) ;
#8826=CARTESIAN_POINT ( 'NONE',  ( 3.249999999999999556, 8.250000000000000000, -3.500000000000000000 ) ) ;
#8827=CARTESIAN_POINT ( 'NONE',  ( 3.749999999999999112, 0.1875000000000000833, -5.053300858899108405 ) ) ;
#8831=CARTESIAN_POINT ( 'NONE',  ( 3.249999999999999112, 13.81250000000000000, -2.153805922287439945 ) ) ;
#8834=CARTESIAN_POINT ( 'NONE',  ( -0.3766621274091715987, 0.5000000000000000000, -7.146945437571387671 ) ) ;
#8837=DIRECTION ( 'NONE',  ( 0.000000000000000000, 0.000000000000000000, -1.000000000000000000 ) ) ;
#8838=ORIENTED_EDGE ( 'NONE', *, *, #14209, .T. ) ;
#8841=CARTESIAN_POINT ( 'NONE',  ( 1.553300858899105963, 0.5625000000000001110, -7.250000000000000888 ) ) ;
#8842=CARTESIAN_POINT ( 'NONE',  ( 3.249999999999998224, 9.312500000000001776, -2.153805922287439945 ) ) ;
#8843=CARTESIAN_POINT ( 'NONE',  ( -1.346194077712559389, 0.06250000000000000000, -0.2500000000000002220 ) ) ;
#8845=CARTESIAN_POINT ( 'NONE',  ( -2.298097038856278918, 12.37500000000000000, -5.798097038856277585 ) ) ;
#8849=FACE_OUTER_BOUND ( 'NONE', #2138, .T. ) ;
#8857=CARTESIAN_POINT ( 'NONE',  ( 2.298097038856279362, 3.875000000000000000, -1.201902961143720860 ) ) ;
#8859=CARTESIAN_POINT ( 'NONE',  ( -4.592425496802573972E-16, 14.50000000000000000, -7.249999999999999112 ) ) ;
#8863=CARTESIAN_POINT ( 'NONE',  ( 0.000000000000000000, 2.000000000000000000, 0.2500000000000002220 ) ) ;
#8866=CARTESIAN_POINT ( 'NONE',  ( 0.000000000000000000, 1.000000000000000000, 0.2500000000000002220 ) ) ;
#8873=CARTESIAN_POINT ( 'NONE',  ( -0.3766621274091715987, 0.2398196381212478467, -0.1347136637304948426 ) ) ;
#8874=CARTESIAN_POINT ( 'NONE',  ( -3.249999999999999112, 2.687500000000000888, -2.153805922287440833 ) ) ;
#8875=CARTESIAN_POINT ( 'NONE',  ( -2.298097038856279362, 11.87500000000000000, -5.798097038856278473 ) ) ;
#8878=CARTESIAN_POINT ( 'NONE',  ( 2.298097038856279362, 2.875000000000000000, -1.201902961143720860 ) ) ;
#8879=CARTESIAN_POINT ( 'NONE',  ( 3.749999999999999556, 6.250000000000000000, -3.500000000000000444 ) ) ;
#8880=CARTESIAN_POINT ( 'NONE',  ( -3.750000000000000000, 8.312500000000000000, -5.053300858899105741 ) ) ;
#8885=CARTESIAN_POINT ( 'NONE',  ( -2.651650429449552870, 11.62500000000000000, -0.8483495705504463524 ) ) ;
#8894=CARTESIAN_POINT ( 'NONE',  ( -1.346194077712558945, -0.4374999999999998890, -0.2500000000000002220 ) ) ;
#8898=CARTESIAN_POINT ( 'NONE',  ( -1.553300858899106629, 10.56250000000000355, 0.2499999999999998335 ) ) ;
#8901=CARTESIAN_POINT ( 'NONE',  ( -3.249999999999999556, 6.750000000000000888, -3.500000000000000000 ) ) ;
#8903=CARTESIAN_POINT ( 'NONE',  ( 2.651650429449553759, 11.87500000000000000, -0.8483495705504471296 ) ) ;
#8907=CARTESIAN_POINT ( 'NONE',  ( -2.298097038856278473, 13.12500000000000000, -1.201902961143720416 ) ) ;
#8911=CARTESIAN_POINT ( 'NONE',  ( 3.249999999999999112, 6.812500000000000000, -2.153805922287439945 ) ) ;
#8917=CARTESIAN_POINT ( 'NONE',  ( 2.651650429449553759, 0.8750000000000000000, -0.8483495705504471296 ) ) ;
#8918=CARTESIAN_POINT ( 'NONE',  ( 3.249999999999999556, 10.25000000000000178, -3.500000000000000000 ) ) ;
#8919=CARTESIAN_POINT ( 'NONE',  ( -2.298097038856278473, 0.1250000000000000000, -1.201902961143720416 ) ) ;
#8922=CARTESIAN_POINT ( 'NONE',  ( -3.249999999999999556, 11.31249999999999822, -4.846194077712557835 ) ) ;
#8934=CARTESIAN_POINT ( 'NONE',  ( -2.298097038856278473, 3.125000000000000000, -1.201902961143720416 ) ) ;
#8936=CARTESIAN_POINT ( 'NONE',  ( -3.749999999999999556, 2.750000000000000444, -3.499999999999999112 ) ) ;
#8940=CARTESIAN_POINT ( 'NONE',  ( 1.553300858899105963, 0.5625000000000001110, -7.250000000000000888 ) ) ;
#8944=CARTESIAN_POINT ( 'NONE',  ( 3.749999999999999556, 1.812500000000000000, -1.946699141100892261 ) ) ;
#8950=CARTESIAN_POINT ( 'NONE',  ( 1.346194077712558279, 2.062500000000000000, -6.750000000000000888 ) ) ;
#8953=CARTESIAN_POINT ( 'NONE',  ( -3.749999999999999556, 4.750000000000000000, -3.499999999999999112 ) ) ;
#8955=CARTESIAN_POINT ( 'NONE',  ( -4.592425496802573972E-16, 9.500000000000000000, -7.249999999999999112 ) ) ;
#8958=CARTESIAN_POINT ( 'NONE',  ( -1.346194077712559389, 8.062500000000000000, -0.2500000000000002220 ) ) ;
#8959=CARTESIAN_POINT ( 'NONE',  ( 1.553300858899105963, 9.062500000000000000, -7.250000000000000888 ) ) ;
#8968=CARTESIAN_POINT ( 'NONE',  ( 3.249999999999998224, 2.312500000000000000, -2.153805922287439945 ) ) ;
#8977=CARTESIAN_POINT ( 'NONE',  ( 2.298097038856278029, 9.125000000000001776, -5.798097038856279362 ) ) ;
#8980=CARTESIAN_POINT ( 'NONE',  ( 3.749999999999998668, 14.68750000000000000, -5.053300858899107517 ) ) ;
#8983=CARTESIAN_POINT ( 'NONE',  ( -3.249999999999999556, 11.25000000000000000, -3.499999999999999556 ) ) ;
#8986=CARTESIAN_POINT ( 'NONE',  ( -2.298097038856278473, 10.12500000000000000, -1.201902961143720416 ) ) ;
#8993=CARTESIAN_POINT ( 'NONE',  ( -1.553300858899107295, 1.437500000000000000, -7.250000000000000000 ) ) ;
#8994=CARTESIAN_POINT ( 'NONE',  ( -1.346194077712558945, 14.56250000000000000, -0.2500000000000002220 ) ) ;
#8995=CARTESIAN_POINT ( 'NONE',  ( 3.249999999999999556, 13.25000000000000000, -3.500000000000000000 ) ) ;
#8997=CARTESIAN_POINT ( 'NONE',  ( 3.249999999999999112, 10.81250000000000178, -2.153805922287439945 ) ) ;
#9010=CARTESIAN_POINT ( 'NONE',  ( -3.249999999999999556, 6.187500000000000888, -2.153805922287440833 ) ) ;
#9012=CARTESIAN_POINT ( 'NONE',  ( 2.651650429449552870, 0.1250000000000001110, -6.151650429449555091 ) ) ;
#9017=CARTESIAN_POINT ( 'NONE',  ( -2.651650429449553314, 7.375000000000000888, -6.151650429449552426 ) ) ;
#9020=CARTESIAN_POINT ( 'NONE',  ( 0.000000000000000000, 3.000000000000000000, 0.2500000000000002220 ) ) ;
#9023=PLANE ( 'NONE',  #8397 ) ;
#9026=CARTESIAN_POINT ( 'NONE',  ( -0.1258718175769854841, 0.2162433659573944622, -0.1347136637304948981 ) ) ;
#9027=CARTESIAN_POINT ( 'NONE',  ( -1.346194077712559167, 4.937500000000000000, -6.749999999999999112 ) ) ;
#9030=CARTESIAN_POINT ( 'NONE',  ( 3.749999999999999112, 8.312500000000003553, -1.946699141100893149 ) ) ;
#9031=CARTESIAN_POINT ( 'NONE',  ( -4.592425496802573972E-16, 12.50000000000000000, -7.249999999999999112 ) ) ;
#9035=CARTESIAN_POINT ( 'NONE',  ( 0.000000000000000000, 8.000000000000000000, -0.2500000000000002220 ) ) ;
#9036=CARTESIAN_POINT ( 'NONE',  ( -1.553300858899107073, 8.937500000000000000, -7.249999999999999112 ) ) ;
#9048=CARTESIAN_POINT ( 'NONE',  ( -3.980102097228897738E-16, 4.000000000000000888, -6.749999999999999112 ) ) ;
#9055=CARTESIAN_POINT ( 'NONE',  ( 2.298097038856278029, 10.12500000000000000, -5.798097038856279362 ) ) ;
#9057=CARTESIAN_POINT ( 'NONE',  ( 2.651650429449552870, 13.62500000000000000, -6.151650429449554203 ) ) ;
#9060=CARTESIAN_POINT ( 'NONE',  ( 1.346194077712560944, 13.93750000000000000, -0.2500000000000010547 ) ) ;
#9063=CARTESIAN_POINT ( 'NONE',  ( 2.298097038856279362, 7.875000000000000000, -1.201902961143720860 ) ) ;
#9070=CARTESIAN_POINT ( 'NONE',  ( 2.651650429449552870, 0.6250000000000000000, -6.151650429449554203 ) ) ;
#9071=CARTESIAN_POINT ( 'NONE',  ( 2.298097038856279362, 13.37500000000000000, -1.201902961143720860 ) ) ;
#9072=CARTESIAN_POINT ( 'NONE',  ( 1.346194077712558057, 0.5625000000000001110, -6.750000000000000000 ) ) ;
#9075=CARTESIAN_POINT ( 'NONE',  ( -3.980102097228897245E-16, 12.50000000000000000, -6.749999999999999112 ) ) ;
#9084=CARTESIAN_POINT ( 'NONE',  ( 3.249999999999999112, 11.81250000000000000, -2.153805922287439945 ) ) ;
#9086=CARTESIAN_POINT ( 'NONE',  ( -3.980102097228897245E-16, 5.500000000000000000, -6.749999999999999112 ) ) ;
#9088=CARTESIAN_POINT ( 'NONE',  ( -3.749999999999999556, 0.7500000000000001110, -3.499999999999999112 ) ) ;
#9092=CARTESIAN_POINT ( 'NONE',  ( 3.749999999999999112, 6.812500000000000000, -1.946699141100892039 ) ) ;
#9099=CARTESIAN_POINT ( 'NONE',  ( 2.298097038856278029, 2.125000000000000000, -5.798097038856279362 ) ) ;
#9103=CARTESIAN_POINT ( 'NONE',  ( 3.749999999999998668, 11.18750000000000178, -5.053300858899108405 ) ) ;
#9104=CARTESIAN_POINT ( 'NONE',  ( -1.553300858899106407, 14.06250000000000178, 0.2500000000000002220 ) ) ;
#9108=CARTESIAN_POINT ( 'NONE',  ( -3.980102097228897738E-16, 1.000000000000000000, -6.749999999999999112 ) ) ;
#9115=CARTESIAN_POINT ( 'NONE',  ( -3.249999999999999556, 4.750000000000000888, -3.500000000000000000 ) ) ;
#9123=CARTESIAN_POINT ( 'NONE',  ( 2.298097038856279362, 14.37500000000000000, -1.201902961143720860 ) ) ;
#9127=CARTESIAN_POINT ( 'NONE',  ( -2.651650429449552870, 0.6250000000000002220, -0.8483495705504463524 ) ) ;
#9132=CARTESIAN_POINT ( 'NONE',  ( -1.346194077712559389, 14.43750000000000000, -6.749999999999999112 ) ) ;
#9136=CARTESIAN_POINT ( 'NONE',  ( -3.249999999999999556, 9.187500000000000000, -2.153805922287440833 ) ) ;
#9143=CARTESIAN_POINT ( 'NONE',  ( -1.553300858899106629, 2.062500000000000000, 0.2500000000000002220 ) ) ;
#9144=CARTESIAN_POINT ( 'NONE',  ( -3.249999999999999112, 14.68750000000000178, -2.153805922287440833 ) ) ;
#9147=CARTESIAN_POINT ( 'NONE',  ( 0.000000000000000000, 15.00000000000000000, -0.2500000000000002220 ) ) ;
#9160=CARTESIAN_POINT ( 'NONE',  ( -2.298097038856278918, 11.37500000000000000, -5.798097038856277585 ) ) ;
#9164=CARTESIAN_POINT ( 'NONE',  ( 0.000000000000000000, 5.000000000000000000, -0.2500000000000002220 ) ) ;
#9166=CARTESIAN_POINT ( 'NONE',  ( 3.750000000000000000, 0.3125000000000002220, -1.946699141100892705 ) ) ;
#9167=CARTESIAN_POINT ( 'NONE',  ( -1.346194077712558945, 6.562500000000000888, -0.2500000000000002220 ) ) ;
#9171=CARTESIAN_POINT ( 'NONE',  ( -1.553300858899106629, 6.062500000000000000, 0.2500000000000002220 ) ) ;
#9178=CARTESIAN_POINT ( 'NONE',  ( -3.249999999999999112, 5.812500000000000888, -4.846194077712558723 ) ) ;
#9181=CARTESIAN_POINT ( 'NONE',  ( 3.749999999999999112, 11.31250000000000355, -1.946699141100893149 ) ) ;
#9182=CARTESIAN_POINT ( 'NONE',  ( 0.000000000000000000, 14.00000000000000000, 0.2500000000000002220 ) ) ;
#9185=CARTESIAN_POINT ( 'NONE',  ( -3.750000000000000000, 12.81250000000000178, -5.053300858899105741 ) ) ;
#9191=CARTESIAN_POINT ( 'NONE',  ( -3.249999999999999556, 0.3125000000000000555, -4.846194077712557835 ) ) ;
#9196=CARTESIAN_POINT ( 'NONE',  ( 0.000000000000000000, 2.500000000000000000, -0.2500000000000002220 ) ) ;
#9202=CARTESIAN_POINT ( 'NONE',  ( -3.980102097228897738E-16, 13.00000000000000000, -6.749999999999999112 ) ) ;
#9204=CARTESIAN_POINT ( 'NONE',  ( -1.553300858899106629, 2.562500000000000444, 0.2500000000000002220 ) ) ;
#9205=VECTOR ( 'NONE', #9870, 1000.000000000000000 ) ;
#9210=CARTESIAN_POINT ( 'NONE',  ( 1.346194077712560944, 8.937500000000001776, -0.2500000000000010547 ) ) ;
#9216=CARTESIAN_POINT ( 'NONE',  ( -4.592425496802573972E-16, 5.500000000000000000, -7.249999999999999112 ) ) ;
#9218=CARTESIAN_POINT ( 'NONE',  ( -3.980102097228897738E-16, 14.00000000000000000, -6.749999999999999112 ) ) ;
#9223=CARTESIAN_POINT ( 'NONE',  ( -3.980102097228897738E-16, 1.000000000000000000, -6.749999999999999112 ) ) ;
#9226=DIRECTION ( 'NONE',  ( 0.000000000000000000, 0.000000000000000000, 1.000000000000000000 ) ) ;
#9227=CARTESIAN_POINT ( 'NONE',  ( 2.298097038856278473, 5.625000000000000000, -5.798097038856279362 ) ) ;
#9236=CARTESIAN_POINT ( 'NONE',  ( 0.000000000000000000, 12.00000000000000000, -0.2500000000000002220 ) ) ;
#9240=CARTESIAN_POINT ( 'NONE',  ( -3.749999999999999556, 11.75000000000000178, -3.499999999999999112 ) ) ;
#9242=CARTESIAN_POINT ( 'NONE',  ( -3.750000000000000000, 2.812500000000000444, -5.053300858899105741 ) ) ;
#9244=CARTESIAN_POINT ( 'NONE',  ( 3.249999999999998224, 7.312500000000001776, -2.153805922287439945 ) ) ;
#9249=CARTESIAN_POINT ( 'NONE',  ( -3.980102097228897245E-16, 3.500000000000000000, -6.749999999999999112 ) ) ;
#9250=CARTESIAN_POINT ( 'NONE',  ( 2.651650429449552870, 7.625000000000000000, -6.151650429449554203 ) ) ;
#9256=CARTESIAN_POINT ( 'NONE',  ( -1.346194077712559167, 5.937500000000000000, -6.749999999999999112 ) ) ;
#9259=CARTESIAN_POINT ( 'NONE',  ( 3.749999999999999112, 10.31250000000000000, -1.946699141100893149 ) ) ;
#9260=CARTESIAN_POINT ( 'NONE',  ( -2.651650429449552870, 13.12500000000000000, -0.8483495705504462414 ) ) ;
#9262=CARTESIAN_POINT ( 'NONE',  ( -0.1260096660175019090, -0.1954009359728117456, 0.1491815183709511716 ) ) ;
#9263=CARTESIAN_POINT ( 'NONE',  ( -3.249999999999999556, 8.187500000000000000, -2.153805922287440833 ) ) ;
#9264=CARTESIAN_POINT ( 'NONE',  ( -3.249999999999999112, -0.1874999999999998890, -4.846194077712558723 ) ) ;
#9271=CARTESIAN_POINT ( 'NONE',  ( 1.346194077712560944, 3.937500000000000000, -0.2500000000000011102 ) ) ;
#9273=CARTESIAN_POINT ( 'NONE',  ( 3.249999999999999556, 2.249999999999999556, -3.500000000000000000 ) ) ;
#9279=CARTESIAN_POINT ( 'NONE',  ( -3.249999999999999112, 11.68749999999999822, -2.153805922287440833 ) ) ;
#9282=CARTESIAN_POINT ( 'NONE',  ( 0.000000000000000000, 0.5000000000000001110, 0.2500000000000002220 ) ) ;
#9287=CARTESIAN_POINT ( 'NONE',  ( -2.298097038856278473, 13.12500000000000000, -1.201902961143720416 ) ) ;
#9290=EDGE_LOOP ( 'NONE', ( #13699, #12224, #10595, #11536 ) ) ;
#9292=CARTESIAN_POINT ( 'NONE',  ( -0.3766621274091715987, -0.2500000000000000000, -7.146945437571387671 ) ) ;
#9293=CARTESIAN_POINT ( 'NONE',  ( 1.553300858899108849, 5.937500000000000000, 0.2499999999999993616 ) ) ;
#9294=CARTESIAN_POINT ( 'NONE',  ( -1.553300858899106629, 5.562500000000000000, 0.2499999999999998335 ) ) ;
#9297=CARTESIAN_POINT ( 'NONE',  ( -2.298097038856279362, 1.874999999999999778, -5.798097038856278473 ) ) ;
#9303=CARTESIAN_POINT ( 'NONE',  ( -1.346194077712559389, 2.437500000000000444, -6.749999999999999112 ) ) ;
#9309=CARTESIAN_POINT ( 'NONE',  ( 2.298097038856278473, 10.62500000000000000, -5.798097038856279362 ) ) ;
#9312=CARTESIAN_POINT ( 'NONE',  ( 1.553300858899109516, 9.437500000000000000, 0.2499999999999993616 ) ) ;
#9314=SHAPE_REPRESENTATION ( 'SmallSpring', ( #9419 ), #6710 ) ;
#9315=CARTESIAN_POINT ( 'NONE',  ( 0.000000000000000000, 7.500000000000000888, 0.2500000000000002220 ) ) ;
#9317=CARTESIAN_POINT ( 'NONE',  ( 3.249999999999999556, 8.250000000000000000, -3.500000000000000000 ) ) ;
#9318=ORIENTED_EDGE ( 'NONE', *, *, #10561, .T. ) ;
#9320=CARTESIAN_POINT ( 'NONE',  ( -3.249999999999999556, 3.312500000000000000, -4.846194077712557835 ) ) ;
#9321=CARTESIAN_POINT ( 'NONE',  ( -3.749999999999999556, 4.312500000000000888, -5.053300858899104853 ) ) ;
#9332=CARTESIAN_POINT ( 'NONE',  ( -3.980102097228897738E-16, 8.000000000000000000, -6.749999999999999112 ) ) ;
#9334=CARTESIAN_POINT ( 'NONE',  ( -2.651650429449552870, 8.625000000000000000, -0.8483495705504467965 ) ) ;
#9335=CARTESIAN_POINT ( 'NONE',  ( -3.750000000000000000, 12.31250000000000000, -5.053300858899105741 ) ) ;
#9338=CARTESIAN_POINT ( 'NONE',  ( -1.346194077712559167, -0.06249999999999988898, -6.749999999999999112 ) ) ;
#9344=CARTESIAN_POINT ( 'NONE',  ( 0.3766621274091715987, -0.2500000000000000000, -6.863050255469941519 ) ) ;
#9345=CARTESIAN_POINT ( 'NONE',  ( -1.346194077712558945, 2.062500000000000000, -0.2500000000000002220 ) ) ;
#9346=CARTESIAN_POINT ( 'NONE',  ( 3.249999999999998224, 7.187500000000000888, -4.846194077712561388 ) ) ;
#9351=CARTESIAN_POINT ( 'NONE',  ( -3.249999999999999112, 10.81250000000000000, -4.846194077712558723 ) ) ;
#9353=CARTESIAN_POINT ( 'NONE',  ( -1.553300858899107073, 2.937500000000000444, -7.249999999999999112 ) ) ;
#9355=DIRECTION ( 'NONE',  ( 1.000000000000000000, 0.000000000000000000, 0.000000000000000000 ) ) ;
#9358=CARTESIAN_POINT ( 'NONE',  ( -2.298097038856278918, 11.37500000000000000, -5.798097038856277585 ) ) ;
#9364=CARTESIAN_POINT ( 'NONE',  ( -2.651650429449552870, 5.125000000000000000, -0.8483495705504462414 ) ) ;
#9365=CARTESIAN_POINT ( 'NONE',  ( -2.651650429449552870, 5.875000000000000888, -6.151650429449552426 ) ) ;
#9368=CARTESIAN_POINT ( 'NONE',  ( 3.249999999999999556, 1.249999999999999778, -3.500000000000000000 ) ) ;
#9373=CARTESIAN_POINT ( 'NONE',  ( 2.298097038856279362, 2.875000000000000000, -1.201902961143720860 ) ) ;
#9386=CARTESIAN_POINT ( 'NONE',  ( -2.651650429449552870, 4.625000000000000888, -0.8483495705504463524 ) ) ;
#9387=CARTESIAN_POINT ( 'NONE',  ( 3.249999999999998224, 5.312500000000000000, -2.153805922287439945 ) ) ;
#9393=CARTESIAN_POINT ( 'NONE',  ( -3.980102097228897245E-16, 4.500000000000000888, -6.749999999999999112 ) ) ;
#9396=CARTESIAN_POINT ( 'NONE',  ( 3.749999999999999112, 8.812500000000000000, -1.946699141100892039 ) ) ;
#9406=CARTESIAN_POINT ( 'NONE',  ( 3.249999999999998224, 7.312500000000000000, -2.153805922287439945 ) ) ;
#9409=CARTESIAN_POINT ( 'NONE',  ( -3.750000000000000000, 11.68749999999999822, -1.946699141100893149 ) ) ;
#9413=CARTESIAN_POINT ( 'NONE',  ( -1.553300858899107073, 12.93750000000000178, -7.249999999999999112 ) ) ;
#9417=CARTESIAN_POINT ( 'NONE',  ( 3.249999999999999112, 14.81250000000000000, -2.153805922287439945 ) ) ;
#9419=AXIS2_PLACEMENT_3D ( 'NONE', #15272, #9226, #12943 ) ;
#9422=CARTESIAN_POINT ( 'NONE',  ( -2.298097038856278918, 1.375000000000000000, -5.798097038856277585 ) ) ;
#9424=CARTESIAN_POINT ( 'NONE',  ( -1.346194077712558945, 5.562500000000001776, -0.2500000000000002220 ) ) ;
#9430=CARTESIAN_POINT ( 'NONE',  ( 3.249999999999999112, 1.812500000000000222, -2.153805922287439945 ) ) ;
#9431=CARTESIAN_POINT ( 'NONE',  ( 2.298097038856279362, 12.37500000000000178, -1.201902961143720860 ) ) ;
#9434=CARTESIAN_POINT ( 'NONE',  ( -1.553300858899106629, 3.562500000000000888, 0.2500000000000002220 ) ) ;
#9439=CARTESIAN_POINT ( 'NONE',  ( 2.298097038856278473, 11.62500000000000000, -5.798097038856279362 ) ) ;
#9445=CARTESIAN_POINT ( 'NONE',  ( -0.3766621274091715987, 0.5000000000000000000, -0.1347136637304948981 ) ) ;
#9446=CARTESIAN_POINT ( 'NONE',  ( 3.749999999999999112, 4.812500000000000888, -1.946699141100892039 ) ) ;
#9447=CARTESIAN_POINT ( 'NONE',  ( 3.749999999999999112, 5.312500000000000000, -1.946699141100893149 ) ) ;
#9453=CARTESIAN_POINT ( 'NONE',  ( -1.346194077712559389, 13.43749999999999822, -6.749999999999999112 ) ) ;
#9457=CARTESIAN_POINT ( 'NONE',  ( -2.298097038856278473, 4.125000000000000000, -1.201902961143720416 ) ) ;
#9468=CARTESIAN_POINT ( 'NONE',  ( -2.651650429449552870, 5.625000000000000888, -0.8483495705504463524 ) ) ;
#9469=CARTESIAN_POINT ( 'NONE',  ( -2.298097038856279362, 5.875000000000001776, -5.798097038856278473 ) ) ;
#9472=CARTESIAN_POINT ( 'NONE',  ( 1.346194077712560944, 1.937500000000000000, -0.2500000000000010547 ) ) ;
#9479=B_SPLINE_CURVE_WITH_KNOTS ( 'NONE', 3,
 ( #10903, #13472, #9901, #2875 ),
 .UNSPECIFIED., .F., .F.,
 ( 4, 4 ),
 ( 4.512482785797534139E-18, 0.0003024267748246941591 ),
 .UNSPECIFIED. ) ;
#9483=CARTESIAN_POINT ( 'NONE',  ( -2.651650429449552870, 11.87500000000000000, -6.151650429449552426 ) ) ;
#9487=CARTESIAN_POINT ( 'NONE',  ( -1.346194077712559167, 3.937500000000001332, -6.749999999999999112 ) ) ;
#9496=CARTESIAN_POINT ( 'NONE',  ( -2.298097038856278473, 3.125000000000000000, -1.201902961143720416 ) ) ;
#9499=CARTESIAN_POINT ( 'NONE',  ( 1.346194077712558057, 11.56249999999999822, -6.750000000000000000 ) ) ;
#9500=CARTESIAN_POINT ( 'NONE',  ( 3.249999999999998224, 6.312500000000000000, -2.153805922287439945 ) ) ;
#9505=CARTESIAN_POINT ( 'NONE',  ( -1.346194077712559389, 2.062500000000000000, -0.2500000000000002220 ) ) ;
#9506=CARTESIAN_POINT ( 'NONE',  ( -3.750000000000000000, 0.6875000000000000000, -1.946699141100893149 ) ) ;
#9507=CARTESIAN_POINT ( 'NONE',  ( 3.750000000000000000, 3.750000000000000000, -3.500000000000000444 ) ) ;
#9508=CARTESIAN_POINT ( 'NONE',  ( -0.2508417382212070335, 0.2913627682709560296, -7.146945437571385895 ) ) ;
#9509=CARTESIAN_POINT ( 'NONE',  ( 0.000000000000000000, 6.500000000000000000, 0.2500000000000002220 ) ) ;
#9517=CARTESIAN_POINT ( 'NONE',  ( 1.346194077712560944, 12.93750000000000000, -0.2500000000000010547 ) ) ;
#9523=FACE_OUTER_BOUND ( 'NONE', #3137, .T. ) ;
#9524=CARTESIAN_POINT ( 'NONE',  ( -3.749999999999999556, 5.312500000000001776, -5.053300858899104853 ) ) ;
#9525=CARTESIAN_POINT ( 'NONE',  ( 3.749999999999999112, 2.312500000000000000, -1.946699141100893149 ) ) ;
#9528=ORIENTED_EDGE ( 'NONE', *, *, #8813, .T. ) ;
#9529=CARTESIAN_POINT ( 'NONE',  ( 3.249999999999998224, 5.312500000000000000, -2.153805922287439945 ) ) ;
#9532=CARTESIAN_POINT ( 'NONE',  ( 0.000000000000000000, 10.00000000000000000, -0.2500000000000002220 ) ) ;
#9543=CARTESIAN_POINT ( 'NONE',  ( -1.553300858899107073, 4.937500000000000888, -7.249999999999999112 ) ) ;
#9544=CARTESIAN_POINT ( 'NONE',  ( 3.249999999999998224, 9.187500000000001776, -4.846194077712561388 ) ) ;
#9547=CARTESIAN_POINT ( 'NONE',  ( 0.000000000000000000, 5.000000000000000000, -0.2500000000000002220 ) ) ;
#9555=CARTESIAN_POINT ( 'NONE',  ( 0.000000000000000000, 14.50000000000000355, 0.2499999999999998057 ) ) ;
#9559=CARTESIAN_POINT ( 'NONE',  ( -1.346194077712558945, 4.562500000000000000, -0.2500000000000002220 ) ) ;
#9562=CARTESIAN_POINT ( 'NONE',  ( 3.249999999999998668, 14.68750000000000000, -4.846194077712560500 ) ) ;
#9566=CARTESIAN_POINT ( 'NONE',  ( 3.249999999999998668, 2.687500000000000444, -4.846194077712560500 ) ) ;
#9568=CARTESIAN_POINT ( 'NONE',  ( 1.346194077712560944, 12.93750000000000000, -0.2500000000000010547 ) ) ;
#9569=CARTESIAN_POINT ( 'NONE',  ( -2.298097038856279362, 7.874999999999999112, -5.798097038856278473 ) ) ;
#9575=CARTESIAN_POINT ( 'NONE',  ( 2.298097038856278473, 0.6250000000000000000, -5.798097038856279362 ) ) ;
#9576=CARTESIAN_POINT ( 'NONE',  ( -1.553300858899107073, 0.9375000000000000000, -7.249999999999999112 ) ) ;
#9577=CARTESIAN_POINT ( 'NONE',  ( 2.651650429449553759, 5.875000000000000000, -0.8483495705504471296 ) ) ;
#9579=CARTESIAN_POINT ( 'NONE',  ( -1.553300858899107073, 5.937500000000002665, -7.249999999999999112 ) ) ;
#9585=CARTESIAN_POINT ( 'NONE',  ( 2.298097038856279362, 12.87500000000000178, -1.201902961143720860 ) ) ;
#9589=CARTESIAN_POINT ( 'NONE',  ( 3.750000000000000000, 9.312500000000000000, -1.946699141100892705 ) ) ;
#9593=CARTESIAN_POINT ( 'NONE',  ( 3.749999999999999112, 8.812500000000000000, -1.946699141100892039 ) ) ;
#9594=CARTESIAN_POINT ( 'NONE',  ( 2.651650429449553314, 2.375000000000000000, -0.8483495705504476847 ) ) ;
#9599=CARTESIAN_POINT ( 'NONE',  ( 0.000000000000000000, 2.500000000000000000, -0.2500000000000002220 ) ) ;
#9604=CARTESIAN_POINT ( 'NONE',  ( 2.298097038856278473, 6.625000000000000000, -5.798097038856279362 ) ) ;
#9610=CARTESIAN_POINT ( 'NONE',  ( -0.3766621274091715987, 0.5000000000000000000, 0.1491815183709511716 ) ) ;
#9615=CARTESIAN_POINT ( 'NONE',  ( -3.750000000000000000, 4.812500000000001776, -5.053300858899105741 ) ) ;
#9616=CARTESIAN_POINT ( 'NONE',  ( -1.346194077712558945, 9.562500000000000000, -0.2500000000000002220 ) ) ;
#9619=CARTESIAN_POINT ( 'NONE',  ( -1.346194077712559389, 6.062500000000000000, -0.2500000000000002220 ) ) ;
#9631=CARTESIAN_POINT ( 'NONE',  ( -2.298097038856278918, 1.375000000000000000, -5.798097038856277585 ) ) ;
#9634=CARTESIAN_POINT ( 'NONE',  ( 1.553300858899105963, 14.06250000000000178, -7.249999999999999112 ) ) ;
#9638=CARTESIAN_POINT ( 'NONE',  ( -3.980102097228897738E-16, 3.000000000000000444, -6.749999999999999112 ) ) ;
#9648=CARTESIAN_POINT ( 'NONE',  ( 3.249999999999999112, 8.812500000000000000, -2.153805922287439945 ) ) ;
#9650=CARTESIAN_POINT ( 'NONE',  ( 2.298097038856279362, 13.87500000000000000, -1.201902961143720860 ) ) ;
#9652=CARTESIAN_POINT ( 'NONE',  ( -2.298097038856278029, 7.625000000000001776, -1.201902961143720638 ) ) ;
#9656=CARTESIAN_POINT ( 'NONE',  ( -2.298097038856278918, 1.375000000000000000, -5.798097038856277585 ) ) ;
#9657=CARTESIAN_POINT ( 'NONE',  ( -3.750000000000000000, 2.812500000000000444, -5.053300858899105741 ) ) ;
#9658=CARTESIAN_POINT ( 'NONE',  ( 3.749999999999999112, 4.687500000000000888, -5.053300858899108405 ) ) ;
#9660=CARTESIAN_POINT ( 'NONE',  ( 2.651650429449554203, 6.375000000000000888, -0.8483495705504471296 ) ) ;
#9667=PLANE ( 'NONE',  #12100 ) ;
#9672=CARTESIAN_POINT ( 'NONE',  ( 1.553300858899109516, 8.437500000000000000, 0.2499999999999993616 ) ) ;
#9676=CARTESIAN_POINT ( 'NONE',  ( -3.749999999999999556, 7.187500000000000000, -1.946699141100892927 ) ) ;
#9677=CARTESIAN_POINT ( 'NONE',  ( 3.749999999999999112, 7.312500000000000000, -1.946699141100893149 ) ) ;
#9682=CARTESIAN_POINT ( 'NONE',  ( 3.249999999999998224, 5.187499999999999112, -4.846194077712561388 ) ) ;
#9683=CARTESIAN_POINT ( 'NONE',  ( -1.553300858899106629, 11.06250000000000000, 0.2500000000000002220 ) ) ;
#9686=CARTESIAN_POINT ( 'NONE',  ( 0.000000000000000000, 9.000000000000001776, -0.2500000000000002220 ) ) ;
#9695=CARTESIAN_POINT ( 'NONE',  ( -3.980102097228897245E-16, 13.50000000000000000, -6.749999999999999112 ) ) ;
#9699=CARTESIAN_POINT ( 'NONE',  ( 0.000000000000000000, 14.50000000000000355, 0.2499999999999998057 ) ) ;
#9701=CARTESIAN_POINT ( 'NONE',  ( -2.298097038856279362, 6.875000000000000000, -5.798097038856278473 ) ) ;
#9702=CARTESIAN_POINT ( 'NONE',  ( 0.000000000000000000, 11.50000000000000000, -0.2500000000000002220 ) ) ;
#9705=CARTESIAN_POINT ( 'NONE',  ( -1.346194077712559389, 5.062500000000001776, -0.2500000000000002220 ) ) ;
#9716=VERTEX_POINT ( 'NONE', #3499 ) ;
#9717=CARTESIAN_POINT ( 'NONE',  ( -1.346194077712559167, 13.93750000000000000, -6.749999999999999112 ) ) ;
#9718=CARTESIAN_POINT ( 'NONE',  ( -3.750000000000000000, 13.25000000000000000, -3.499999999999999112 ) ) ;
#9722=CARTESIAN_POINT ( 'NONE',  ( -3.750000000000000000, 11.81250000000000178, -5.053300858899105741 ) ) ;
#9726=CARTESIAN_POINT ( 'NONE',  ( 1.346194077712558279, 4.062500000000001776, -6.750000000000000888 ) ) ;
#9729=CARTESIAN_POINT ( 'NONE',  ( 0.000000000000000000, 15.00000000000000000, 0.2500000000000002220 ) ) ;
#9735=CARTESIAN_POINT ( 'NONE',  ( 3.249999999999999556, 7.750000000000000000, -3.500000000000000000 ) ) ;
#9737=CARTESIAN_POINT ( 'NONE',  ( -3.249999999999999556, 13.18749999999999822, -2.153805922287440833 ) ) ;
#9738=CARTESIAN_POINT ( 'NONE',  ( -2.298097038856278029, 9.624999999999998224, -1.201902961143720638 ) ) ;
#9742=CARTESIAN_POINT ( 'NONE',  ( 3.249999999999999112, 2.812500000000000000, -2.153805922287439945 ) ) ;
#9744=CARTESIAN_POINT ( 'NONE',  ( -2.298097038856278029, 14.62500000000000178, -1.201902961143720638 ) ) ;
#9745=CARTESIAN_POINT ( 'NONE',  ( 3.750000000000000000, 4.750000000000000000, -3.500000000000000444 ) ) ;
#9747=CARTESIAN_POINT ( 'NONE',  ( -1.553300858899107073, 7.937500000000001776, -7.249999999999999112 ) ) ;
#9756=VERTEX_POINT ( 'NONE', #3271 ) ;
#9757=CARTESIAN_POINT ( 'NONE',  ( -4.592425496802573972E-16, 10.00000000000000000, -7.250000000000000000 ) ) ;
#9760=CARTESIAN_POINT ( 'NONE',  ( -3.749999999999999556, 9.312499999999998224, -5.053300858899104853 ) ) ;
#9761=CARTESIAN_POINT ( 'NONE',  ( -3.750000000000000000, 9.812500000000000000, -5.053300858899105741 ) ) ;
#9764=CARTESIAN_POINT ( 'NONE',  ( -3.249999999999999112, 4.687500000000000000, -2.153805922287440833 ) ) ;
#9765=CARTESIAN_POINT ( 'NONE',  ( -2.651650429449552870, 9.125000000000000000, -0.8483495705504462414 ) ) ;
#9768=CARTESIAN_POINT ( 'NONE',  ( -1.346194077712559389, 8.062500000000000000, -0.2500000000000002220 ) ) ;
#9773=DIRECTION ( 'NONE',  ( 0.000000000000000000, 0.000000000000000000, -1.000000000000000000 ) ) ;
#9778=CARTESIAN_POINT ( 'NONE',  ( 3.749999999999999556, 11.25000000000000178, -3.500000000000000444 ) ) ;
#9779=CARTESIAN_POINT ( 'NONE',  ( 3.249999999999998224, 13.18750000000000000, -4.846194077712561388 ) ) ;
#9780=CARTESIAN_POINT ( 'NONE',  ( 1.346194077712561166, 9.437500000000000000, -0.2500000000000011102 ) ) ;
#9784=CARTESIAN_POINT ( 'NONE',  ( 0.000000000000000000, 6.000000000000000000, -0.2500000000000002220 ) ) ;
#9789=DIRECTION ( 'NONE',  ( 1.000000000000000000, 0.000000000000000000, 0.000000000000000000 ) ) ;
#9793=CARTESIAN_POINT ( 'NONE',  ( 3.249999999999999112, 9.812500000000000000, -2.153805922287439945 ) ) ;
#9794=CARTESIAN_POINT ( 'NONE',  ( 1.346194077712558279, 14.06250000000000178, -6.750000000000000888 ) ) ;
#9795=CARTESIAN_POINT ( 'NONE',  ( -3.750000000000000000, 14.25000000000000000, -3.499999999999999112 ) ) ;
#9797=CARTESIAN_POINT ( 'NONE',  ( 3.749999999999999112, 3.812500000000000000, -1.946699141100892039 ) ) ;
#9807=CARTESIAN_POINT ( 'NONE',  ( 1.346194077712560944, 5.937500000000000000, -0.2500000000000011102 ) ) ;
#9809=CARTESIAN_POINT ( 'NONE',  ( -3.249999999999999556, 14.18750000000000000, -2.153805922287440833 ) ) ;
#9810=CARTESIAN_POINT ( 'NONE',  ( -3.249999999999999112, 9.812500000000000000, -4.846194077712558723 ) ) ;
#9815=CARTESIAN_POINT ( 'NONE',  ( 1.346194077712560944, 5.937500000000000000, -0.2500000000000010547 ) ) ;
#9816=CARTESIAN_POINT ( 'NONE',  ( 3.749999999999998668, 3.187500000000000444, -5.053300858899108405 ) ) ;
#9818=CARTESIAN_POINT ( 'NONE',  ( 0.000000000000000000, 10.00000000000000000, 0.2500000000000002220 ) ) ;
#9820=CARTESIAN_POINT ( 'NONE',  ( 2.651650429449554203, 7.375000000000000000, -0.8483495705504471296 ) ) ;
#9828=CARTESIAN_POINT ( 'NONE',  ( 1.346194077712561166, 0.4375000000000000555, -0.2500000000000011102 ) ) ;
#9832=CARTESIAN_POINT ( 'NONE',  ( -1.553300858899107295, 8.437500000000000000, -7.250000000000000000 ) ) ;
#9833=CARTESIAN_POINT ( 'NONE',  ( -4.592425496802573972E-16, 8.999999999999998224, -7.250000000000000000 ) ) ;
#9836=CARTESIAN_POINT ( 'NONE',  ( 3.249999999999998224, 4.187500000000000888, -4.846194077712561388 ) ) ;
#9837=CARTESIAN_POINT ( 'NONE',  ( -1.553300858899106629, 8.062500000000000000, 0.2500000000000002220 ) ) ;
#9841=CARTESIAN_POINT ( 'NONE',  ( -3.249999999999999556, 8.250000000000000000, -3.499999999999999556 ) ) ;
#9851=CARTESIAN_POINT ( 'NONE',  ( -1.553300858899106629, 13.56250000000000000, 0.2499999999999998335 ) ) ;
#9852=CARTESIAN_POINT ( 'NONE',  ( -1.346194077712559167, 11.93750000000000178, -6.749999999999999112 ) ) ;
#9853=CARTESIAN_POINT ( 'NONE',  ( -3.249999999999999556, 11.75000000000000178, -3.500000000000000000 ) ) ;
#9856=CARTESIAN_POINT ( 'NONE',  ( 2.298097038856278473, 8.625000000000000000, -5.798097038856279362 ) ) ;
#9860=DIRECTION ( 'NONE',  ( 0.000000000000000000, 0.000000000000000000, 1.000000000000000000 ) ) ;
#9866=CARTESIAN_POINT ( 'NONE',  ( -1.346194077712558945, 13.56250000000000000, -0.2500000000000002220 ) ) ;
#9867=CARTESIAN_POINT ( 'NONE',  ( -4.592425496802573972E-16, 13.50000000000000000, -7.249999999999999112 ) ) ;
#9870=DIRECTION ( 'NONE',  ( -1.000000000000000000, -0.000000000000000000, -0.000000000000000000 ) ) ;
#9872=CARTESIAN_POINT ( 'NONE',  ( -3.750000000000000000, 1.250000000000000000, -3.499999999999999112 ) ) ;
#9881=CARTESIAN_POINT ( 'NONE',  ( 1.346194077712558279, 6.562500000000000000, -6.750000000000000000 ) ) ;
#9883=CARTESIAN_POINT ( 'NONE',  ( -3.980102097228897245E-16, 13.50000000000000000, -6.749999999999999112 ) ) ;
#9884=CARTESIAN_POINT ( 'NONE',  ( 3.249999999999999556, 12.25000000000000000, -3.500000000000000000 ) ) ;
#9889=CARTESIAN_POINT ( 'NONE',  ( -3.980102097228897245E-16, 6.500000000000000888, -6.749999999999999112 ) ) ;
#9890=CARTESIAN_POINT ( 'NONE',  ( 3.749999999999999112, 7.312500000000000000, -1.946699141100893149 ) ) ;
#9892=VECTOR ( 'NONE', #12116, 1000.000000000000000 ) ;
#9893=CARTESIAN_POINT ( 'NONE',  ( -4.592425496802573972E-16, 7.500000000000000000, -7.249999999999999112 ) ) ;
#9895=CARTESIAN_POINT ( 'NONE',  ( -3.750000000000000000, 10.81250000000000000, -5.053300858899105741 ) ) ;
#9901=CARTESIAN_POINT ( 'NONE',  ( -0.3766621274091710991, 0.2295137623791638215, -7.070595193497560160 ) ) ;
#9907=CARTESIAN_POINT ( 'NONE',  ( -1.553300858899107073, 12.93750000000000178, -7.249999999999999112 ) ) ;
#9911=CARTESIAN_POINT ( 'NONE',  ( -4.592425496802573972E-16, 8.500000000000000000, -7.249999999999999112 ) ) ;
#9912=CARTESIAN_POINT ( 'NONE',  ( 3.749999999999998668, 9.187500000000001776, -5.053300858899108405 ) ) ;
#9916=CARTESIAN_POINT ( 'NONE',  ( -3.249999999999999112, 8.687500000000003553, -2.153805922287440833 ) ) ;
#9917=CARTESIAN_POINT ( 'NONE',  ( -2.651650429449553314, 8.375000000000000000, -6.151650429449552426 ) ) ;
#9921=CARTESIAN_POINT ( 'NONE',  ( -1.346194077712559389, 10.43750000000000000, -6.749999999999999112 ) ) ;
#9925=CARTESIAN_POINT ( 'NONE',  ( 0.3766621274091715987, 0.2956834184403337451, -6.863050255469942407 ) ) ;
#9926=AXIS2_PLACEMENT_3D ( 'NONE', #7767, #12481, #4296 ) ;
#9929=CARTESIAN_POINT ( 'NONE',  ( -0.1260668993691365092, 0.2851798274189282778, -6.863050255469941519 ) ) ;
#9930=CARTESIAN_POINT ( 'NONE',  ( 0.000000000000000000, 12.50000000000000178, 0.2499999999999998057 ) ) ;
#9931=CARTESIAN_POINT ( 'NONE',  ( -2.298097038856278029, 10.62500000000000178, -1.201902961143720638 ) ) ;
#9932=CARTESIAN_POINT ( 'NONE',  ( 3.249999999999998224, 13.31250000000000178, -2.153805922287439945 ) ) ;
#9934=CARTESIAN_POINT ( 'NONE',  ( -3.980102097228897245E-16, 7.500000000000000000, -6.749999999999999112 ) ) ;
#9943=CARTESIAN_POINT ( 'NONE',  ( 0.000000000000000000, 14.50000000000000000, -0.2500000000000002220 ) ) ;
#9944=CARTESIAN_POINT ( 'NONE',  ( 1.553300858899105963, 13.56250000000000000, -7.250000000000000888 ) ) ;
#9947=CARTESIAN_POINT ( 'NONE',  ( -2.651650429449552870, 2.125000000000000000, -0.8483495705504462414 ) ) ;
#9951=CARTESIAN_POINT ( 'NONE',  ( -4.592425496802573972E-16, 2.500000000000000000, -7.249999999999999112 ) ) ;
#9954=FACE_OUTER_BOUND ( 'NONE', #968, .T. ) ;
#9956=CARTESIAN_POINT ( 'NONE',  ( 3.249999999999998668, 7.687500000000000000, -4.846194077712560500 ) ) ;
#9960=CARTESIAN_POINT ( 'NONE',  ( 2.298097038856278029, 4.125000000000000000, -5.798097038856279362 ) ) ;
#9961=CARTESIAN_POINT ( 'NONE',  ( -1.346194077712558945, 9.562500000000000000, -0.2500000000000002220 ) ) ;
#9964=CARTESIAN_POINT ( 'NONE',  ( -2.298097038856278473, 3.125000000000000000, -1.201902961143720416 ) ) ;
#9965=CARTESIAN_POINT ( 'NONE',  ( 1.553300858899105963, 4.062500000000001776, -7.249999999999999112 ) ) ;
#9966=CARTESIAN_POINT ( 'NONE',  ( -3.750000000000000000, 11.18750000000000000, -1.946699141100892927 ) ) ;
#9967=EDGE_CURVE ( 'NONE', #6060, #15209, #13247, .T. ) ;
#9970=CARTESIAN_POINT ( 'NONE',  ( 3.749999999999999556, 9.249999999999998224, -3.500000000000000444 ) ) ;
#9979=CARTESIAN_POINT ( 'NONE',  ( 3.749999999999999556, 12.25000000000000000, -3.500000000000000444 ) ) ;
#9980=ORIENTED_EDGE ( 'NONE', *, *, #4492, .T. ) ;
#9983=CARTESIAN_POINT ( 'NONE',  ( -1.553300858899106629, 11.06250000000000000, 0.2500000000000002220 ) ) ;
#9985=CARTESIAN_POINT ( 'NONE',  ( -3.750000000000000000, 6.812500000000000000, -5.053300858899105741 ) ) ;
#9988=CARTESIAN_POINT ( 'NONE',  ( 2.298097038856278029, 7.124999999999999112, -5.798097038856279362 ) ) ;
#9990=CARTESIAN_POINT ( 'NONE',  ( -3.750000000000000000, 12.25000000000000000, -3.499999999999999112 ) ) ;
#9994=DIRECTION ( 'NONE',  ( 1.000000000000000000, 0.000000000000000000, 0.000000000000000000 ) ) ;
#9996=CARTESIAN_POINT ( 'NONE',  ( 3.249999999999999556, 11.75000000000000000, -3.500000000000000000 ) ) ;
#10004=ORIENTED_EDGE ( 'NONE', *, *, #10732, .F. ) ;
#10008=CARTESIAN_POINT ( 'NONE',  ( 2.651650429449552870, 11.12500000000000178, -6.151650429449553314 ) ) ;
#10009=CARTESIAN_POINT ( 'NONE',  ( -2.298097038856278029, 11.62500000000000000, -1.201902961143720638 ) ) ;
#10010=CARTESIAN_POINT ( 'NONE',  ( 2.298097038856278029, 13.12499999999999822, -5.798097038856279362 ) ) ;
#10012=CARTESIAN_POINT ( 'NONE',  ( -3.980102097228897245E-16, 9.500000000000000000, -6.749999999999999112 ) ) ;
#10013=PLANE ( 'NONE',  #5209 ) ;
#10021=ORIENTED_EDGE ( 'NONE', *, *, #11469, .T. ) ;
#10022=CARTESIAN_POINT ( 'NONE',  ( 3.249999999999999556, 5.750000000000000000, -3.500000000000000000 ) ) ;
#10023=CARTESIAN_POINT ( 'NONE',  ( -1.553300858899106629, 13.06250000000000000, 0.2500000000000002220 ) ) ;
#10026=CARTESIAN_POINT ( 'NONE',  ( -2.651650429449553314, 0.3750000000000000555, -6.151650429449552426 ) ) ;
#10029=CARTESIAN_POINT ( 'NONE',  ( -4.592425496802573972E-16, 0.5000000000000000000, -7.249999999999999112 ) ) ;
#10034=CARTESIAN_POINT ( 'NONE',  ( 0.000000000000000000, 11.00000000000000000, -0.2500000000000002220 ) ) ;
#10035=CARTESIAN_POINT ( 'NONE',  ( 0.000000000000000000, 0.2105996885190176970, -0.1347136637304948981 ) ) ;
#10036=CARTESIAN_POINT ( 'NONE',  ( 1.346194077712558279, 5.062500000000000000, -6.750000000000000888 ) ) ;
#10037=CARTESIAN_POINT ( 'NONE',  ( -1.346194077712558945, 11.56250000000000178, -0.2500000000000002220 ) ) ;
#10040=CARTESIAN_POINT ( 'NONE',  ( -3.249999999999999556, 5.187500000000001776, -2.153805922287440833 ) ) ;
#10041=CARTESIAN_POINT ( 'NONE',  ( 3.749999999999999556, 4.249999999999999112, -3.500000000000000444 ) ) ;
#10042=CARTESIAN_POINT ( 'NONE',  ( 0.000000000000000000, 8.000000000000000000, 0.2500000000000002220 ) ) ;
#10044=DIRECTION ( 'NONE',  ( -0.000000000000000000, -0.000000000000000000, -1.000000000000000000 ) ) ;
#10047=CARTESIAN_POINT ( 'NONE',  ( 2.651650429449552870, 9.125000000000000000, -6.151650429449555091 ) ) ;
#10052=CARTESIAN_POINT ( 'NONE',  ( 1.346194077712558279, 0.5625000000000002220, -6.750000000000000000 ) ) ;
#10057=CARTESIAN_POINT ( 'NONE',  ( 3.750000000000000000, 14.31250000000000355, -1.946699141100892705 ) ) ;
#10058=ORIENTED_EDGE ( 'NONE', *, *, #13579, .T. ) ;
#10061=CARTESIAN_POINT ( 'NONE',  ( 3.749999999999999112, 10.31250000000000000, -1.946699141100893149 ) ) ;
#10064=CARTESIAN_POINT ( 'NONE',  ( -3.980102097228897738E-16, 8.999999999999998224, -6.749999999999999112 ) ) ;
#10066=CARTESIAN_POINT ( 'NONE',  ( -1.553300858899106629, 14.06249999999999822, 0.2500000000000002220 ) ) ;
#10070=CARTESIAN_POINT ( 'NONE',  ( -3.980102097228897245E-16, 12.50000000000000000, -6.749999999999999112 ) ) ;
#10071=CARTESIAN_POINT ( 'NONE',  ( -0.3766621274091715987, 0.2694895414731200423, 0.07352276961066842031 ) ) ;
#10080=CARTESIAN_POINT ( 'NONE',  ( 2.651650429449553759, 2.875000000000000000, -0.8483495705504471296 ) ) ;
#10081=CARTESIAN_POINT ( 'NONE',  ( 2.298097038856278029, 10.12500000000000000, -5.798097038856279362 ) ) ;
#10082=EDGE_CURVE ( 'NONE', #9716, #11175, #3727, .T. ) ;
#10083=CARTESIAN_POINT ( 'NONE',  ( 1.346194077712560944, 0.9374999999999998890, -0.2500000000000010547 ) ) ;
#10085=CARTESIAN_POINT ( 'NONE',  ( 2.298097038856279362, 10.87500000000000178, -1.201902961143720860 ) ) ;
#10094=CARTESIAN_POINT ( 'NONE',  ( 2.298097038856279362, 2.875000000000000000, -1.201902961143720860 ) ) ;
#10096=CARTESIAN_POINT ( 'NONE',  ( -2.651650429449553314, 2.875000000000000000, -6.151650429449552426 ) ) ;
#10100=CARTESIAN_POINT ( 'NONE',  ( -2.651650429449553314, 3.375000000000000000, -6.151650429449552426 ) ) ;
#10103=CARTESIAN_POINT ( 'NONE',  ( -1.553300858899106407, 0.06250000000000002776, 0.2500000000000002220 ) ) ;
#10110=CARTESIAN_POINT ( 'NONE',  ( 3.249999999999998224, 4.312500000000000000, -2.153805922287439945 ) ) ;
#10111=CARTESIAN_POINT ( 'NONE',  ( 1.346194077712558279, 13.06249999999999822, -6.750000000000000888 ) ) ;
#10114=CARTESIAN_POINT ( 'NONE',  ( -1.553300858899106629, 3.562500000000000888, 0.2499999999999998335 ) ) ;
#10115=CARTESIAN_POINT ( 'NONE',  ( -3.750000000000000000, 8.187500000000000000, -1.946699141100892927 ) ) ;
#10120=CARTESIAN_POINT ( 'NONE',  ( 1.553300858899105963, 12.06250000000000000, -7.250000000000000888 ) ) ;
#10128=CARTESIAN_POINT ( 'NONE',  ( 3.749999999999999112, 13.18750000000000000, -5.053300858899108405 ) ) ;
#10138=CARTESIAN_POINT ( 'NONE',  ( 0.000000000000000000, 9.500000000000001776, -0.2500000000000002220 ) ) ;
#10140=CARTESIAN_POINT ( 'NONE',  ( 3.750000000000000000, 13.75000000000000000, -3.500000000000000444 ) ) ;
#10146=CARTESIAN_POINT ( 'NONE',  ( 3.249999999999998668, 11.68750000000000000, -4.846194077712560500 ) ) ;
#10150=CARTESIAN_POINT ( 'NONE',  ( -1.346194077712559389, 8.062500000000000000, -0.2500000000000002220 ) ) ;
#10156=CARTESIAN_POINT ( 'NONE',  ( 3.749999999999999112, 1.812500000000000222, -1.946699141100892039 ) ) ;
#10157=CARTESIAN_POINT ( 'NONE',  ( -3.750000000000000000, 1.812499999999999778, -5.053300858899105741 ) ) ;
#10158=CARTESIAN_POINT ( 'NONE',  ( -3.249999999999999556, 1.187500000000000444, -2.153805922287440833 ) ) ;
#10161=CARTESIAN_POINT ( 'NONE',  ( -3.980102097228897245E-16, 10.50000000000000000, -6.749999999999999112 ) ) ;
#10174=CARTESIAN_POINT ( 'NONE',  ( 1.346194077712560944, 3.937500000000000000, -0.2500000000000010547 ) ) ;
#10176=CARTESIAN_POINT ( 'NONE',  ( 3.749999999999999112, 1.187500000000000222, -5.053300858899108405 ) ) ;
#10181=CARTESIAN_POINT ( 'NONE',  ( 2.651650429449552870, 4.625000000000000000, -6.151650429449554203 ) ) ;
#10193=CARTESIAN_POINT ( 'NONE',  ( -2.298097038856279362, 4.875000000000000000, -5.798097038856278473 ) ) ;
#10197=CARTESIAN_POINT ( 'NONE',  ( 3.749999999999999112, 4.312500000000000000, -1.946699141100893149 ) ) ;
#10198=CARTESIAN_POINT ( 'NONE',  ( 2.651650429449552870, 11.62500000000000000, -6.151650429449554203 ) ) ;
#10202=CARTESIAN_POINT ( 'NONE',  ( -1.553300858899107073, 10.93750000000000000, -7.249999999999999112 ) ) ;
#10211=CARTESIAN_POINT ( 'NONE',  ( 3.249999999999999556, 4.250000000000000000, -3.500000000000000000 ) ) ;
#10216=CARTESIAN_POINT ( 'NONE',  ( -1.346194077712559389, 10.43750000000000000, -6.749999999999999112 ) ) ;
#10219=CARTESIAN_POINT ( 'NONE',  ( 1.346194077712558279, 10.06250000000000000, -6.750000000000000888 ) ) ;
#10222=CARTESIAN_POINT ( 'NONE',  ( 0.000000000000000000, -0.4999999999999999445, 0.2500000000000002220 ) ) ;
#10225=CARTESIAN_POINT ( 'NONE',  ( 2.298097038856279362, 13.87500000000000000, -1.201902961143720860 ) ) ;
#10228=CARTESIAN_POINT ( 'NONE',  ( -2.298097038856278918, 10.37500000000000000, -5.798097038856277585 ) ) ;
#10235=CARTESIAN_POINT ( 'NONE',  ( -2.651650429449552870, 14.62500000000000178, -0.8483495705504467965 ) ) ;
#10236=CARTESIAN_POINT ( 'NONE',  ( 3.249999999999999556, 14.25000000000000178, -3.500000000000000000 ) ) ;
#10237=CARTESIAN_POINT ( 'NONE',  ( -3.249999999999999112, 13.68750000000000178, -2.153805922287440833 ) ) ;
#10239=CARTESIAN_POINT ( 'NONE',  ( 3.249999999999999556, 12.75000000000000178, -3.500000000000000000 ) ) ;
#10249=CARTESIAN_POINT ( 'NONE',  ( -3.980102097228897245E-16, 3.500000000000000000, -6.749999999999999112 ) ) ;
#10251=CARTESIAN_POINT ( 'NONE',  ( -2.651650429449552870, 2.625000000000000000, -0.8483495705504463524 ) ) ;
#10256=CARTESIAN_POINT ( 'NONE',  ( -2.651650429449553314, 6.375000000000000888, -6.151650429449552426 ) ) ;
#10262=CARTESIAN_POINT ( 'NONE',  ( -1.346194077712558945, 4.562500000000000000, -0.2500000000000002220 ) ) ;
#10265=CARTESIAN_POINT ( 'NONE',  ( 1.553300858899105963, 11.06250000000000178, -7.249999999999999112 ) ) ;
#10266=CARTESIAN_POINT ( 'NONE',  ( 2.651650429449552870, 13.62500000000000000, -6.151650429449554203 ) ) ;
#10268=ORIENTED_EDGE ( 'NONE', *, *, #161, .T. ) ;
#10270=CARTESIAN_POINT ( 'NONE',  ( -3.249999999999999112, 0.8125000000000001110, -4.846194077712558723 ) ) ;
#10279=CARTESIAN_POINT ( 'NONE',  ( -1.346194077712558945, 4.562500000000000000, -0.2500000000000002220 ) ) ;
#10281=CARTESIAN_POINT ( 'NONE',  ( 0.000000000000000000, 1.530808498934191509E-17, 0.000000000000000000 ) ) ;
#10287=CARTESIAN_POINT ( 'NONE',  ( -3.249999999999999112, 12.68750000000000178, -2.153805922287440833 ) ) ;
#10289=CARTESIAN_POINT ( 'NONE',  ( -1.553300858899106629, 12.06250000000000000, 0.2500000000000002220 ) ) ;
#10292=DIRECTION ( 'NONE',  ( -1.000000000000000000, 0.000000000000000000, 0.000000000000000000 ) ) ;
#10295=CARTESIAN_POINT ( 'NONE',  ( 1.346194077712560944, 6.937500000000000000, -0.2500000000000010547 ) ) ;
#10300=CARTESIAN_POINT ( 'NONE',  ( 0.000000000000000000, 3.000000000000000000, 0.2500000000000002220 ) ) ;
#10301=CARTESIAN_POINT ( 'NONE',  ( 2.298097038856278029, 14.12500000000000000, -5.798097038856279362 ) ) ;
#10305=CARTESIAN_POINT ( 'NONE',  ( -3.249999999999999556, 9.312499999999998224, -4.846194077712557835 ) ) ;
#10314=CARTESIAN_POINT ( 'NONE',  ( -1.346194077712558945, 11.06250000000000000, -0.2500000000000002220 ) ) ;
#10317=CARTESIAN_POINT ( 'NONE',  ( -3.249999999999999556, 4.250000000000000000, -3.499999999999999556 ) ) ;
#10319=CARTESIAN_POINT ( 'NONE',  ( -1.553300858899106629, 2.562500000000000444, 0.2500000000000002220 ) ) ;
#10320=CARTESIAN_POINT ( 'NONE',  ( 1.346194077712558279, 6.062500000000000888, -6.750000000000000888 ) ) ;
#10324=CARTESIAN_POINT ( 'NONE',  ( 2.651650429449553759, 4.875000000000000000, -0.8483495705504471296 ) ) ;
#10332=CARTESIAN_POINT ( 'NONE',  ( 2.298097038856279362, 6.374999999999999112, -1.201902961143720860 ) ) ;
#10334=CARTESIAN_POINT ( 'NONE',  ( -3.749999999999999556, 9.750000000000000000, -3.499999999999999112 ) ) ;
#10336=ORIENTED_EDGE ( 'NONE', *, *, #4932, .F. ) ;
#10338=CARTESIAN_POINT ( 'NONE',  ( -1.553300858899106629, 12.56250000000000355, 0.2500000000000002220 ) ) ;
#10350=CARTESIAN_POINT ( 'NONE',  ( -2.298097038856279362, 1.874999999999999778, -5.798097038856278473 ) ) ;
#10354=CARTESIAN_POINT ( 'NONE',  ( 1.346194077712558057, 10.56250000000000000, -6.750000000000000000 ) ) ;
#10358=CARTESIAN_POINT ( 'NONE',  ( 2.298097038856278029, 12.12500000000000000, -5.798097038856279362 ) ) ;
#10362=CARTESIAN_POINT ( 'NONE',  ( 0.000000000000000000, 1.500000000000000222, 0.2500000000000002220 ) ) ;
#10371=CARTESIAN_POINT ( 'NONE',  ( -3.249999999999999556, 7.250000000000000000, -3.499999999999999556 ) ) ;
#10374=CARTESIAN_POINT ( 'NONE',  ( -0.3766621274091715987, 0.5000000000000000000, -0.1347136637304948981 ) ) ;
#10378=CARTESIAN_POINT ( 'NONE',  ( -3.749999999999999556, 2.312500000000000888, -5.053300858899104853 ) ) ;
#10379=CARTESIAN_POINT ( 'NONE',  ( -3.749999999999999556, 0.7499999999999998890, -3.499999999999999112 ) ) ;
#10382=CARTESIAN_POINT ( 'NONE',  ( -2.298097038856278918, 7.375000000000000888, -5.798097038856277585 ) ) ;
#10383=CARTESIAN_POINT ( 'NONE',  ( -3.249999999999999556, 1.750000000000000000, -3.500000000000000000 ) ) ;
#10391=CARTESIAN_POINT ( 'NONE',  ( -3.249999999999999556, 4.187500000000000000, -2.153805922287440833 ) ) ;
#10397=CARTESIAN_POINT ( 'NONE',  ( 1.346194077712558279, 9.562500000000000000, -6.750000000000000000 ) ) ;
#10402=CARTESIAN_POINT ( 'NONE',  ( -4.592425496802573972E-16, 11.00000000000000000, -7.250000000000000000 ) ) ;
#10405=CARTESIAN_POINT ( 'NONE',  ( 1.553300858899109516, 1.437500000000000000, 0.2499999999999993616 ) ) ;
#10406=CARTESIAN_POINT ( 'NONE',  ( 2.298097038856278029, 7.125000000000000888, -5.798097038856279362 ) ) ;
#10409=CARTESIAN_POINT ( 'NONE',  ( 0.000000000000000000, 2.000000000000000000, -0.2500000000000002220 ) ) ;
#10410=CARTESIAN_POINT ( 'NONE',  ( -3.749999999999999556, 7.187500000000000000, -1.946699141100892927 ) ) ;
#10416=CARTESIAN_POINT ( 'NONE',  ( 3.249999999999998224, 9.187500000000001776, -4.846194077712561388 ) ) ;
#10419=CARTESIAN_POINT ( 'NONE',  ( 2.651650429449552870, 9.125000000000001776, -6.151650429449553314 ) ) ;
#10420=CARTESIAN_POINT ( 'NONE',  ( 1.553300858899105963, 13.56250000000000000, -7.250000000000000000 ) ) ;
#10423=CARTESIAN_POINT ( 'NONE',  ( -4.592425496802573972E-16, 14.00000000000000000, -7.250000000000000000 ) ) ;
#10430=CARTESIAN_POINT ( 'NONE',  ( 0.000000000000000000, 3.000000000000000000, -0.2500000000000002220 ) ) ;
#10433=CARTESIAN_POINT ( 'NONE',  ( -3.249999999999999112, 2.812500000000000444, -4.846194077712558723 ) ) ;
#10440=CARTESIAN_POINT ( 'NONE',  ( 0.000000000000000000, 12.50000000000000178, -0.2500000000000002220 ) ) ;
#10442=CARTESIAN_POINT ( 'NONE',  ( -3.750000000000000000, 0.8125000000000001110, -5.053300858899105741 ) ) ;
#10448=CARTESIAN_POINT ( 'NONE',  ( 1.346194077712558057, 7.562500000000000000, -6.750000000000000000 ) ) ;
#10454=CARTESIAN_POINT ( 'NONE',  ( -1.553300858899106629, 4.062500000000000000, 0.2500000000000002220 ) ) ;
#10456=CARTESIAN_POINT ( 'NONE',  ( 1.553300858899105963, 2.062500000000000000, -7.249999999999999112 ) ) ;
#10460=CARTESIAN_POINT ( 'NONE',  ( 0.000000000000000000, 14.00000000000000000, -0.2500000000000002220 ) ) ;
#10463=CARTESIAN_POINT ( 'NONE',  ( -1.346194077712559389, 11.43750000000000000, -6.749999999999999112 ) ) ;
#10467=CARTESIAN_POINT ( 'NONE',  ( 0.000000000000000000, 4.000000000000000000, -0.2500000000000002220 ) ) ;
#10475=CARTESIAN_POINT ( 'NONE',  ( 0.000000000000000000, 13.00000000000000178, -0.2500000000000002220 ) ) ;
#10478=CARTESIAN_POINT ( 'NONE',  ( -1.553300858899106629, 8.562500000000000000, 0.2500000000000002220 ) ) ;
#10480=CARTESIAN_POINT ( 'NONE',  ( 3.750000000000000000, 7.312500000000001776, -1.946699141100892705 ) ) ;
#10481=CARTESIAN_POINT ( 'NONE',  ( -1.346194077712559167, 7.937500000000001776, -6.749999999999999112 ) ) ;
#10485=CARTESIAN_POINT ( 'NONE',  ( 3.249999999999999112, 1.812500000000000222, -2.153805922287439945 ) ) ;
#10488=CARTESIAN_POINT ( 'NONE',  ( -3.749999999999999556, 4.187500000000000000, -1.946699141100892927 ) ) ;
#10493=DIRECTION ( 'NONE',  ( -0.000000000000000000, -1.000000000000000000, -0.000000000000000000 ) ) ;
#10496=CARTESIAN_POINT ( 'NONE',  ( -3.249999999999999556, 5.750000000000000000, -3.500000000000000000 ) ) ;
#10498=CARTESIAN_POINT ( 'NONE',  ( -2.651650429449552870, 10.87500000000000000, -6.151650429449552426 ) ) ;
#10499=CARTESIAN_POINT ( 'NONE',  ( -3.750000000000000000, 13.18750000000000000, -1.946699141100892927 ) ) ;
#10502=CARTESIAN_POINT ( 'NONE',  ( 3.750000000000000000, 14.31250000000000355, -1.946699141100892705 ) ) ;
#10508=CARTESIAN_POINT ( 'NONE',  ( -3.980102097228897245E-16, 2.500000000000000000, -6.749999999999999112 ) ) ;
#10510=CARTESIAN_POINT ( 'NONE',  ( 3.249999999999998224, 1.312500000000000444, -2.153805922287439945 ) ) ;
#10515=FACE_BOUND ( 'NONE', #13098, .T. ) ;
#10516=CARTESIAN_POINT ( 'NONE',  ( -3.249999999999999556, 10.75000000000000178, -3.500000000000000000 ) ) ;
#10518=CARTESIAN_POINT ( 'NONE',  ( 3.750000000000000000, 0.3125000000000002220, -1.946699141100892705 ) ) ;
#10523=EDGE_CURVE ( 'NONE', #11692, #5961, #5124, .T. ) ;
#10525=CARTESIAN_POINT ( 'NONE',  ( 1.346194077712558057, 13.56250000000000000, -6.750000000000000000 ) ) ;
#10531=CARTESIAN_POINT ( 'NONE',  ( 2.651650429449552870, 3.625000000000000000, -6.151650429449554203 ) ) ;
#10532=CARTESIAN_POINT ( 'NONE',  ( 3.749999999999999556, 5.249999999999999112, -3.500000000000000444 ) ) ;
#10535=CARTESIAN_POINT ( 'NONE',  ( 1.346194077712558057, 13.56250000000000000, -6.750000000000000000 ) ) ;
#10538=CARTESIAN_POINT ( 'NONE',  ( 3.249999999999999556, 5.750000000000000000, -3.500000000000000000 ) ) ;
#10545=PLANE ( 'NONE',  #7909 ) ;
#10546=CARTESIAN_POINT ( 'NONE',  ( 1.346194077712558279, 10.56250000000000000, -6.750000000000000000 ) ) ;
#10549=DIRECTION ( 'NONE',  ( -1.000000000000000000, -0.000000000000000000, -0.000000000000000000 ) ) ;
#10550=CARTESIAN_POINT ( 'NONE',  ( 3.749999999999999556, 4.250000000000000000, -3.500000000000000444 ) ) ;
#10551=CARTESIAN_POINT ( 'NONE',  ( -1.346194077712559167, 6.937500000000001776, -6.749999999999999112 ) ) ;
#10552=ORIENTED_EDGE ( 'NONE', *, *, #7140, .F. ) ;
#10554=CARTESIAN_POINT ( 'NONE',  ( -3.249999999999999556, 4.250000000000000000, -3.499999999999999556 ) ) ;
#10555=CARTESIAN_POINT ( 'NONE',  ( -3.749999999999999556, 10.18750000000000000, -1.946699141100892927 ) ) ;
#10558=CARTESIAN_POINT ( 'NONE',  ( 0.3766621274091715987, 0.5000000000000000000, 0.1491815183709511716 ) ) ;
#10561=EDGE_CURVE ( 'NONE', #5120, #13895, #11936, .T. ) ;
#10563=CARTESIAN_POINT ( 'NONE',  ( 2.298097038856279362, 8.375000000000000000, -1.201902961143720860 ) ) ;
#10564=CARTESIAN_POINT ( 'NONE',  ( -2.651650429449552870, 7.625000000000000000, -0.8483495705504467965 ) ) ;
#10568=CARTESIAN_POINT ( 'NONE',  ( 2.651650429449552870, 14.12500000000000000, -6.151650429449555091 ) ) ;
#10575=CARTESIAN_POINT ( 'NONE',  ( 0.000000000000000000, 5.000000000000000000, -0.2500000000000002220 ) ) ;
#10577=CARTESIAN_POINT ( 'NONE',  ( -1.346194077712558945, 6.562500000000000888, -0.2500000000000002220 ) ) ;
#10582=CARTESIAN_POINT ( 'NONE',  ( 3.249999999999998668, 1.687500000000000000, -4.846194077712560500 ) ) ;
#10583=CARTESIAN_POINT ( 'NONE',  ( -3.249999999999999556, 12.75000000000000178, -3.500000000000000000 ) ) ;
#10585=CARTESIAN_POINT ( 'NONE',  ( -4.592425496802573972E-16, 3.000000000000000444, -7.250000000000000000 ) ) ;
#10590=CARTESIAN_POINT ( 'NONE',  ( -3.980102097228897245E-16, 12.50000000000000000, -6.749999999999999112 ) ) ;
#10595=ORIENTED_EDGE ( 'NONE', *, *, #9967, .T. ) ;
#10598=CARTESIAN_POINT ( 'NONE',  ( 2.651650429449552870, 6.625000000000000000, -6.151650429449554203 ) ) ;
#10599=CARTESIAN_POINT ( 'NONE',  ( 3.749999999999999112, 4.312500000000000000, -1.946699141100893149 ) ) ;
#10603=CARTESIAN_POINT ( 'NONE',  ( 1.346194077712561166, 2.437500000000000444, -0.2500000000000011102 ) ) ;
#10607=CARTESIAN_POINT ( 'NONE',  ( 2.298097038856278473, 2.625000000000000000, -5.798097038856279362 ) ) ;
#10615=CARTESIAN_POINT ( 'NONE',  ( 2.298097038856278473, 13.62500000000000000, -5.798097038856279362 ) ) ;
#10619=CARTESIAN_POINT ( 'NONE',  ( 0.000000000000000000, 5.500000000000000888, 0.2500000000000002220 ) ) ;
#10620=CARTESIAN_POINT ( 'NONE',  ( 2.298097038856279362, 7.375000000000000000, -1.201902961143720860 ) ) ;
#10624=CARTESIAN_POINT ( 'NONE',  ( 3.249999999999999112, 2.812500000000000000, -2.153805922287439945 ) ) ;
#10640=EDGE_CURVE ( 'NONE', #2112, #1425, #1461, .T. ) ;
#10641=CARTESIAN_POINT ( 'NONE',  ( 2.651650429449552870, 13.12500000000000178, -6.151650429449553314 ) ) ;
#10647=CARTESIAN_POINT ( 'NONE',  ( 2.298097038856278029, 3.125000000000000444, -5.798097038856279362 ) ) ;
#10656=CARTESIAN_POINT ( 'NONE',  ( -1.346194077712559167, 1.437500000000000000, -6.749999999999999112 ) ) ;
#10658=CARTESIAN_POINT ( 'NONE',  ( -1.346194077712559167, 6.937500000000001776, -6.749999999999999112 ) ) ;
#10664=CARTESIAN_POINT ( 'NONE',  ( 3.249999999999998224, 15.31250000000000355, -2.153805922287439945 ) ) ;
#10665=CARTESIAN_POINT ( 'NONE',  ( 1.553300858899105963, 4.562500000000001776, -7.250000000000000000 ) ) ;
#10667=CARTESIAN_POINT ( 'NONE',  ( 0.1262058122322286813, 0.3029806520654600432, -7.146945437571384119 ) ) ;
#10668=CARTESIAN_POINT ( 'NONE',  ( -3.749999999999999556, 3.750000000000000444, -3.499999999999999112 ) ) ;
#10673=CARTESIAN_POINT ( 'NONE',  ( -3.249999999999999556, 13.25000000000000000, -3.499999999999999556 ) ) ;
#10676=ORIENTED_EDGE ( 'NONE', *, *, #5371, .T. ) ;
#10680=CARTESIAN_POINT ( 'NONE',  ( 3.749999999999998668, 6.687500000000000888, -5.053300858899107517 ) ) ;
#10681=CARTESIAN_POINT ( 'NONE',  ( -4.592425496802573972E-16, 3.000000000000000444, -7.250000000000000000 ) ) ;
#10685=CARTESIAN_POINT ( 'NONE',  ( -3.249999999999999112, 3.812500000000000000, -4.846194077712558723 ) ) ;
#10688=CARTESIAN_POINT ( 'NONE',  ( 0.000000000000000000, 6.000000000000000000, -0.2500000000000002220 ) ) ;
#10697=CARTESIAN_POINT ( 'NONE',  ( 1.346194077712558279, 14.56250000000000000, -6.750000000000000000 ) ) ;
#10701=CARTESIAN_POINT ( 'NONE',  ( 1.553300858899109516, 4.437500000000001776, 0.2499999999999993616 ) ) ;
#10702=CARTESIAN_POINT ( 'NONE',  ( -3.249999999999999112, 10.81250000000000000, -4.846194077712558723 ) ) ;
#10705=CARTESIAN_POINT ( 'NONE',  ( -2.298097038856278918, 2.375000000000000000, -5.798097038856277585 ) ) ;
#10706=AXIS2_PLACEMENT_3D ( 'NONE', #9729, #612, #14460 ) ;
#10718=CARTESIAN_POINT ( 'NONE',  ( 3.749999999999998668, 12.18750000000000178, -5.053300858899108405 ) ) ;
#10722=CARTESIAN_POINT ( 'NONE',  ( -1.346194077712558945, 1.562500000000000222, -0.2500000000000002220 ) ) ;
#10731=CARTESIAN_POINT ( 'NONE',  ( -1.346194077712558945, 3.062500000000000000, -0.2500000000000002220 ) ) ;
#10732=EDGE_CURVE ( 'NONE', #5680, #1124, #5463, .T. ) ;
#10734=CARTESIAN_POINT ( 'NONE',  ( 1.346194077712558279, 5.062500000000000000, -6.750000000000000888 ) ) ;
#10739=CARTESIAN_POINT ( 'NONE',  ( -3.980102097228897245E-16, 2.500000000000000000, -6.749999999999999112 ) ) ;
#10740=CARTESIAN_POINT ( 'NONE',  ( -4.592425496802573972E-16, 3.000000000000000444, -7.250000000000000000 ) ) ;
#10741=CARTESIAN_POINT ( 'NONE',  ( 0.000000000000000000, 4.000000000000000000, 0.2500000000000002220 ) ) ;
#10743=CARTESIAN_POINT ( 'NONE',  ( 3.749999999999999112, 6.187500000000001776, -5.053300858899108405 ) ) ;
#10748=CARTESIAN_POINT ( 'NONE',  ( 3.249999999999999112, 12.81250000000000000, -2.153805922287439945 ) ) ;
#10753=CARTESIAN_POINT ( 'NONE',  ( 3.749999999999999112, 9.187500000000001776, -5.053300858899108405 ) ) ;
#10757=CARTESIAN_POINT ( 'NONE',  ( 2.651650429449553759, 4.875000000000000000, -0.8483495705504471296 ) ) ;
#10758=CARTESIAN_POINT ( 'NONE',  ( 0.000000000000000000, 5.500000000000000000, 0.2499999999999998057 ) ) ;
#10761=CARTESIAN_POINT ( 'NONE',  ( 1.346194077712561166, 6.437499999999999112, -0.2500000000000011102 ) ) ;
#10766=CARTESIAN_POINT ( 'NONE',  ( 3.249999999999999556, 6.750000000000000000, -3.500000000000000000 ) ) ;
#10771=DIRECTION ( 'NONE',  ( -0.000000000000000000, -1.000000000000000000, -0.000000000000000000 ) ) ;
#10776=CARTESIAN_POINT ( 'NONE',  ( -3.750000000000000000, 6.812500000000001776, -5.053300858899105741 ) ) ;
#10777=CARTESIAN_POINT ( 'NONE',  ( -3.980102097228897738E-16, 11.00000000000000000, -6.749999999999999112 ) ) ;
#10780=CARTESIAN_POINT ( 'NONE',  ( 3.249999999999998668, 5.687500000000000000, -4.846194077712560500 ) ) ;
#10788=CARTESIAN_POINT ( 'NONE',  ( 3.249999999999998224, 14.31250000000000355, -2.153805922287439945 ) ) ;
#10791=CARTESIAN_POINT ( 'NONE',  ( 3.749999999999999556, 12.25000000000000000, -3.500000000000000444 ) ) ;
#10795=CARTESIAN_POINT ( 'NONE',  ( -3.980102097228897738E-16, 2.000000000000000000, -6.749999999999999112 ) ) ;
#10802=CARTESIAN_POINT ( 'NONE',  ( -3.249999999999999556, 5.312500000000000888, -4.846194077712557835 ) ) ;
#10804=CARTESIAN_POINT ( 'NONE',  ( -1.346194077712559167, 0.9375000000000000000, -6.749999999999999112 ) ) ;
#10805=CARTESIAN_POINT ( 'NONE',  ( 1.346194077712558279, 7.062500000000000888, -6.750000000000000888 ) ) ;
#10807=CARTESIAN_POINT ( 'NONE',  ( -0.1255007366002022229, -0.2049726491322196309, -0.1347136637248375068 ) ) ;
#10809=CARTESIAN_POINT ( 'NONE',  ( -3.980102097228897245E-16, 1.500000000000000000, -6.749999999999999112 ) ) ;
#10810=CARTESIAN_POINT ( 'NONE',  ( -1.553300858899106629, 2.562500000000000444, 0.2499999999999998335 ) ) ;
#10811=CARTESIAN_POINT ( 'NONE',  ( -3.750000000000000000, 4.250000000000000000, -3.499999999999999112 ) ) ;
#10813=CARTESIAN_POINT ( 'NONE',  ( 3.749999999999999112, 5.187500000000001776, -5.053300858899108405 ) ) ;
#10822=CARTESIAN_POINT ( 'NONE',  ( 2.298097038856279362, 8.875000000000001776, -1.201902961143720860 ) ) ;
#10824=CARTESIAN_POINT ( 'NONE',  ( -3.750000000000000000, 9.812500000000000000, -5.053300858899105741 ) ) ;
#10828=CARTESIAN_POINT ( 'NONE',  ( -3.750000000000000000, 9.250000000000000000, -3.499999999999999112 ) ) ;
#10829=CARTESIAN_POINT ( 'NONE',  ( -4.592425496802573972E-16, 5.000000000000000000, -7.250000000000000000 ) ) ;
#10832=CARTESIAN_POINT ( 'NONE',  ( 1.346194077712558279, 3.062500000000000000, -6.750000000000000888 ) ) ;
#10834=CARTESIAN_POINT ( 'NONE',  ( 3.750000000000000000, 9.750000000000000000, -3.500000000000000444 ) ) ;
#10839=CARTESIAN_POINT ( 'NONE',  ( 1.346194077712558057, 7.562500000000000000, -6.750000000000000000 ) ) ;
#10846=PLANE ( 'NONE',  #1747 ) ;
#10851=CARTESIAN_POINT ( 'NONE',  ( 2.651650429449552870, 12.12500000000000000, -6.151650429449553314 ) ) ;
#10852=CARTESIAN_POINT ( 'NONE',  ( -2.298097038856278029, 6.625000000000000000, -1.201902961143720638 ) ) ;
#10853=CARTESIAN_POINT ( 'NONE',  ( 3.249999999999999556, 10.25000000000000178, -3.500000000000000000 ) ) ;
#10856=CARTESIAN_POINT ( 'NONE',  ( -3.249999999999999556, 7.187500000000000000, -2.153805922287440833 ) ) ;
#10867=CARTESIAN_POINT ( 'NONE',  ( -3.249999999999999556, 2.312500000000000888, -4.846194077712557835 ) ) ;
#10868=CARTESIAN_POINT ( 'NONE',  ( -1.553300858899107295, 14.43750000000000000, -7.250000000000000000 ) ) ;
#10871=CARTESIAN_POINT ( 'NONE',  ( -2.651650429449552870, 12.87500000000000178, -6.151650429449552426 ) ) ;
#10875=CARTESIAN_POINT ( 'NONE',  ( -2.298097038856278029, 3.625000000000000888, -1.201902961143720638 ) ) ;
#10883=CARTESIAN_POINT ( 'NONE',  ( -2.298097038856278918, 6.375000000000000888, -5.798097038856277585 ) ) ;
#10887=CARTESIAN_POINT ( 'NONE',  ( 3.249999999999998224, 1.187499999999999778, -4.846194077712561388 ) ) ;
#10889=CARTESIAN_POINT ( 'NONE',  ( 3.249999999999998224, 11.18750000000000178, -4.846194077712561388 ) ) ;
#10894=CARTESIAN_POINT ( 'NONE',  ( -3.249999999999999556, 6.312500000000000888, -4.846194077712557835 ) ) ;
#10895=CARTESIAN_POINT ( 'NONE',  ( 2.298097038856279362, 15.37500000000000178, -1.201902961143720860 ) ) ;
#10896=CARTESIAN_POINT ( 'NONE',  ( 3.749999999999999556, 5.812500000000000000, -1.946699141100892261 ) ) ;
#10898=CARTESIAN_POINT ( 'NONE',  ( 2.651650429449552870, 5.125000000000000888, -6.151650429449555091 ) ) ;
#10903=CARTESIAN_POINT ( 'NONE',  ( -0.3766621274091715987, 0.2613176957160640579, -6.863050255469941519 ) ) ;
#10908=CARTESIAN_POINT ( 'NONE',  ( -2.651650429449553314, 8.874999999999996447, -6.151650429449552426 ) ) ;
#10912=CARTESIAN_POINT ( 'NONE',  ( 1.553300858899105963, 9.562500000000000000, -7.250000000000000888 ) ) ;
#10913=CARTESIAN_POINT ( 'NONE',  ( 1.553300858899109071, 8.437500000000000000, 0.2499999999999989175 ) ) ;
#10918=CARTESIAN_POINT ( 'NONE',  ( -3.980102097228897738E-16, 5.000000000000000000, -6.749999999999999112 ) ) ;
#10919=CARTESIAN_POINT ( 'NONE',  ( -2.651650429449553314, 10.37500000000000000, -6.151650429449552426 ) ) ;
#10923=CARTESIAN_POINT ( 'NONE',  ( 3.249999999999998668, 6.687500000000000888, -4.846194077712560500 ) ) ;
#10930=CARTESIAN_POINT ( 'NONE',  ( -1.346194077712558945, 13.06250000000000000, -0.2500000000000002220 ) ) ;
#10932=ADVANCED_FACE ( 'NONE', ( #6624 ), #6558, .F. ) ;
#10935=CARTESIAN_POINT ( 'NONE',  ( 3.749999999999998668, 12.18750000000000178, -5.053300858899108405 ) ) ;
#10936=CARTESIAN_POINT ( 'NONE',  ( -3.249999999999999112, 12.81250000000000178, -4.846194077712558723 ) ) ;
#10938=CARTESIAN_POINT ( 'NONE',  ( 3.249999999999999556, 11.25000000000000000, -3.500000000000000000 ) ) ;
#10942=CARTESIAN_POINT ( 'NONE',  ( -1.346194077712559389, 5.437500000000002665, -6.749999999999999112 ) ) ;
#10950=CARTESIAN_POINT ( 'NONE',  ( 3.249999999999999556, 9.750000000000000000, -3.500000000000000000 ) ) ;
#10951=CARTESIAN_POINT ( 'NONE',  ( 1.346194077712558057, 2.562500000000000444, -6.750000000000000000 ) ) ;
#10952=CARTESIAN_POINT ( 'NONE',  ( 3.750000000000000000, 14.75000000000000178, -3.500000000000000444 ) ) ;
#10957=CARTESIAN_POINT ( 'NONE',  ( -1.553300858899106629, 0.06250000000000002776, 0.2500000000000002220 ) ) ;
#10967=CARTESIAN_POINT ( 'NONE',  ( 1.346194077712560944, 6.937500000000000000, -0.2500000000000011102 ) ) ;
#10969=CARTESIAN_POINT ( 'NONE',  ( 1.346194077712560944, 11.93750000000000000, -0.2500000000000010547 ) ) ;
#10970=CARTESIAN_POINT ( 'NONE',  ( -3.980102097228897738E-16, 12.00000000000000178, -6.749999999999999112 ) ) ;
#10972=CARTESIAN_POINT ( 'NONE',  ( -3.249999999999999556, 0.2500000000000000000, -3.499999999999999556 ) ) ;
#10974=CARTESIAN_POINT ( 'NONE',  ( -2.298097038856278918, 4.375000000000000000, -5.798097038856277585 ) ) ;
#10976=CARTESIAN_POINT ( 'NONE',  ( -3.249999999999999112, 14.68750000000000178, -2.153805922287440833 ) ) ;
#10977=CARTESIAN_POINT ( 'NONE',  ( -1.553300858899106407, 4.062500000000000000, 0.2500000000000002220 ) ) ;
#10979=CARTESIAN_POINT ( 'NONE',  ( 3.749999999999999112, 7.187500000000000888, -5.053300858899108405 ) ) ;
#10988=CARTESIAN_POINT ( 'NONE',  ( -3.249999999999999112, -0.1874999999999998890, -4.846194077712558723 ) ) ;
#10992=CARTESIAN_POINT ( 'NONE',  ( 3.749999999999998668, 10.68750000000000000, -5.053300858899107517 ) ) ;
#10993=CARTESIAN_POINT ( 'NONE',  ( 2.651650429449552870, 7.124999999999999112, -6.151650429449553314 ) ) ;
#10996=CARTESIAN_POINT ( 'NONE',  ( 1.346194077712558279, 4.062500000000001776, -6.750000000000000888 ) ) ;
#10999=CARTESIAN_POINT ( 'NONE',  ( 1.553300858899108849, 9.937499999999998224, 0.2499999999999993616 ) ) ;
#11004=CARTESIAN_POINT ( 'NONE',  ( -1.346194077712559389, 7.062500000000000000, -0.2500000000000002220 ) ) ;
#11015=CARTESIAN_POINT ( 'NONE',  ( -4.592425496802573972E-16, 12.00000000000000178, -7.250000000000000000 ) ) ;
#11016=CARTESIAN_POINT ( 'NONE',  ( 1.346194077712561166, 9.437500000000003553, -0.2500000000000011102 ) ) ;
#11017=CARTESIAN_POINT ( 'NONE',  ( 3.249999999999999556, 12.25000000000000000, -3.500000000000000000 ) ) ;
#11020=CARTESIAN_POINT ( 'NONE',  ( 3.249999999999999112, 6.812500000000000000, -2.153805922287439945 ) ) ;
#11025=ADVANCED_FACE ( 'NONE', ( #7317 ), #874, .F. ) ;
#11029=CARTESIAN_POINT ( 'NONE',  ( 3.249999999999999112, 1.812500000000000222, -2.153805922287439945 ) ) ;
#11030=CARTESIAN_POINT ( 'NONE',  ( -3.749999999999999556, 14.18750000000000000, -1.946699141100892927 ) ) ;
#11033=CARTESIAN_POINT ( 'NONE',  ( 2.651650429449553759, 2.875000000000000000, -0.8483495705504471296 ) ) ;
#11037=CARTESIAN_POINT ( 'NONE',  ( -3.750000000000000000, 2.187500000000000444, -1.946699141100892927 ) ) ;
#11041=CARTESIAN_POINT ( 'NONE',  ( -0.3766621274091715987, -0.2500000000000000000, -0.1347136637304948981 ) ) ;
#11043=CARTESIAN_POINT ( 'NONE',  ( -2.298097038856278473, 8.125000000000000000, -1.201902961143720416 ) ) ;
#11045=CARTESIAN_POINT ( 'NONE',  ( 1.346194077712558057, 13.56250000000000000, -6.750000000000000000 ) ) ;
#11046=CARTESIAN_POINT ( 'NONE',  ( -2.298097038856279362, 9.875000000000000000, -5.798097038856278473 ) ) ;
#11050=CARTESIAN_POINT ( 'NONE',  ( 2.298097038856278473, 3.625000000000000000, -5.798097038856279362 ) ) ;
#11051=CARTESIAN_POINT ( 'NONE',  ( 3.749999999999998668, 7.187500000000000888, -5.053300858899108405 ) ) ;
#11052=CARTESIAN_POINT ( 'NONE',  ( -2.651650429449553314, 8.375000000000000000, -6.151650429449552426 ) ) ;
#11054=CARTESIAN_POINT ( 'NONE',  ( 1.553300858899105963, 7.062500000000000888, -7.250000000000000888 ) ) ;
#11062=CARTESIAN_POINT ( 'NONE',  ( -1.346194077712559167, -0.06249999999999988898, -6.749999999999999112 ) ) ;
#11066=CARTESIAN_POINT ( 'NONE',  ( 0.000000000000000000, 9.000000000000001776, 0.2500000000000002220 ) ) ;
#11067=CARTESIAN_POINT ( 'NONE',  ( 0.000000000000000000, 9.500000000000001776, 0.2499999999999998057 ) ) ;
#11070=CARTESIAN_POINT ( 'NONE',  ( 3.249999999999998224, 8.312500000000003553, -2.153805922287439945 ) ) ;
#11071=CARTESIAN_POINT ( 'NONE',  ( -4.592425496802573972E-16, 10.50000000000000000, -7.249999999999999112 ) ) ;
#11074=CARTESIAN_POINT ( 'NONE',  ( 3.249999999999999112, 7.812500000000000000, -2.153805922287439945 ) ) ;
#11076=CARTESIAN_POINT ( 'NONE',  ( 0.000000000000000000, -0.2006112523677016091, 0.1491815183709511716 ) ) ;
#11082=CARTESIAN_POINT ( 'NONE',  ( 0.3766621274091715987, 0.2956834184403337451, -6.863050255469942407 ) ) ;
#11083=CARTESIAN_POINT ( 'NONE',  ( -1.553300858899107073, 11.93750000000000178, -7.249999999999999112 ) ) ;
#11084=CARTESIAN_POINT ( 'NONE',  ( 1.346194077712558279, 10.06250000000000000, -6.750000000000000888 ) ) ;
#11086=CARTESIAN_POINT ( 'NONE',  ( -1.346194077712559389, 1.437500000000000000, -6.749999999999999112 ) ) ;
#11088=CARTESIAN_POINT ( 'NONE',  ( -2.298097038856278918, 7.375000000000000888, -5.798097038856277585 ) ) ;
#11096=CARTESIAN_POINT ( 'NONE',  ( -3.249999999999999112, 13.81250000000000178, -4.846194077712558723 ) ) ;
#11097=CARTESIAN_POINT ( 'NONE',  ( -3.749999999999999556, 12.31250000000000000, -5.053300858899104853 ) ) ;
#11102=CARTESIAN_POINT ( 'NONE',  ( 2.651650429449553759, 0.8750000000000000000, -0.8483495705504471296 ) ) ;
#11105=CARTESIAN_POINT ( 'NONE',  ( -1.553300858899107073, 2.437500000000000444, -7.250000000000000000 ) ) ;
#11112=CARTESIAN_POINT ( 'NONE',  ( 0.000000000000000000, 8.000000000000000000, -0.2500000000000002220 ) ) ;
#11114=CARTESIAN_POINT ( 'NONE',  ( 3.249999999999998224, 2.187500000000000000, -4.846194077712561388 ) ) ;
#11116=CARTESIAN_POINT ( 'NONE',  ( 3.249999999999999556, 11.25000000000000000, -3.500000000000000000 ) ) ;
#11122=CARTESIAN_POINT ( 'NONE',  ( 3.249999999999999556, 6.750000000000000000, -3.500000000000000000 ) ) ;
#11124=CARTESIAN_POINT ( 'NONE',  ( 2.651650429449553314, 6.374999999999999112, -0.8483495705504476847 ) ) ;
#11127=CARTESIAN_POINT ( 'NONE',  ( 3.749999999999999112, 10.68750000000000000, -5.053300858899108405 ) ) ;
#11130=CARTESIAN_POINT ( 'NONE',  ( 1.553300858899109516, 10.43750000000000178, 0.2499999999999993616 ) ) ;
#11139=CARTESIAN_POINT ( 'NONE',  ( -3.750000000000000000, 13.81250000000000178, -5.053300858899105741 ) ) ;
#11143=CARTESIAN_POINT ( 'NONE',  ( -2.651650429449553314, 11.37500000000000000, -6.151650429449552426 ) ) ;
#11144=CARTESIAN_POINT ( 'NONE',  ( 1.553300858899109071, 6.437499999999999112, 0.2499999999999989175 ) ) ;
#11148=CARTESIAN_POINT ( 'NONE',  ( 0.000000000000000000, 7.499999999999999112, -0.2500000000000002220 ) ) ;
#11149=CARTESIAN_POINT ( 'NONE',  ( -4.592425496802573972E-16, 1.084202172485504434E-16, -7.250000000000000000 ) ) ;
#11153=CARTESIAN_POINT ( 'NONE',  ( -2.298097038856278473, 10.12500000000000000, -1.201902961143720416 ) ) ;
#11162=CARTESIAN_POINT ( 'NONE',  ( 1.553300858899105963, 14.06250000000000178, -7.249999999999999112 ) ) ;
#11163=CARTESIAN_POINT ( 'NONE',  ( -2.298097038856278029, 9.624999999999998224, -1.201902961143720638 ) ) ;
#11164=CARTESIAN_POINT ( 'NONE',  ( 0.000000000000000000, 14.50000000000000000, -0.2500000000000002220 ) ) ;
#11166=CARTESIAN_POINT ( 'NONE',  ( 2.298097038856279362, 12.87500000000000178, -1.201902961143720860 ) ) ;
#11175=VERTEX_POINT ( 'NONE', #6395 ) ;
#11176=CARTESIAN_POINT ( 'NONE',  ( -1.346194077712559389, 4.437500000000000888, -6.749999999999999112 ) ) ;
#11177=CARTESIAN_POINT ( 'NONE',  ( -4.592425496802573972E-16, 11.50000000000000000, -7.249999999999999112 ) ) ;
#11180=CARTESIAN_POINT ( 'NONE',  ( 3.750000000000000000, 2.750000000000000000, -3.500000000000000444 ) ) ;
#11184=CARTESIAN_POINT ( 'NONE',  ( -3.750000000000000000, 0.1875000000000000555, -1.946699141100892927 ) ) ;
#11187=PLANE ( 'NONE',  #10706 ) ;
#11188=CARTESIAN_POINT ( 'NONE',  ( -3.249999999999999556, 11.25000000000000000, -3.499999999999999556 ) ) ;
#11189=DIRECTION ( 'NONE',  ( -0.000000000000000000, -0.000000000000000000, 1.000000000000000000 ) ) ;
#11191=CARTESIAN_POINT ( 'NONE',  ( -3.980102097228897245E-16, 9.500000000000000000, -6.749999999999999112 ) ) ;
#11195=CARTESIAN_POINT ( 'NONE',  ( -3.249999999999999112, 4.687500000000000000, -2.153805922287440833 ) ) ;
#11196=CARTESIAN_POINT ( 'NONE',  ( 1.346194077712558279, 10.06250000000000000, -6.750000000000000888 ) ) ;
#11200=CARTESIAN_POINT ( 'NONE',  ( 2.298097038856278473, 4.625000000000000000, -5.798097038856279362 ) ) ;
#11201=CARTESIAN_POINT ( 'NONE',  ( -4.592425496802573972E-16, 4.000000000000000000, -7.250000000000000000 ) ) ;
#11202=CARTESIAN_POINT ( 'NONE',  ( -1.553300858899106407, 9.062500000000000000, 0.2500000000000002220 ) ) ;
#11206=CARTESIAN_POINT ( 'NONE',  ( 2.651650429449554203, 8.375000000000000000, -0.8483495705504471296 ) ) ;
#11211=ADVANCED_FACE ( 'NONE', ( #6470 ), #11187, .T. ) ;
#11216=CARTESIAN_POINT ( 'NONE',  ( -2.651650429449553314, 11.87500000000000000, -6.151650429449552426 ) ) ;
#11221=CARTESIAN_POINT ( 'NONE',  ( -4.592425496802573972E-16, 7.000000000000000000, -7.250000000000000000 ) ) ;
#11222=DIRECTION ( 'NONE',  ( 0.000000000000000000, 0.000000000000000000, -1.000000000000000000 ) ) ;
#11224=CARTESIAN_POINT ( 'NONE',  ( 3.249999999999998224, 8.187500000000000000, -4.846194077712561388 ) ) ;
#11226=CARTESIAN_POINT ( 'NONE',  ( -1.553300858899107295, 12.43750000000000000, -7.250000000000000000 ) ) ;
#11229=CARTESIAN_POINT ( 'NONE',  ( -2.298097038856278918, 12.37500000000000000, -5.798097038856277585 ) ) ;
#11233=FACE_OUTER_BOUND ( 'NONE', #14679, .T. ) ;
#11236=DIRECTION ( 'NONE',  ( 0.000000000000000000, 0.000000000000000000, 1.000000000000000000 ) ) ;
#11240=CARTESIAN_POINT ( 'NONE',  ( 2.651650429449553759, 1.875000000000000000, -0.8483495705504471296 ) ) ;
#11241=CARTESIAN_POINT ( 'NONE',  ( -3.249999999999999556, 11.75000000000000178, -3.500000000000000000 ) ) ;
#11242=CARTESIAN_POINT ( 'NONE',  ( 3.249999999999998668, 0.6875000000000000000, -4.846194077712560500 ) ) ;
#11244=CARTESIAN_POINT ( 'NONE',  ( -1.346194077712559389, 10.06250000000000000, -0.2500000000000002220 ) ) ;
#11253=CARTESIAN_POINT ( 'NONE',  ( 2.298097038856278473, 4.625000000000000000, -5.798097038856279362 ) ) ;
#11255=CARTESIAN_POINT ( 'NONE',  ( -4.592425496802573972E-16, 1.084202172485504434E-16, -7.250000000000000000 ) ) ;
#11258=CARTESIAN_POINT ( 'NONE',  ( -3.750000000000000000, 3.250000000000000444, -3.499999999999999112 ) ) ;
#11261=CARTESIAN_POINT ( 'NONE',  ( 3.749999999999999112, 1.687500000000000000, -5.053300858899108405 ) ) ;
#11266=FACE_OUTER_BOUND ( 'NONE', #9290, .T. ) ;
#11267=CARTESIAN_POINT ( 'NONE',  ( -2.298097038856278029, 3.625000000000000888, -1.201902961143720638 ) ) ;
#11268=CARTESIAN_POINT ( 'NONE',  ( 2.298097038856278029, 13.12499999999999822, -5.798097038856279362 ) ) ;
#11273=CARTESIAN_POINT ( 'NONE',  ( 0.000000000000000000, 7.000000000000000000, -0.2500000000000002220 ) ) ;
#11274=CARTESIAN_POINT ( 'NONE',  ( 1.553300858899109071, 6.437499999999999112, 0.2499999999999989175 ) ) ;
#11275=CARTESIAN_POINT ( 'NONE',  ( 1.553300858899108849, 9.937499999999998224, 0.2499999999999993616 ) ) ;
#11279=CARTESIAN_POINT ( 'NONE',  ( 2.651650429449554203, 11.37500000000000000, -0.8483495705504471296 ) ) ;
#11285=CARTESIAN_POINT ( 'NONE',  ( 0.000000000000000000, 1.000000000000000000, -0.2500000000000002220 ) ) ;
#11287=CARTESIAN_POINT ( 'NONE',  ( 2.298097038856278029, 0.1250000000000001110, -5.798097038856279362 ) ) ;
#11294=CARTESIAN_POINT ( 'NONE',  ( 1.346194077712561166, 7.437499999999999112, -0.2500000000000011102 ) ) ;
#11296=CARTESIAN_POINT ( 'NONE',  ( 3.749999999999999112, 13.81250000000000000, -1.946699141100892039 ) ) ;
#11300=CARTESIAN_POINT ( 'NONE',  ( 3.249999999999999556, 10.75000000000000000, -3.500000000000000000 ) ) ;
#11301=CARTESIAN_POINT ( 'NONE',  ( -0.3766621274091715987, 0.2858031308077496613, -0.04317668481647501943 ) ) ;
#11303=CARTESIAN_POINT ( 'NONE',  ( -2.298097038856278918, 8.375000000000000000, -5.798097038856277585 ) ) ;
#11310=CARTESIAN_POINT ( 'NONE',  ( -3.749999999999999556, 1.312500000000000444, -5.053300858899104853 ) ) ;
#11311=CARTESIAN_POINT ( 'NONE',  ( 1.346194077712561166, 15.43750000000000178, -0.2500000000000011102 ) ) ;
#11312=CARTESIAN_POINT ( 'NONE',  ( -1.346194077712559389, 1.062500000000000222, -0.2500000000000002220 ) ) ;
#11315=CARTESIAN_POINT ( 'NONE',  ( -1.346194077712559389, 12.43750000000000000, -6.749999999999999112 ) ) ;
#11327=CARTESIAN_POINT ( 'NONE',  ( -2.298097038856278918, 5.375000000000000000, -5.798097038856277585 ) ) ;
#11329=CARTESIAN_POINT ( 'NONE',  ( 3.749999999999999112, 2.187500000000000000, -5.053300858899108405 ) ) ;
#11332=CARTESIAN_POINT ( 'NONE',  ( -4.592425496802573972E-16, 4.500000000000000888, -7.249999999999999112 ) ) ;
#11335=CARTESIAN_POINT ( 'NONE',  ( 3.749999999999999556, 0.8125000000000001110, -1.946699141100892261 ) ) ;
#11338=CARTESIAN_POINT ( 'NONE',  ( -3.249999999999999556, 11.18749999999999822, -2.153805922287440833 ) ) ;
#11341=CARTESIAN_POINT ( 'NONE',  ( 1.346194077712558279, 3.062500000000000000, -6.750000000000000888 ) ) ;
#11344=CARTESIAN_POINT ( 'NONE',  ( 0.000000000000000000, 4.499999999999999112, 0.2499999999999998057 ) ) ;
#11345=CARTESIAN_POINT ( 'NONE',  ( 1.553300858899108849, 7.937500000000000000, 0.2499999999999993616 ) ) ;
#11350=CARTESIAN_POINT ( 'NONE',  ( -4.592425496802573972E-16, 12.00000000000000178, -7.250000000000000000 ) ) ;
#11360=CARTESIAN_POINT ( 'NONE',  ( 1.346194077712558279, 4.062500000000001776, -6.750000000000000888 ) ) ;
#11368=CARTESIAN_POINT ( 'NONE',  ( -3.249999999999999556, 10.31250000000000000, -4.846194077712557835 ) ) ;
#11371=CARTESIAN_POINT ( 'NONE',  ( -1.346194077712559167, 9.937500000000001776, -6.749999999999999112 ) ) ;
#11373=CARTESIAN_POINT ( 'NONE',  ( 2.651650429449553759, 13.87500000000000000, -0.8483495705504471296 ) ) ;
#11378=CARTESIAN_POINT ( 'NONE',  ( -2.298097038856278473, 11.12500000000000000, -1.201902961143720416 ) ) ;
#11383=CARTESIAN_POINT ( 'NONE',  ( 2.298097038856279362, 8.875000000000001776, -1.201902961143720860 ) ) ;
#11389=CARTESIAN_POINT ( 'NONE',  ( 2.651650429449553314, 15.37500000000000178, -0.8483495705504476847 ) ) ;
#11390=CARTESIAN_POINT ( 'NONE',  ( -1.346194077712558945, 13.56250000000000000, -0.2500000000000002220 ) ) ;
#11391=CARTESIAN_POINT ( 'NONE',  ( 3.249999999999998224, 14.18750000000000178, -4.846194077712561388 ) ) ;
#11392=ORIENTED_EDGE ( 'NONE', *, *, #12738, .T. ) ;
#11395=CARTESIAN_POINT ( 'NONE',  ( 3.249999999999998668, 10.68750000000000000, -4.846194077712560500 ) ) ;
#11407=CARTESIAN_POINT ( 'NONE',  ( 3.249999999999998668, 3.687500000000000444, -4.846194077712560500 ) ) ;
#11409=CARTESIAN_POINT ( 'NONE',  ( -3.750000000000000000, 3.812500000000000888, -5.053300858899105741 ) ) ;
#11414=CARTESIAN_POINT ( 'NONE',  ( -3.749999999999999556, 6.312500000000000888, -5.053300858899104853 ) ) ;
#11417=CARTESIAN_POINT ( 'NONE',  ( -1.553300858899107073, 3.437500000000000000, -7.250000000000000000 ) ) ;
#11422=CARTESIAN_POINT ( 'NONE',  ( -2.298097038856278029, 1.625000000000000000, -1.201902961143720638 ) ) ;
#11425=CARTESIAN_POINT ( 'NONE',  ( 1.553300858899109071, 7.437499999999999112, 0.2499999999999989175 ) ) ;
#11426=CARTESIAN_POINT ( 'NONE',  ( 2.651650429449553759, 13.87500000000000000, -0.8483495705504471296 ) ) ;
#11429=CARTESIAN_POINT ( 'NONE',  ( 3.249999999999998668, 8.687500000000000000, -4.846194077712560500 ) ) ;
#11430=CARTESIAN_POINT ( 'NONE',  ( -3.249999999999999112, 0.6875000000000000000, -2.153805922287440833 ) ) ;
#11440=CARTESIAN_POINT ( 'NONE',  ( 2.298097038856279362, 4.375000000000000888, -1.201902961143720860 ) ) ;
#11447=CARTESIAN_POINT ( 'NONE',  ( -3.249999999999999112, 11.81250000000000178, -4.846194077712558723 ) ) ;
#11451=CARTESIAN_POINT ( 'NONE',  ( -2.651650429449552870, 13.12500000000000000, -0.8483495705504462414 ) ) ;
#11454=CARTESIAN_POINT ( 'NONE',  ( 0.000000000000000000, 11.00000000000000000, -0.2500000000000002220 ) ) ;
#11457=CARTESIAN_POINT ( 'NONE',  ( 3.249999999999998668, 6.687500000000000888, -4.846194077712560500 ) ) ;
#11464=CARTESIAN_POINT ( 'NONE',  ( 3.750000000000000000, 2.750000000000000000, -3.500000000000000444 ) ) ;
#11465=CARTESIAN_POINT ( 'NONE',  ( 0.000000000000000000, 14.50000000000000355, -0.2500000000000002220 ) ) ;
#11467=ORIENTED_EDGE ( 'NONE', *, *, #2714, .T. ) ;
#11468=CARTESIAN_POINT ( 'NONE',  ( 2.298097038856279362, 11.87500000000000000, -1.201902961143720860 ) ) ;
#11469=EDGE_CURVE ( 'NONE', #2776, #13242, #12966, .T. ) ;
#11472=CARTESIAN_POINT ( 'NONE',  ( -1.346194077712559389, 7.437500000000000888, -6.749999999999999112 ) ) ;
#11481=CARTESIAN_POINT ( 'NONE',  ( 2.298097038856278473, 9.625000000000000000, -5.798097038856279362 ) ) ;
#11485=CARTESIAN_POINT ( 'NONE',  ( -3.980102097228897245E-16, 4.500000000000000888, -6.749999999999999112 ) ) ;
#11488=CARTESIAN_POINT ( 'NONE',  ( 1.553300858899109516, 2.437500000000000444, 0.2499999999999993616 ) ) ;
#11491=CARTESIAN_POINT ( 'NONE',  ( 2.298097038856279362, 0.8750000000000000000, -1.201902961143720860 ) ) ;
#11492=CARTESIAN_POINT ( 'NONE',  ( -1.553300858899107295, 4.437500000000000888, -7.250000000000000000 ) ) ;
#11500=CARTESIAN_POINT ( 'NONE',  ( -2.298097038856278029, 5.625000000000000000, -1.201902961143720638 ) ) ;
#11503=CARTESIAN_POINT ( 'NONE',  ( 3.749999999999999556, 11.25000000000000178, -3.500000000000000444 ) ) ;
#11505=CARTESIAN_POINT ( 'NONE',  ( 3.749999999999999112, 13.68750000000000000, -5.053300858899108405 ) ) ;
#11509=CARTESIAN_POINT ( 'NONE',  ( 0.000000000000000000, 0.5000000000000001110, -0.2500000000000002220 ) ) ;
#11517=CARTESIAN_POINT ( 'NONE',  ( 2.298097038856279362, 2.375000000000000000, -1.201902961143720860 ) ) ;
#11523=CARTESIAN_POINT ( 'NONE',  ( -3.980102097228897738E-16, 12.00000000000000178, -6.749999999999999112 ) ) ;
#11525=CARTESIAN_POINT ( 'NONE',  ( -1.553300858899106629, 1.562500000000000222, 0.2500000000000002220 ) ) ;
#11532=CARTESIAN_POINT ( 'NONE',  ( -1.346194077712559389, 10.06250000000000000, -0.2500000000000002220 ) ) ;
#11536=ORIENTED_EDGE ( 'NONE', *, *, #438, .T. ) ;
#11537=CARTESIAN_POINT ( 'NONE',  ( -1.553300858899106629, 1.062500000000000222, 0.2500000000000002220 ) ) ;
#11538=CARTESIAN_POINT ( 'NONE',  ( -2.298097038856279362, 14.87500000000000355, -5.798097038856278473 ) ) ;
#11541=CARTESIAN_POINT ( 'NONE',  ( -3.249999999999999112, 1.687499999999999778, -2.153805922287440833 ) ) ;
#11544=CARTESIAN_POINT ( 'NONE',  ( 3.249999999999998668, 2.687500000000000888, -4.846194077712560500 ) ) ;
#11550=CARTESIAN_POINT ( 'NONE',  ( -3.249999999999999556, 11.25000000000000000, -3.499999999999999556 ) ) ;
#11553=CARTESIAN_POINT ( 'NONE',  ( -2.651650429449553314, 9.875000000000000000, -6.151650429449552426 ) ) ;
#11555=CARTESIAN_POINT ( 'NONE',  ( -1.553300858899107073, -0.06249999999999988898, -7.249999999999999112 ) ) ;
#11556=CARTESIAN_POINT ( 'NONE',  ( -3.249999999999999112, 5.687500000000000888, -2.153805922287440833 ) ) ;
#11559=CARTESIAN_POINT ( 'NONE',  ( 0.000000000000000000, 4.000000000000000000, -0.2500000000000002220 ) ) ;
#11560=CARTESIAN_POINT ( 'NONE',  ( 0.000000000000000000, 4.000000000000000000, 0.2500000000000002220 ) ) ;
#11569=CARTESIAN_POINT ( 'NONE',  ( 2.298097038856278029, 9.125000000000001776, -5.798097038856279362 ) ) ;
#11571=CARTESIAN_POINT ( 'NONE',  ( 1.553300858899105963, 9.062500000000003553, -7.249999999999999112 ) ) ;
#11572=CARTESIAN_POINT ( 'NONE',  ( 2.651650429449552870, 12.62500000000000000, -6.151650429449554203 ) ) ;
#11576=CARTESIAN_POINT ( 'NONE',  ( -2.651650429449552870, 13.62500000000000000, -0.8483495705504463524 ) ) ;
#11583=CARTESIAN_POINT ( 'NONE',  ( 2.298097038856279362, 3.875000000000000000, -1.201902961143720860 ) ) ;
#11587=CARTESIAN_POINT ( 'NONE',  ( -2.298097038856278029, 2.625000000000000000, -1.201902961143720638 ) ) ;
#11593=CARTESIAN_POINT ( 'NONE',  ( 3.249999999999999556, 11.25000000000000178, -3.500000000000000000 ) ) ;
#11596=CARTESIAN_POINT ( 'NONE',  ( -1.553300858899106629, 0.5625000000000003331, 0.2500000000000002220 ) ) ;
#11597=CARTESIAN_POINT ( 'NONE',  ( -0.3766621274091715987, -0.1687972351630583345, 0.1491815183709511161 ) ) ;
#11602=CARTESIAN_POINT ( 'NONE',  ( 3.249999999999999112, 7.812500000000000000, -2.153805922287439945 ) ) ;
#11609=ORIENTED_EDGE ( 'NONE', *, *, #13579, .F. ) ;
#11611=CARTESIAN_POINT ( 'NONE',  ( -1.553300858899106629, 3.062500000000000000, 0.2500000000000002220 ) ) ;
#11612=CARTESIAN_POINT ( 'NONE',  ( 0.000000000000000000, 0.4999999999999999445, 0.2499999999999998057 ) ) ;
#11615=CARTESIAN_POINT ( 'NONE',  ( 3.249999999999998224, 1.312500000000000000, -2.153805922287439945 ) ) ;
#11621=CARTESIAN_POINT ( 'NONE',  ( -3.980102097228897245E-16, 2.500000000000000000, -6.749999999999999112 ) ) ;
#11627=CARTESIAN_POINT ( 'NONE',  ( -2.298097038856278473, 12.12500000000000000, -1.201902961143720416 ) ) ;
#11631=CARTESIAN_POINT ( 'NONE',  ( -1.553300858899106629, 10.56249999999999822, 0.2500000000000002220 ) ) ;
#11633=CARTESIAN_POINT ( 'NONE',  ( 2.651650429449554203, 5.375000000000000888, -0.8483495705504471296 ) ) ;
#11634=CARTESIAN_POINT ( 'NONE',  ( -1.346194077712558945, 5.562500000000001776, -0.2500000000000002220 ) ) ;
#11637=CARTESIAN_POINT ( 'NONE',  ( -3.249999999999999556, 1.187500000000000444, -2.153805922287440833 ) ) ;
#11639=CARTESIAN_POINT ( 'NONE',  ( 3.249999999999998668, 11.68750000000000000, -4.846194077712560500 ) ) ;
#11640=CARTESIAN_POINT ( 'NONE',  ( 2.651650429449553759, 5.875000000000000000, -0.8483495705504471296 ) ) ;
#11647=CARTESIAN_POINT ( 'NONE',  ( -3.980102097228897738E-16, 5.999999999999999112, -6.749999999999999112 ) ) ;
#11650=CARTESIAN_POINT ( 'NONE',  ( 1.553300858899105963, 10.06250000000000000, -7.249999999999999112 ) ) ;
#11651=CARTESIAN_POINT ( 'NONE',  ( 0.000000000000000000, 13.00000000000000178, 0.2500000000000002220 ) ) ;
#11654=CARTESIAN_POINT ( 'NONE',  ( -0.2516503215200827648, -0.1858217187662949132, 0.1491815183709512271 ) ) ;
#11655=CARTESIAN_POINT ( 'NONE',  ( -1.553300858899107073, 13.93750000000000000, -7.249999999999999112 ) ) ;
#11662=CARTESIAN_POINT ( 'NONE',  ( 3.249999999999998668, 4.687500000000000888, -4.846194077712560500 ) ) ;
#11663=CIRCLE ( 'NONE', #4276, 0.2500000000000002220 ) ;
#11666=CARTESIAN_POINT ( 'NONE',  ( 3.249999999999998224, 1.187500000000000222, -4.846194077712561388 ) ) ;
#11672=CARTESIAN_POINT ( 'NONE',  ( -3.249999999999999112, 13.81250000000000178, -4.846194077712558723 ) ) ;
#11675=CARTESIAN_POINT ( 'NONE',  ( 1.553300858899105963, 2.062500000000000000, -7.250000000000000888 ) ) ;
#11681=CARTESIAN_POINT ( 'NONE',  ( -3.980102097228897245E-16, 13.50000000000000000, -6.749999999999999112 ) ) ;
#11687=CARTESIAN_POINT ( 'NONE',  ( 1.553300858899105963, 4.562500000000000888, -7.250000000000000888 ) ) ;
#11689=CARTESIAN_POINT ( 'NONE',  ( -1.553300858899107073, 2.937500000000000444, -7.249999999999999112 ) ) ;
#11692=VERTEX_POINT ( 'NONE', #443 ) ;
#11693=CARTESIAN_POINT ( 'NONE',  ( 1.346194077712560944, 13.93750000000000000, -0.2500000000000010547 ) ) ;
#11697=CARTESIAN_POINT ( 'NONE',  ( -2.298097038856278473, 5.125000000000000000, -1.201902961143720416 ) ) ;
#11704=CARTESIAN_POINT ( 'NONE',  ( -1.346194077712559167, 12.43750000000000000, -6.749999999999999112 ) ) ;
#11708=CARTESIAN_POINT ( 'NONE',  ( 3.750000000000000000, 6.312500000000000000, -1.946699141100892705 ) ) ;
#11709=CARTESIAN_POINT ( 'NONE',  ( -2.298097038856279362, 7.874999999999999112, -5.798097038856278473 ) ) ;
#11712=CARTESIAN_POINT ( 'NONE',  ( 2.298097038856279362, 3.875000000000000000, -1.201902961143720860 ) ) ;
#11713=CARTESIAN_POINT ( 'NONE',  ( 1.553300858899105963, 9.562500000000000000, -7.250000000000000888 ) ) ;
#11720=CARTESIAN_POINT ( 'NONE',  ( 3.249999999999999556, 7.250000000000000000, -3.500000000000000000 ) ) ;
#11722=CARTESIAN_POINT ( 'NONE',  ( -3.750000000000000000, 9.812500000000000000, -5.053300858899105741 ) ) ;
#11723=CARTESIAN_POINT ( 'NONE',  ( 3.749999999999999556, 11.81250000000000000, -1.946699141100892261 ) ) ;
#11726=CARTESIAN_POINT ( 'NONE',  ( 2.651650429449554203, 12.37500000000000178, -0.8483495705504471296 ) ) ;
#11732=CARTESIAN_POINT ( 'NONE',  ( -3.980102097228897245E-16, 3.500000000000000000, -6.749999999999999112 ) ) ;
#11735=CARTESIAN_POINT ( 'NONE',  ( -2.298097038856278029, 8.624999999999998224, -1.201902961143720638 ) ) ;
#11736=ORIENTED_EDGE ( 'NONE', *, *, #12902, .T. ) ;
#11740=CARTESIAN_POINT ( 'NONE',  ( -2.298097038856278473, 0.1250000000000000000, -1.201902961143720416 ) ) ;
#11741=CARTESIAN_POINT ( 'NONE',  ( 2.298097038856278029, 14.12500000000000000, -5.798097038856279362 ) ) ;
#11743=CARTESIAN_POINT ( 'NONE',  ( 1.553300858899109516, 1.437500000000000000, 0.2499999999999993616 ) ) ;
#11746=CARTESIAN_POINT ( 'NONE',  ( 0.3766621274091715987, -0.2500000000000000000, -7.146945437571387671 ) ) ;
#11748=CARTESIAN_POINT ( 'NONE',  ( 3.249999999999998668, 12.68750000000000178, -4.846194077712560500 ) ) ;
#11752=PRODUCT_DEFINITION_SHAPE ( 'NONE', 'NONE',  #8454 ) ;
#11757=CARTESIAN_POINT ( 'NONE',  ( -3.749999999999999556, 6.312500000000000888, -5.053300858899104853 ) ) ;
#11758=CARTESIAN_POINT ( 'NONE',  ( 1.553300858899105963, 3.062500000000000000, -7.249999999999999112 ) ) ;
#11761=CARTESIAN_POINT ( 'NONE',  ( -1.346194077712559167, 1.937500000000000222, -6.749999999999999112 ) ) ;
#11765=CARTESIAN_POINT ( 'NONE',  ( 3.249999999999999556, 4.750000000000000000, -3.500000000000000000 ) ) ;
#11773=ORIENTED_EDGE ( 'NONE', *, *, #10640, .F. ) ;
#11777=CARTESIAN_POINT ( 'NONE',  ( 0.000000000000000000, 4.499999999999999112, 0.2500000000000002220 ) ) ;
#11779=CARTESIAN_POINT ( 'NONE',  ( -1.346194077712558945, 8.562500000000000000, -0.2500000000000002220 ) ) ;
#11783=CARTESIAN_POINT ( 'NONE',  ( -2.298097038856278918, 3.375000000000000000, -5.798097038856277585 ) ) ;
#11784=CARTESIAN_POINT ( 'NONE',  ( 0.000000000000000000, 8.000000000000000000, 0.2500000000000002220 ) ) ;
#11790=ORIENTED_EDGE ( 'NONE', *, *, #12707, .T. ) ;
#11793=CARTESIAN_POINT ( 'NONE',  ( -3.750000000000000000, 12.68750000000000178, -1.946699141100893149 ) ) ;
#11797=CARTESIAN_POINT ( 'NONE',  ( 1.346194077712561166, 2.437500000000000444, -0.2500000000000011102 ) ) ;
#11804=CARTESIAN_POINT ( 'NONE',  ( 3.249999999999999112, 1.812500000000000000, -2.153805922287439945 ) ) ;
#11807=CARTESIAN_POINT ( 'NONE',  ( 2.298097038856278029, 5.125000000000000888, -5.798097038856279362 ) ) ;
#11812=CARTESIAN_POINT ( 'NONE',  ( -0.3766621274091713767, 0.2975415354274087432, -7.146945437571386783 ) ) ;
#11813=CARTESIAN_POINT ( 'NONE',  ( 2.651650429449553314, 3.375000000000000444, -0.8483495705504476847 ) ) ;
#11814=CARTESIAN_POINT ( 'NONE',  ( 3.749999999999999556, 4.812500000000000888, -1.946699141100892261 ) ) ;
#11816=CARTESIAN_POINT ( 'NONE',  ( -1.553300858899107073, 3.937500000000001332, -7.249999999999999112 ) ) ;
#11821=CARTESIAN_POINT ( 'NONE',  ( -1.346194077712559389, 12.43750000000000000, -6.749999999999999112 ) ) ;
#11828=CARTESIAN_POINT ( 'NONE',  ( -2.651650429449552870, 3.125000000000000000, -0.8483495705504462414 ) ) ;
#11829=CARTESIAN_POINT ( 'NONE',  ( 2.651650429449552870, 5.125000000000000000, -6.151650429449553314 ) ) ;
#11833=CARTESIAN_POINT ( 'NONE',  ( -2.298097038856278029, 0.6249999999999998890, -1.201902961143720638 ) ) ;
#11839=CARTESIAN_POINT ( 'NONE',  ( -1.346194077712559389, 3.062500000000000000, -0.2500000000000002220 ) ) ;
#11844=CARTESIAN_POINT ( 'NONE',  ( -2.298097038856278473, 13.12500000000000000, -1.201902961143720416 ) ) ;
#11848=CARTESIAN_POINT ( 'NONE',  ( 1.553300858899105963, 6.062500000000000888, -7.250000000000000888 ) ) ;
#11849=CARTESIAN_POINT ( 'NONE',  ( 3.249999999999999556, 6.250000000000000888, -3.500000000000000000 ) ) ;
#11851=AXIS2_PLACEMENT_3D ( 'NONE', #13604, #617, #2929 ) ;
#11854=CARTESIAN_POINT ( 'NONE',  ( 2.298097038856279362, 2.875000000000000000, -1.201902961143720860 ) ) ;
#11869=CARTESIAN_POINT ( 'NONE',  ( 1.553300858899109071, 11.43750000000000178, 0.2499999999999989175 ) ) ;
#11873=CARTESIAN_POINT ( 'NONE',  ( 3.249999999999998224, 2.187500000000000000, -4.846194077712561388 ) ) ;
#11882=CARTESIAN_POINT ( 'NONE',  ( 2.298097038856278473, 3.625000000000000000, -5.798097038856279362 ) ) ;
#11884=CARTESIAN_POINT ( 'NONE',  ( 1.346194077712561166, 7.437500000000000000, -0.2500000000000011102 ) ) ;
#11889=CARTESIAN_POINT ( 'NONE',  ( 3.249999999999999112, 0.8125000000000001110, -2.153805922287439945 ) ) ;
#11890=CARTESIAN_POINT ( 'NONE',  ( 1.553300858899109071, 1.437500000000000000, 0.2499999999999989175 ) ) ;
#11891=CARTESIAN_POINT ( 'NONE',  ( -1.553300858899107073, 5.437500000000001776, -7.250000000000000000 ) ) ;
#11894=CARTESIAN_POINT ( 'NONE',  ( -2.651650429449553314, 6.875000000000000000, -6.151650429449552426 ) ) ;
#11899=CARTESIAN_POINT ( 'NONE',  ( 2.298097038856279362, 10.87500000000000178, -1.201902961143720860 ) ) ;
#11901=CARTESIAN_POINT ( 'NONE',  ( 3.249999999999998668, 11.68750000000000000, -4.846194077712560500 ) ) ;
#11905=CARTESIAN_POINT ( 'NONE',  ( 1.553300858899105963, 8.062500000000001776, -7.250000000000000888 ) ) ;
#11909=CARTESIAN_POINT ( 'NONE',  ( -3.750000000000000000, 5.250000000000000000, -3.499999999999999112 ) ) ;
#11910=CARTESIAN_POINT ( 'NONE',  ( 1.553300858899109071, 4.437499999999999112, 0.2499999999999989175 ) ) ;
#11914=CARTESIAN_POINT ( 'NONE',  ( 3.249999999999998224, 6.187500000000001776, -4.846194077712561388 ) ) ;
#11917=CARTESIAN_POINT ( 'NONE',  ( -2.298097038856278918, 6.375000000000000888, -5.798097038856277585 ) ) ;
#11922=ORIENTED_EDGE ( 'NONE', *, *, #14541, .F. ) ;
#11930=CARTESIAN_POINT ( 'NONE',  ( -3.749999999999999556, 6.750000000000001776, -3.499999999999999112 ) ) ;
#11931=CARTESIAN_POINT ( 'NONE',  ( -1.346194077712558945, 12.56250000000000355, -0.2500000000000002220 ) ) ;
#11935=CARTESIAN_POINT ( 'NONE',  ( 3.249999999999999556, 8.750000000000000000, -3.500000000000000000 ) ) ;
#11936=CIRCLE ( 'NONE', #4311, 0.2500000000000002220 ) ;
#11946=CARTESIAN_POINT ( 'NONE',  ( 2.651650429449553314, 12.37500000000000178, -0.8483495705504476847 ) ) ;
#11950=CARTESIAN_POINT ( 'NONE',  ( -2.298097038856279362, 3.875000000000000444, -5.798097038856278473 ) ) ;
#11959=CARTESIAN_POINT ( 'NONE',  ( -1.346194077712558945, 5.062500000000000888, -0.2500000000000002220 ) ) ;
#11962=CARTESIAN_POINT ( 'NONE',  ( 0.000000000000000000, 0.4999999999999999445, -0.2500000000000002220 ) ) ;
#11964=CARTESIAN_POINT ( 'NONE',  ( -3.249999999999999556, 6.750000000000001776, -3.500000000000000000 ) ) ;
#11971=CARTESIAN_POINT ( 'NONE',  ( 3.249999999999998668, 2.687500000000000888, -4.846194077712560500 ) ) ;
#11972=CARTESIAN_POINT ( 'NONE',  ( 3.749999999999999112, 2.312500000000000000, -1.946699141100893149 ) ) ;
#11973=CARTESIAN_POINT ( 'NONE',  ( -3.750000000000000000, 6.187500000000000000, -1.946699141100892927 ) ) ;
#11975=CARTESIAN_POINT ( 'NONE',  ( 3.750000000000000000, 5.312500000000000000, -1.946699141100892705 ) ) ;
#11980=CARTESIAN_POINT ( 'NONE',  ( -3.249999999999999556, 14.18750000000000000, -2.153805922287440833 ) ) ;
#11983=CARTESIAN_POINT ( 'NONE',  ( -3.749999999999999556, 10.75000000000000000, -3.499999999999999112 ) ) ;
#11987=CARTESIAN_POINT ( 'NONE',  ( 3.749999999999999112, 9.812500000000000000, -1.946699141100892039 ) ) ;
#11988=CARTESIAN_POINT ( 'NONE',  ( -4.592425496802573972E-16, 4.000000000000000000, -7.250000000000000000 ) ) ;
#11991=CARTESIAN_POINT ( 'NONE',  ( -1.346194077712559167, 4.937500000000000000, -6.749999999999999112 ) ) ;
#11995=CARTESIAN_POINT ( 'NONE',  ( -3.980102097228897245E-16, 8.500000000000000000, -6.749999999999999112 ) ) ;
#11999=VERTEX_POINT ( 'NONE', #11076 ) ;
#12005=CARTESIAN_POINT ( 'NONE',  ( -3.750000000000000000, 10.81250000000000000, -5.053300858899105741 ) ) ;
#12006=CARTESIAN_POINT ( 'NONE',  ( 3.249999999999998224, 6.312500000000000000, -2.153805922287439945 ) ) ;
#12007=CARTESIAN_POINT ( 'NONE',  ( -2.298097038856278029, 8.624999999999998224, -1.201902961143720638 ) ) ;
#12010=CARTESIAN_POINT ( 'NONE',  ( 3.249999999999999112, 5.812500000000000000, -2.153805922287439945 ) ) ;
#12022=CARTESIAN_POINT ( 'NONE',  ( -3.249999999999999556, 2.187500000000000444, -2.153805922287440833 ) ) ;
#12024=CARTESIAN_POINT ( 'NONE',  ( 3.749999999999999556, 15.25000000000000355, -3.500000000000000444 ) ) ;
#12027=CARTESIAN_POINT ( 'NONE',  ( 3.249999999999999556, 3.250000000000000000, -3.500000000000000000 ) ) ;
#12035=CARTESIAN_POINT ( 'NONE',  ( -2.298097038856278473, 6.125000000000000000, -1.201902961143720416 ) ) ;
#12037=CARTESIAN_POINT ( 'NONE',  ( -2.298097038856278473, 14.12500000000000000, -1.201902961143720416 ) ) ;
#12038=CARTESIAN_POINT ( 'NONE',  ( -3.980102097228897738E-16, 5.000000000000000000, -6.749999999999999112 ) ) ;
#12042=CARTESIAN_POINT ( 'NONE',  ( 1.346194077712558057, 4.562500000000000888, -6.750000000000000000 ) ) ;
#12043=CARTESIAN_POINT ( 'NONE',  ( -1.553300858899106629, 0.5625000000000001110, 0.2499999999999998335 ) ) ;
#12044=CARTESIAN_POINT ( 'NONE',  ( -2.651650429449552870, 5.125000000000000000, -0.8483495705504462414 ) ) ;
#12046=CARTESIAN_POINT ( 'NONE',  ( -1.553300858899106629, 4.562500000000000000, 0.2500000000000002220 ) ) ;
#12054=DIRECTION ( 'NONE',  ( 0.000000000000000000, 0.000000000000000000, -1.000000000000000000 ) ) ;
#12059=CARTESIAN_POINT ( 'NONE',  ( 3.750000000000000000, 11.31250000000000000, -1.946699141100892705 ) ) ;
#12063=CARTESIAN_POINT ( 'NONE',  ( -4.592425496802573972E-16, 7.500000000000000000, -7.249999999999999112 ) ) ;
#12064=CARTESIAN_POINT ( 'NONE',  ( 1.553300858899109071, 7.437499999999999112, 0.2499999999999989175 ) ) ;
#12066=ORIENTED_EDGE ( 'NONE', *, *, #13823, .T. ) ;
#12068=CARTESIAN_POINT ( 'NONE',  ( -1.346194077712559167, 2.937500000000000444, -6.749999999999999112 ) ) ;
#12069=CARTESIAN_POINT ( 'NONE',  ( 2.651650429449553759, 7.875000000000000000, -0.8483495705504471296 ) ) ;
#12072=CARTESIAN_POINT ( 'NONE',  ( -2.298097038856278473, 6.125000000000000000, -1.201902961143720416 ) ) ;
#12079=DIRECTION ( 'NONE',  ( 0.000000000000000000, 0.000000000000000000, 1.000000000000000000 ) ) ;
#12084=CARTESIAN_POINT ( 'NONE',  ( 2.651650429449552870, 14.12500000000000000, -6.151650429449553314 ) ) ;
#12085=CARTESIAN_POINT ( 'NONE',  ( -2.298097038856278029, 12.62500000000000000, -1.201902961143720638 ) ) ;
#12086=CARTESIAN_POINT ( 'NONE',  ( 2.298097038856279362, 10.37500000000000000, -1.201902961143720860 ) ) ;
#12089=CARTESIAN_POINT ( 'NONE',  ( -3.249999999999999556, 6.250000000000000000, -3.499999999999999556 ) ) ;
#12099=CARTESIAN_POINT ( 'NONE',  ( -1.346194077712559389, 9.062499999999998224, -0.2500000000000002220 ) ) ;
#12100=AXIS2_PLACEMENT_3D ( 'NONE', #14398, #3797, #12054 ) ;
#12101=CARTESIAN_POINT ( 'NONE',  ( 2.298097038856278029, 14.12500000000000000, -5.798097038856279362 ) ) ;
#12102=CARTESIAN_POINT ( 'NONE',  ( 1.553300858899105963, 14.56250000000000000, -7.250000000000000888 ) ) ;
#12106=CARTESIAN_POINT ( 'NONE',  ( 3.749999999999998668, 14.18750000000000178, -5.053300858899108405 ) ) ;
#12110=CARTESIAN_POINT ( 'NONE',  ( -2.298097038856279362, 2.875000000000000000, -5.798097038856278473 ) ) ;
#12116=DIRECTION ( 'NONE',  ( -0.000000000000000000, -1.000000000000000000, -0.000000000000000000 ) ) ;
#12119=CARTESIAN_POINT ( 'NONE',  ( -2.298097038856278918, 7.375000000000000888, -5.798097038856277585 ) ) ;
#12121=CARTESIAN_POINT ( 'NONE',  ( 0.000000000000000000, 14.00000000000000000, -0.2500000000000002220 ) ) ;
#12123=CARTESIAN_POINT ( 'NONE',  ( -2.298097038856278029, 11.62500000000000000, -1.201902961143720638 ) ) ;
#12128=EDGE_CURVE ( 'NONE', #4833, #7693, #5579, .T. ) ;
#12129=CARTESIAN_POINT ( 'NONE',  ( 2.298097038856278473, 5.625000000000000000, -5.798097038856279362 ) ) ;
#12130=CARTESIAN_POINT ( 'NONE',  ( 3.249999999999998224, 15.18750000000000355, -4.846194077712561388 ) ) ;
#12131=CARTESIAN_POINT ( 'NONE',  ( -4.592425496802573972E-16, 4.500000000000000888, -7.249999999999999112 ) ) ;
#12133=CARTESIAN_POINT ( 'NONE',  ( 2.651650429449554203, 4.375000000000000888, -0.8483495705504471296 ) ) ;
#12141=CARTESIAN_POINT ( 'NONE',  ( -2.651650429449553314, 13.87500000000000178, -6.151650429449552426 ) ) ;
#12146=CARTESIAN_POINT ( 'NONE',  ( 1.553300858899108849, 10.93750000000000000, 0.2499999999999993616 ) ) ;
#12147=CARTESIAN_POINT ( 'NONE',  ( -2.651650429449552870, 8.875000000000000000, -6.151650429449552426 ) ) ;
#12151=CARTESIAN_POINT ( 'NONE',  ( -2.298097038856278029, 3.625000000000000888, -1.201902961143720638 ) ) ;
#12153=CARTESIAN_POINT ( 'NONE',  ( 1.553300858899105963, 11.56249999999999822, -7.250000000000000888 ) ) ;
#12157=CARTESIAN_POINT ( 'NONE',  ( -3.249999999999999556, 9.187500000000000000, -2.153805922287440833 ) ) ;
#12160=B_SPLINE_CURVE_WITH_KNOTS ( 'NONE', 3,
 ( #12748, #9262, #11654, #3384 ),
 .UNSPECIFIED., .F., .F.,
 ( 4, 4 ),
 ( 0.000000000000000000, 0.0003780032935241441918 ),
 .UNSPECIFIED. ) ;
#12169=CARTESIAN_POINT ( 'NONE',  ( 3.749999999999999556, 12.25000000000000000, -3.500000000000000444 ) ) ;
#12171=CARTESIAN_POINT ( 'NONE',  ( -3.249999999999999112, 9.687500000000000000, -2.153805922287440833 ) ) ;
#12172=CARTESIAN_POINT ( 'NONE',  ( 1.346194077712558279, 12.06250000000000000, -6.750000000000000888 ) ) ;
#12174=CARTESIAN_POINT ( 'NONE',  ( 1.346194077712560944, 7.937500000000000888, -0.2500000000000010547 ) ) ;
#12175=ADVANCED_FACE ( 'NONE', ( #11233 ), #7894, .F. ) ;
#12183=CARTESIAN_POINT ( 'NONE',  ( -3.249999999999999556, 1.250000000000000000, -3.499999999999999556 ) ) ;
#12184=CARTESIAN_POINT ( 'NONE',  ( -2.651650429449552870, 13.12500000000000000, -0.8483495705504462414 ) ) ;
#12189=CARTESIAN_POINT ( 'NONE',  ( 2.651650429449553759, 1.875000000000000000, -0.8483495705504471296 ) ) ;
#12192=CARTESIAN_POINT ( 'NONE',  ( -3.750000000000000000, 1.250000000000000000, -3.499999999999999112 ) ) ;
#12200=CARTESIAN_POINT ( 'NONE',  ( 2.298097038856279362, 7.875000000000000000, -1.201902961143720860 ) ) ;
#12202=CARTESIAN_POINT ( 'NONE',  ( -3.249999999999999556, 13.25000000000000000, -3.499999999999999556 ) ) ;
#12203=CARTESIAN_POINT ( 'NONE',  ( 3.249999999999998224, 11.31250000000000000, -2.153805922287439945 ) ) ;
#12207=CARTESIAN_POINT ( 'NONE',  ( -3.249999999999999556, 6.187500000000000888, -2.153805922287440833 ) ) ;
#12208=VECTOR ( 'NONE', #10493, 1000.000000000000000 ) ;
#12209=CARTESIAN_POINT ( 'NONE',  ( -3.750000000000000000, 4.812500000000000000, -5.053300858899105741 ) ) ;
#12210=CARTESIAN_POINT ( 'NONE',  ( 2.651650429449552870, 8.625000000000000000, -6.151650429449554203 ) ) ;
#12212=CARTESIAN_POINT ( 'NONE',  ( -3.750000000000000000, 4.687500000000000888, -1.946699141100893149 ) ) ;
#12220=CARTESIAN_POINT ( 'NONE',  ( 3.249999999999999556, 14.75000000000000178, -3.500000000000000000 ) ) ;
#12223=CARTESIAN_POINT ( 'NONE',  ( -2.298097038856278029, 0.6250000000000002220, -1.201902961143720638 ) ) ;
#12224=ORIENTED_EDGE ( 'NONE', *, *, #7140, .T. ) ;
#12227=CARTESIAN_POINT ( 'NONE',  ( -2.651650429449552870, 10.12500000000000000, -0.8483495705504462414 ) ) ;
#12228=CARTESIAN_POINT ( 'NONE',  ( 3.749999999999999112, 8.312500000000003553, -1.946699141100893149 ) ) ;
#12232=CARTESIAN_POINT ( 'NONE',  ( -3.980102097228897738E-16, 3.000000000000000444, -6.749999999999999112 ) ) ;
#12233=CARTESIAN_POINT ( 'NONE',  ( 3.749999999999998668, 9.687500000000000000, -5.053300858899107517 ) ) ;
#12237=CARTESIAN_POINT ( 'NONE',  ( 0.000000000000000000, 8.000000000000000000, -0.2500000000000002220 ) ) ;
#12248=CARTESIAN_POINT ( 'NONE',  ( -2.651650429449552870, 11.87500000000000000, -6.151650429449552426 ) ) ;
#12249=CARTESIAN_POINT ( 'NONE',  ( -3.249999999999999556, 12.75000000000000178, -3.500000000000000000 ) ) ;
#12250=CARTESIAN_POINT ( 'NONE',  ( -3.249999999999999112, 13.81250000000000178, -4.846194077712558723 ) ) ;
#12253=CARTESIAN_POINT ( 'NONE',  ( -2.298097038856278918, 6.375000000000000888, -5.798097038856277585 ) ) ;
#12263=CARTESIAN_POINT ( 'NONE',  ( 1.346194077712561166, 13.43750000000000178, -0.2500000000000011102 ) ) ;
#12264=CARTESIAN_POINT ( 'NONE',  ( 2.651650429449553759, 13.87500000000000000, -0.8483495705504471296 ) ) ;
#12268=CARTESIAN_POINT ( 'NONE',  ( 3.749999999999999112, 0.8125000000000001110, -1.946699141100892039 ) ) ;
#12272=CARTESIAN_POINT ( 'NONE',  ( -2.651650429449552870, 0.1250000000000000278, -0.8483495705504462414 ) ) ;
#12277=CARTESIAN_POINT ( 'NONE',  ( 1.346194077712558279, 7.562500000000000000, -6.750000000000000000 ) ) ;
#12279=CARTESIAN_POINT ( 'NONE',  ( -1.346194077712559389, 14.06249999999999822, -0.2500000000000002220 ) ) ;
#12280=CARTESIAN_POINT ( 'NONE',  ( 1.346194077712561166, 12.43750000000000000, -0.2500000000000011102 ) ) ;
#12283=CARTESIAN_POINT ( 'NONE',  ( 3.249999999999998668, 3.687500000000000444, -4.846194077712560500 ) ) ;
#12284=CARTESIAN_POINT ( 'NONE',  ( 1.553300858899109071, 3.437500000000000444, 0.2499999999999989175 ) ) ;
#12285=CARTESIAN_POINT ( 'NONE',  ( 1.553300858899105963, 9.562500000000000000, -7.250000000000000000 ) ) ;
#12288=CARTESIAN_POINT ( 'NONE',  ( -1.553300858899106629, 11.56250000000000178, 0.2500000000000002220 ) ) ;
#12295=CARTESIAN_POINT ( 'NONE',  ( -4.592425496802573972E-16, 12.00000000000000178, -7.250000000000000000 ) ) ;
#12298=CARTESIAN_POINT ( 'NONE',  ( -3.749999999999999556, 8.312500000000000000, -5.053300858899104853 ) ) ;
#12299=CARTESIAN_POINT ( 'NONE',  ( 0.000000000000000000, 7.499999999999999112, 0.2499999999999998057 ) ) ;
#12301=CARTESIAN_POINT ( 'NONE',  ( -1.346194077712558945, 6.562500000000000888, -0.2500000000000002220 ) ) ;
#12302=CARTESIAN_POINT ( 'NONE',  ( 3.749999999999999112, 14.81250000000000000, -1.946699141100892039 ) ) ;
#12306=CARTESIAN_POINT ( 'NONE',  ( 3.249999999999999112, 10.81250000000000178, -2.153805922287439945 ) ) ;
#12308=DIRECTION ( 'NONE',  ( 0.000000000000000000, 0.000000000000000000, 1.000000000000000000 ) ) ;
#12315=CARTESIAN_POINT ( 'NONE',  ( -3.749999999999999556, 10.75000000000000178, -3.499999999999999112 ) ) ;
#12316=CARTESIAN_POINT ( 'NONE',  ( -3.980102097228897738E-16, 10.00000000000000000, -6.749999999999999112 ) ) ;
#12317=CARTESIAN_POINT ( 'NONE',  ( 0.000000000000000000, 2.000000000000000000, -0.2500000000000002220 ) ) ;
#12320=CARTESIAN_POINT ( 'NONE',  ( -1.346194077712559389, 9.062499999999998224, -0.2500000000000002220 ) ) ;
#12324=CARTESIAN_POINT ( 'NONE',  ( -0.3766621274091715987, -0.2500000000000000000, -6.863050255469941519 ) ) ;
#12330=CARTESIAN_POINT ( 'NONE',  ( -3.980102097228897738E-16, 14.00000000000000000, -6.749999999999999112 ) ) ;
#12331=CARTESIAN_POINT ( 'NONE',  ( -3.750000000000000000, -0.1874999999999998890, -5.053300858899105741 ) ) ;
#12336=CARTESIAN_POINT ( 'NONE',  ( 0.000000000000000000, 3.061616997868383018E-17, 0.2500000000000002220 ) ) ;
#12347=CARTESIAN_POINT ( 'NONE',  ( -3.249999999999999556, 10.25000000000000000, -3.499999999999999556 ) ) ;
#12349=CARTESIAN_POINT ( 'NONE',  ( 3.249999999999999556, 2.249999999999999556, -3.500000000000000000 ) ) ;
#12350=CARTESIAN_POINT ( 'NONE',  ( -3.249999999999999112, 12.68750000000000000, -2.153805922287440833 ) ) ;
#12354=CARTESIAN_POINT ( 'NONE',  ( -1.346194077712559389, 3.062500000000000000, -0.2500000000000002220 ) ) ;
#12355=CARTESIAN_POINT ( 'NONE',  ( 1.553300858899105963, 5.062500000000000000, -7.249999999999999112 ) ) ;
#12359=CARTESIAN_POINT ( 'NONE',  ( -3.750000000000000000, 11.25000000000000000, -3.499999999999999112 ) ) ;
#12362=CARTESIAN_POINT ( 'NONE',  ( -3.750000000000000000, 9.812500000000000000, -5.053300858899105741 ) ) ;
#12371=CARTESIAN_POINT ( 'NONE',  ( -1.553300858899107073, 13.93750000000000000, -7.249999999999999112 ) ) ;
#12373=PLANE ( 'NONE',  #14395 ) ;
#12375=CARTESIAN_POINT ( 'NONE',  ( -2.651650429449552870, 9.624999999999998224, -0.8483495705504467965 ) ) ;
#12377=CARTESIAN_POINT ( 'NONE',  ( 1.346194077712558279, 8.062500000000001776, -6.750000000000000888 ) ) ;
#12379=CARTESIAN_POINT ( 'NONE',  ( 1.553300858899108849, 13.93750000000000000, 0.2499999999999993616 ) ) ;
#12382=CARTESIAN_POINT ( 'NONE',  ( 0.3766621274091721538, 0.3292059843107342232, -7.146945437571387671 ) ) ;
#12384=CARTESIAN_POINT ( 'NONE',  ( -1.346194077712559389, 10.06250000000000000, -0.2500000000000002220 ) ) ;
#12394=CARTESIAN_POINT ( 'NONE',  ( 0.000000000000000000, 1.000000000000000000, 0.2500000000000002220 ) ) ;
#12395=CARTESIAN_POINT ( 'NONE',  ( 2.298097038856279362, 12.37500000000000178, -1.201902961143720860 ) ) ;
#12396=CARTESIAN_POINT ( 'NONE',  ( 1.346194077712558279, 13.06249999999999822, -6.750000000000000888 ) ) ;
#12398=CARTESIAN_POINT ( 'NONE',  ( -1.346194077712559389, 11.06250000000000000, -0.2500000000000002220 ) ) ;
#12409=CARTESIAN_POINT ( 'NONE',  ( -1.346194077712559389, 6.062500000000000000, -0.2500000000000002220 ) ) ;
#12411=CARTESIAN_POINT ( 'NONE',  ( 3.749999999999998668, 14.68750000000000000, -5.053300858899107517 ) ) ;
#12414=CARTESIAN_POINT ( 'NONE',  ( -2.651650429449552870, 3.125000000000000000, -0.8483495705504462414 ) ) ;
#12429=CARTESIAN_POINT ( 'NONE',  ( 3.249999999999998224, 4.187500000000000888, -4.846194077712561388 ) ) ;
#12430=CARTESIAN_POINT ( 'NONE',  ( -3.249999999999999112, 11.68749999999999822, -2.153805922287440833 ) ) ;
#12433=CARTESIAN_POINT ( 'NONE',  ( -1.346194077712559389, 7.062500000000000000, -0.2500000000000002220 ) ) ;
#12434=CARTESIAN_POINT ( 'NONE',  ( -3.750000000000000000, 6.812500000000000000, -5.053300858899105741 ) ) ;
#12435=CARTESIAN_POINT ( 'NONE',  ( 3.749999999999999112, 9.687500000000000000, -5.053300858899108405 ) ) ;
#12439=CARTESIAN_POINT ( 'NONE',  ( 2.651650429449552870, 10.12500000000000000, -6.151650429449555091 ) ) ;
#12452=CARTESIAN_POINT ( 'NONE',  ( 1.553300858899109516, 14.43750000000000178, 0.2499999999999993616 ) ) ;
#12459=CARTESIAN_POINT ( 'NONE',  ( -3.980102097228897738E-16, 8.000000000000000000, -6.749999999999999112 ) ) ;
#12461=CARTESIAN_POINT ( 'NONE',  ( -3.749999999999999556, 13.18749999999999822, -1.946699141100892927 ) ) ;
#12464=CARTESIAN_POINT ( 'NONE',  ( -1.346194077712559389, 13.06250000000000000, -0.2500000000000002220 ) ) ;
#12465=CARTESIAN_POINT ( 'NONE',  ( -0.3766621274091715987, 0.2004420829692335482, 0.1491815183709511161 ) ) ;
#12467=CARTESIAN_POINT ( 'NONE',  ( -3.249999999999999556, 8.187500000000000000, -2.153805922287440833 ) ) ;
#12471=DIRECTION ( 'NONE',  ( 1.000000000000000000, 0.000000000000000000, 0.000000000000000000 ) ) ;
#12473=CARTESIAN_POINT ( 'NONE',  ( -3.750000000000000000, 0.2500000000000000555, -3.499999999999999112 ) ) ;
#12474=CARTESIAN_POINT ( 'NONE',  ( 3.249999999999998224, 15.18750000000000355, -4.846194077712561388 ) ) ;
#12475=CARTESIAN_POINT ( 'NONE',  ( -3.249999999999999556, 0.2500000000000000000, -3.499999999999999556 ) ) ;
#12478=CARTESIAN_POINT ( 'NONE',  ( -3.249999999999999556, 9.250000000000000000, -3.499999999999999556 ) ) ;
#12481=DIRECTION ( 'NONE',  ( 0.000000000000000000, 0.000000000000000000, 1.000000000000000000 ) ) ;
#12488=CARTESIAN_POINT ( 'NONE',  ( 3.249999999999999556, 4.750000000000000000, -3.500000000000000000 ) ) ;
#12490=CARTESIAN_POINT ( 'NONE',  ( -1.553300858899107073, 2.937500000000000444, -7.249999999999999112 ) ) ;
#12495=CARTESIAN_POINT ( 'NONE',  ( 2.651650429449552870, 3.625000000000000000, -6.151650429449554203 ) ) ;
#12498=CARTESIAN_POINT ( 'NONE',  ( -2.651650429449553314, 1.375000000000000000, -6.151650429449552426 ) ) ;
#12503=CARTESIAN_POINT ( 'NONE',  ( -3.249999999999999112, 3.687500000000000444, -2.153805922287440833 ) ) ;
#12506=CARTESIAN_POINT ( 'NONE',  ( 2.651650429449553314, 4.375000000000000000, -0.8483495705504476847 ) ) ;
#12507=CARTESIAN_POINT ( 'NONE',  ( -1.553300858899107073, 9.437500000000000000, -7.250000000000000000 ) ) ;
#12513=CARTESIAN_POINT ( 'NONE',  ( 1.346194077712558057, 7.562500000000000000, -6.750000000000000000 ) ) ;
#12514=CARTESIAN_POINT ( 'NONE',  ( 0.000000000000000000, 10.49999999999999822, 0.2500000000000002220 ) ) ;
#12522=CARTESIAN_POINT ( 'NONE',  ( -3.249999999999999112, 3.812500000000000888, -4.846194077712558723 ) ) ;
#12523=ORIENTED_EDGE ( 'NONE', *, *, #3847, .T. ) ;
#12529=CARTESIAN_POINT ( 'NONE',  ( -3.249999999999999112, 9.812500000000000000, -4.846194077712558723 ) ) ;
#12533=CARTESIAN_POINT ( 'NONE',  ( -1.553300858899106629, 13.06250000000000000, 0.2500000000000002220 ) ) ;
#12535=ADVANCED_FACE ( 'NONE', ( #8179 ), #5710, .F. ) ;
#12538=CARTESIAN_POINT ( 'NONE',  ( 1.346194077712558057, 13.56250000000000000, -6.750000000000000000 ) ) ;
#12541=CARTESIAN_POINT ( 'NONE',  ( 3.249999999999998668, 8.687500000000000000, -4.846194077712560500 ) ) ;
#12548=CARTESIAN_POINT ( 'NONE',  ( -2.651650429449552870, 1.125000000000000222, -0.8483495705504462414 ) ) ;
#12549=CARTESIAN_POINT ( 'NONE',  ( -2.651650429449552870, 0.8750000000000000000, -6.151650429449552426 ) ) ;
#12550=CARTESIAN_POINT ( 'NONE',  ( 1.346194077712558279, 14.06250000000000178, -6.750000000000000888 ) ) ;
#12552=CARTESIAN_POINT ( 'NONE',  ( 1.346194077712560944, 11.93750000000000000, -0.2500000000000010547 ) ) ;
#12553=CARTESIAN_POINT ( 'NONE',  ( -3.249999999999999556, 11.31249999999999822, -4.846194077712557835 ) ) ;
#12564=CARTESIAN_POINT ( 'NONE',  ( 3.249999999999998668, 2.687500000000000888, -4.846194077712560500 ) ) ;
#12567=CARTESIAN_POINT ( 'NONE',  ( -2.651650429449552870, 3.625000000000000888, -0.8483495705504463524 ) ) ;
#12571=CARTESIAN_POINT ( 'NONE',  ( 1.553300858899105963, 6.562500000000000000, -7.250000000000000888 ) ) ;
#12574=CARTESIAN_POINT ( 'NONE',  ( -3.750000000000000000, 3.250000000000000444, -3.499999999999999112 ) ) ;
#12581=CARTESIAN_POINT ( 'NONE',  ( 3.249999999999998224, 5.187499999999999112, -4.846194077712561388 ) ) ;
#12583=CARTESIAN_POINT ( 'NONE',  ( 3.749999999999999556, 10.25000000000000178, -3.500000000000000444 ) ) ;
#12584=CARTESIAN_POINT ( 'NONE',  ( 3.749999999999999112, 12.68750000000000178, -5.053300858899108405 ) ) ;
#12589=CARTESIAN_POINT ( 'NONE',  ( -3.980102097228897245E-16, 8.500000000000000000, -6.749999999999999112 ) ) ;
#12590=CARTESIAN_POINT ( 'NONE',  ( -4.592425496802573972E-16, 8.999999999999998224, -7.250000000000000000 ) ) ;
#12600=CARTESIAN_POINT ( 'NONE',  ( -3.980102097228897738E-16, 3.000000000000000444, -6.749999999999999112 ) ) ;
#12609=CARTESIAN_POINT ( 'NONE',  ( 3.249999999999998224, 10.31250000000000000, -2.153805922287439945 ) ) ;
#12611=CARTESIAN_POINT ( 'NONE',  ( -1.553300858899107295, 13.43749999999999822, -7.250000000000000000 ) ) ;
#12615=CARTESIAN_POINT ( 'NONE',  ( 3.249999999999999112, 11.81249999999999822, -2.153805922287439945 ) ) ;
#12616=AXIS2_PLACEMENT_3D ( 'NONE', #7175, #9355, #87 ) ;
#12619=CARTESIAN_POINT ( 'NONE',  ( -3.980102097228897245E-16, 7.500000000000000000, -6.749999999999999112 ) ) ;
#12626=CARTESIAN_POINT ( 'NONE',  ( -3.749999999999999556, 2.187500000000000444, -1.946699141100892927 ) ) ;
#12627=CARTESIAN_POINT ( 'NONE',  ( 3.749999999999998668, 2.187500000000000000, -5.053300858899108405 ) ) ;
#12632=CARTESIAN_POINT ( 'NONE',  ( -2.298097038856278918, 9.375000000000000000, -5.798097038856277585 ) ) ;
#12642=CARTESIAN_POINT ( 'NONE',  ( 3.249999999999999112, 10.81250000000000178, -2.153805922287439945 ) ) ;
#12644=CARTESIAN_POINT ( 'NONE',  ( -1.346194077712559389, 6.437500000000000888, -6.749999999999999112 ) ) ;
#12646=CARTESIAN_POINT ( 'NONE',  ( 1.553300858899105963, 2.062500000000000000, -7.250000000000000888 ) ) ;
#12650=CARTESIAN_POINT ( 'NONE',  ( 3.249999999999998668, 0.6875000000000000000, -4.846194077712560500 ) ) ;
#12652=CARTESIAN_POINT ( 'NONE',  ( 1.553300858899105963, 5.562500000000000000, -7.250000000000000888 ) ) ;
#12658=ORIENTED_EDGE ( 'NONE', *, *, #161, .F. ) ;
#12659=CARTESIAN_POINT ( 'NONE',  ( -1.346194077712558945, 1.562500000000000222, -0.2500000000000002220 ) ) ;
#12662=CARTESIAN_POINT ( 'NONE',  ( -3.750000000000000000, 9.687500000000000000, -1.946699141100893149 ) ) ;
#12663=CARTESIAN_POINT ( 'NONE',  ( -2.651650429449553314, 14.37500000000000000, -6.151650429449552426 ) ) ;
#12666=CARTESIAN_POINT ( 'NONE',  ( -1.346194077712558945, -0.4374999999999998890, -0.2500000000000002220 ) ) ;
#12676=CARTESIAN_POINT ( 'NONE',  ( 2.298097038856278029, 1.124999999999999778, -5.798097038856279362 ) ) ;
#12679=LINE ( 'NONE', #4408, #318 ) ;
#12681=CARTESIAN_POINT ( 'NONE',  ( -2.298097038856278918, 10.37500000000000000, -5.798097038856277585 ) ) ;
#12685=CARTESIAN_POINT ( 'NONE',  ( 1.346194077712561166, 14.43750000000000178, -0.2500000000000011102 ) ) ;
#12688=CARTESIAN_POINT ( 'NONE',  ( -4.592425496802573972E-16, 1.000000000000000000, -7.250000000000000000 ) ) ;
#12689=ADVANCED_FACE ( 'NONE', ( #6052 ), #10545, .F. ) ;
#12695=CARTESIAN_POINT ( 'NONE',  ( -2.298097038856278473, 7.125000000000000000, -1.201902961143720416 ) ) ;
#12702=CARTESIAN_POINT ( 'NONE',  ( -2.651650429449552870, 0.1250000000000000278, -0.8483495705504462414 ) ) ;
#12703=CARTESIAN_POINT ( 'NONE',  ( 1.346194077712558279, 14.06250000000000178, -6.750000000000000888 ) ) ;
#12706=CARTESIAN_POINT ( 'NONE',  ( -3.249999999999999112, 0.8124999999999997780, -4.846194077712558723 ) ) ;
#12707=EDGE_CURVE ( 'NONE', #11692, #9756, #12950, .T. ) ;
#12713=CARTESIAN_POINT ( 'NONE',  ( 3.249999999999998668, 4.687500000000000888, -4.846194077712560500 ) ) ;
#12717=VERTEX_POINT ( 'NONE', #3663 ) ;
#12720=CARTESIAN_POINT ( 'NONE',  ( -1.346194077712559167, 9.437500000000000000, -6.749999999999999112 ) ) ;
#12723=CARTESIAN_POINT ( 'NONE',  ( -2.651650429449552870, 8.624999999999998224, -0.8483495705504463524 ) ) ;
#12724=DIRECTION ( 'NONE',  ( -0.000000000000000000, -1.000000000000000000, -0.000000000000000000 ) ) ;
#12725=CARTESIAN_POINT ( 'NONE',  ( 0.000000000000000000, 0.5000000000000001110, 0.2500000000000002220 ) ) ;
#12726=CARTESIAN_POINT ( 'NONE',  ( 1.346194077712558279, 5.062500000000000000, -6.750000000000000888 ) ) ;
#12730=CARTESIAN_POINT ( 'NONE',  ( -3.980102097228897245E-16, 2.500000000000000000, -6.749999999999999112 ) ) ;
#12732=CARTESIAN_POINT ( 'NONE',  ( -4.592425496802573972E-16, 5.500000000000000000, -7.249999999999999112 ) ) ;
#12738=EDGE_CURVE ( 'NONE', #5493, #7860, #5061, .T. ) ;
#12742=CARTESIAN_POINT ( 'NONE',  ( -3.249999999999999112, 6.687500000000000888, -2.153805922287440833 ) ) ;
#12744=CARTESIAN_POINT ( 'NONE',  ( 2.651650429449553314, 11.37500000000000178, -0.8483495705504476847 ) ) ;
#12745=CARTESIAN_POINT ( 'NONE',  ( -2.651650429449552870, 14.12500000000000000, -0.8483495705504462414 ) ) ;
#12748=CARTESIAN_POINT ( 'NONE',  ( 0.000000000000000000, -0.2006112523677016091, 0.1491815183709511716 ) ) ;
#12749=CARTESIAN_POINT ( 'NONE',  ( -1.553300858899106629, 13.56250000000000000, 0.2500000000000002220 ) ) ;
#12758=CARTESIAN_POINT ( 'NONE',  ( 3.249999999999998224, 3.187500000000000444, -4.846194077712561388 ) ) ;
#12765=CARTESIAN_POINT ( 'NONE',  ( -3.249999999999999112, 13.68750000000000178, -2.153805922287440833 ) ) ;
#12767=CARTESIAN_POINT ( 'NONE',  ( 3.749999999999999112, 2.187500000000000000, -5.053300858899108405 ) ) ;
#12774=CARTESIAN_POINT ( 'NONE',  ( -3.249999999999999556, 7.312500000000000888, -4.846194077712557835 ) ) ;
#12780=CARTESIAN_POINT ( 'NONE',  ( 1.553300858899108849, 6.937500000000000000, 0.2499999999999993616 ) ) ;
#12781=CARTESIAN_POINT ( 'NONE',  ( -3.749999999999999556, 1.750000000000000000, -3.499999999999999112 ) ) ;
#12784=CARTESIAN_POINT ( 'NONE',  ( 1.346194077712558279, 2.062500000000000000, -6.750000000000000888 ) ) ;
#12785=CARTESIAN_POINT ( 'NONE',  ( -2.298097038856278918, 11.37500000000000000, -5.798097038856277585 ) ) ;
#12788=CARTESIAN_POINT ( 'NONE',  ( 1.346194077712560944, 4.937500000000001776, -0.2500000000000010547 ) ) ;
#12792=CARTESIAN_POINT ( 'NONE',  ( -0.3766621274091715987, 0.5000000000000000000, -0.1347136637304948981 ) ) ;
#12793=CARTESIAN_POINT ( 'NONE',  ( -1.346194077712559167, 10.43750000000000000, -6.749999999999999112 ) ) ;
#12797=CARTESIAN_POINT ( 'NONE',  ( -3.750000000000000000, 10.68750000000000178, -1.946699141100893149 ) ) ;
#12799=CARTESIAN_POINT ( 'NONE',  ( 0.000000000000000000, 1.500000000000000222, 0.2500000000000002220 ) ) ;
#12800=CARTESIAN_POINT ( 'NONE',  ( 1.346194077712561166, 7.437500000000000000, -0.2500000000000011102 ) ) ;
#12804=CARTESIAN_POINT ( 'NONE',  ( -2.298097038856278473, 1.125000000000000222, -1.201902961143720416 ) ) ;
#12805=CARTESIAN_POINT ( 'NONE',  ( 1.553300858899105963, 7.562500000000000000, -7.250000000000000888 ) ) ;
#12812=ORIENTED_EDGE ( 'NONE', *, *, #1681, .F. ) ;
#12813=CARTESIAN_POINT ( 'NONE',  ( 2.298097038856278029, 6.125000000000000000, -5.798097038856279362 ) ) ;
#12817=CARTESIAN_POINT ( 'NONE',  ( 0.000000000000000000, 9.500000000000001776, 0.2499999999999998057 ) ) ;
#12818=CARTESIAN_POINT ( 'NONE',  ( -1.553300858899106407, 12.06250000000000000, 0.2500000000000002220 ) ) ;
#12821=CARTESIAN_POINT ( 'NONE',  ( 2.298097038856279362, 7.875000000000000000, -1.201902961143720860 ) ) ;
#12822=CARTESIAN_POINT ( 'NONE',  ( 3.749999999999999112, 13.18750000000000000, -5.053300858899108405 ) ) ;
#12828=CARTESIAN_POINT ( 'NONE',  ( -3.980102097228897245E-16, 4.500000000000000888, -6.749999999999999112 ) ) ;
#12830=CARTESIAN_POINT ( 'NONE',  ( 2.298097038856278029, 2.125000000000000000, -5.798097038856279362 ) ) ;
#12838=CARTESIAN_POINT ( 'NONE',  ( -3.249999999999999112, 12.81250000000000178, -4.846194077712558723 ) ) ;
#12841=CARTESIAN_POINT ( 'NONE',  ( -4.592425496802573972E-16, 2.000000000000000000, -7.250000000000000000 ) ) ;
#12847=CARTESIAN_POINT ( 'NONE',  ( -2.298097038856278918, 14.37500000000000000, -5.798097038856277585 ) ) ;
#12854=CARTESIAN_POINT ( 'NONE',  ( -2.651650429449553314, 3.375000000000000000, -6.151650429449552426 ) ) ;
#12855=CARTESIAN_POINT ( 'NONE',  ( 0.000000000000000000, 3.500000000000000000, 0.2499999999999998057 ) ) ;
#12858=CARTESIAN_POINT ( 'NONE',  ( 2.298097038856278473, 14.62500000000000000, -5.798097038856279362 ) ) ;
#12864=CARTESIAN_POINT ( 'NONE',  ( 2.298097038856279362, 4.875000000000000000, -1.201902961143720860 ) ) ;
#12870=CARTESIAN_POINT ( 'NONE',  ( -2.298097038856278918, 12.37500000000000000, -5.798097038856277585 ) ) ;
#12874=CARTESIAN_POINT ( 'NONE',  ( 0.000000000000000000, 9.500000000000000000, 0.2500000000000002220 ) ) ;
#12876=CARTESIAN_POINT ( 'NONE',  ( -3.749999999999999556, 4.750000000000000888, -3.499999999999999112 ) ) ;
#12877=CARTESIAN_POINT ( 'NONE',  ( 0.000000000000000000, 7.500000000000000888, -0.2500000000000002220 ) ) ;
#12880=CARTESIAN_POINT ( 'NONE',  ( 3.249999999999999556, 1.750000000000000000, -3.500000000000000000 ) ) ;
#12882=CARTESIAN_POINT ( 'NONE',  ( -3.750000000000000000, 5.250000000000000000, -3.499999999999999112 ) ) ;
#12892=CARTESIAN_POINT ( 'NONE',  ( -3.249999999999999112, 8.687500000000003553, -2.153805922287440833 ) ) ;
#12895=CARTESIAN_POINT ( 'NONE',  ( -2.651650429449552870, 9.624999999999998224, -0.8483495705504467965 ) ) ;
#12896=CARTESIAN_POINT ( 'NONE',  ( -3.750000000000000000, 14.31250000000000000, -5.053300858899105741 ) ) ;
#12899=CARTESIAN_POINT ( 'NONE',  ( -2.298097038856279362, -0.1249999999999999029, -5.798097038856278473 ) ) ;
#12902=EDGE_CURVE ( 'NONE', #1425, #15209, #3903, .T. ) ;
#12906=CARTESIAN_POINT ( 'NONE',  ( 1.346194077712560944, 4.937500000000000888, -0.2500000000000011102 ) ) ;
#12908=CARTESIAN_POINT ( 'NONE',  ( -3.980102097228897738E-16, 6.000000000000000888, -6.749999999999999112 ) ) ;
#12911=B_SPLINE_CURVE_WITH_KNOTS ( 'NONE', 3,
 ( #260, #11301, #10071, #12465 ),
 .UNSPECIFIED., .F., .F.,
 ( 4, 4 ),
 ( 0.000000000000000000, 0.0003029267606473190228 ),
 .UNSPECIFIED. ) ;
#12914=CARTESIAN_POINT ( 'NONE',  ( 3.249999999999999556, 0.7500000000000000000, -3.500000000000000000 ) ) ;
#12915=CARTESIAN_POINT ( 'NONE',  ( 1.346194077712558279, 14.06250000000000178, -6.750000000000000888 ) ) ;
#12918=CARTESIAN_POINT ( 'NONE',  ( 1.553300858899109516, 3.437500000000000444, 0.2499999999999993616 ) ) ;
#12927=CARTESIAN_POINT ( 'NONE',  ( 3.249999999999999112, 11.81249999999999822, -2.153805922287439945 ) ) ;
#12933=CARTESIAN_POINT ( 'NONE',  ( 1.553300858899108849, 3.937500000000000000, 0.2499999999999993616 ) ) ;
#12935=CARTESIAN_POINT ( 'NONE',  ( 3.749999999999998668, 6.187500000000001776, -5.053300858899108405 ) ) ;
#12940=CARTESIAN_POINT ( 'NONE',  ( 0.000000000000000000, 1.500000000000000222, -0.2500000000000002220 ) ) ;
#12943=DIRECTION ( 'NONE',  ( 1.000000000000000000, 0.000000000000000000, 0.000000000000000000 ) ) ;
#12944=CARTESIAN_POINT ( 'NONE',  ( -1.346194077712559389, 4.062500000000000000, -0.2500000000000002220 ) ) ;
#12950=LINE ( 'NONE', #12792, #274 ) ;
#12955=CARTESIAN_POINT ( 'NONE',  ( 2.651650429449552870, 5.125000000000000888, -6.151650429449555091 ) ) ;
#12956=CARTESIAN_POINT ( 'NONE',  ( 1.346194077712558279, 8.062500000000001776, -6.750000000000000888 ) ) ;
#12957=ORIENTED_EDGE ( 'NONE', *, *, #2627, .F. ) ;
#12959=CARTESIAN_POINT ( 'NONE',  ( 3.249999999999998668, 3.687500000000000444, -4.846194077712560500 ) ) ;
#12960=CARTESIAN_POINT ( 'NONE',  ( -3.749999999999999556, 9.187500000000000000, -1.946699141100892927 ) ) ;
#12966=LINE ( 'NONE', #2446, #12208 ) ;
#12968=CARTESIAN_POINT ( 'NONE',  ( -2.298097038856278029, 8.625000000000000000, -1.201902961143720638 ) ) ;
#12969=ADVANCED_FACE ( 'NONE', ( #497 ), #10846, .F. ) ;
#12971=CARTESIAN_POINT ( 'NONE',  ( 0.000000000000000000, 11.50000000000000000, 0.2499999999999998057 ) ) ;
#12972=CARTESIAN_POINT ( 'NONE',  ( 0.3766621274091715987, 0.5000000000000000000, 0.1491815183709511716 ) ) ;
#12975=CARTESIAN_POINT ( 'NONE',  ( 3.249999999999998224, 0.3125000000000002220, -2.153805922287439945 ) ) ;
#12979=LINE ( 'NONE', #6003, #9892 ) ;
#12982=CARTESIAN_POINT ( 'NONE',  ( -2.298097038856278918, 4.375000000000000000, -5.798097038856277585 ) ) ;
#12984=CARTESIAN_POINT ( 'NONE',  ( 1.346194077712558279, 6.062500000000000888, -6.750000000000000888 ) ) ;
#12991=CARTESIAN_POINT ( 'NONE',  ( -1.346194077712559389, 0.06250000000000000000, -0.2500000000000002220 ) ) ;
#12992=CARTESIAN_POINT ( 'NONE',  ( -3.249999999999999112, 14.81250000000000355, -4.846194077712558723 ) ) ;
#12993=CARTESIAN_POINT ( 'NONE',  ( -3.750000000000000000, 4.312500000000000888, -5.053300858899105741 ) ) ;
#12995=CARTESIAN_POINT ( 'NONE',  ( -3.750000000000000000, 3.812500000000000888, -5.053300858899105741 ) ) ;
#13000=CARTESIAN_POINT ( 'NONE',  ( -3.249999999999999556, 11.31249999999999822, -4.846194077712557835 ) ) ;
#13007=CARTESIAN_POINT ( 'NONE',  ( -2.651650429449552870, 4.125000000000000000, -0.8483495705504462414 ) ) ;
#13008=CARTESIAN_POINT ( 'NONE',  ( -2.651650429449552870, 2.875000000000000000, -6.151650429449552426 ) ) ;
#13013=CARTESIAN_POINT ( 'NONE',  ( 3.249999999999999556, 13.75000000000000000, -3.500000000000000000 ) ) ;
#13018=CARTESIAN_POINT ( 'NONE',  ( 1.346194077712558057, 3.562500000000000444, -6.750000000000000000 ) ) ;
#13022=DIRECTION ( 'NONE',  ( 0.000000000000000000, 0.000000000000000000, -1.000000000000000000 ) ) ;
#13023=CARTESIAN_POINT ( 'NONE',  ( 3.249999999999998668, 14.68750000000000178, -4.846194077712560500 ) ) ;
#13027=CARTESIAN_POINT ( 'NONE',  ( 1.553300858899109516, 6.437500000000000888, 0.2499999999999993616 ) ) ;
#13028=CARTESIAN_POINT ( 'NONE',  ( -2.298097038856278029, 4.625000000000000888, -1.201902961143720638 ) ) ;
#13031=CARTESIAN_POINT ( 'NONE',  ( 3.249999999999999556, 2.750000000000000000, -3.500000000000000000 ) ) ;
#13040=CARTESIAN_POINT ( 'NONE',  ( -3.750000000000000000, 13.68750000000000178, -1.946699141100893149 ) ) ;
#13044=CARTESIAN_POINT ( 'NONE',  ( 3.249999999999998224, 4.187500000000000888, -4.846194077712561388 ) ) ;
#13047=CARTESIAN_POINT ( 'NONE',  ( -3.249999999999999556, 14.31250000000000000, -4.846194077712557835 ) ) ;
#13051=CARTESIAN_POINT ( 'NONE',  ( -3.980102097228897245E-16, 1.500000000000000000, -6.749999999999999112 ) ) ;
#13053=CARTESIAN_POINT ( 'NONE',  ( -2.298097038856279362, 5.875000000000001776, -5.798097038856278473 ) ) ;
#13058=CARTESIAN_POINT ( 'NONE',  ( -3.249999999999999556, 2.312500000000000888, -4.846194077712557835 ) ) ;
#13059=CARTESIAN_POINT ( 'NONE',  ( 1.553300858899109071, 2.437500000000000444, 0.2499999999999989175 ) ) ;
#13060=CARTESIAN_POINT ( 'NONE',  ( -3.750000000000000000, 6.312500000000000000, -5.053300858899105741 ) ) ;
#13062=CARTESIAN_POINT ( 'NONE',  ( 3.749999999999999556, 7.250000000000001776, -3.500000000000000444 ) ) ;
#13068=CARTESIAN_POINT ( 'NONE',  ( 0.000000000000000000, 11.00000000000000000, -0.2500000000000002220 ) ) ;
#13076=CARTESIAN_POINT ( 'NONE',  ( 0.000000000000000000, 4.000000000000000000, 0.2500000000000002220 ) ) ;
#13077=CARTESIAN_POINT ( 'NONE',  ( -3.750000000000000000, 4.812500000000000000, -5.053300858899105741 ) ) ;
#13078=AXIS2_PLACEMENT_3D ( 'NONE', #7596, #7676, #11236 ) ;
#13082=CARTESIAN_POINT ( 'NONE',  ( 1.346194077712558279, 6.062500000000000000, -6.750000000000000888 ) ) ;
#13086=CARTESIAN_POINT ( 'NONE',  ( -3.249999999999999556, 8.312500000000000000, -4.846194077712557835 ) ) ;
#13093=ORIENTED_EDGE ( 'NONE', *, *, #4492, .F. ) ;
#13098=EDGE_LOOP ( 'NONE', ( #1197, #5156, #6317, #10552 ) ) ;
#13099=CARTESIAN_POINT ( 'NONE',  ( -0.3766621274091715987, 0.2004420829692335482, 0.1491815183709511161 ) ) ;
#13100=CARTESIAN_POINT ( 'NONE',  ( -3.749999999999999556, 5.750000000000000888, -3.499999999999999112 ) ) ;
#13101=CARTESIAN_POINT ( 'NONE',  ( 3.249999999999998224, 12.31250000000000178, -2.153805922287439945 ) ) ;
#13105=CARTESIAN_POINT ( 'NONE',  ( -3.980102097228897245E-16, 8.500000000000000000, -6.749999999999999112 ) ) ;
#13118=CARTESIAN_POINT ( 'NONE',  ( -2.298097038856278473, 9.125000000000000000, -1.201902961143720416 ) ) ;
#13122=CARTESIAN_POINT ( 'NONE',  ( -3.749999999999999556, 14.75000000000000000, -3.499999999999999112 ) ) ;
#13126=CARTESIAN_POINT ( 'NONE',  ( 1.346194077712561166, 1.437500000000000000, -0.2500000000000011102 ) ) ;
#13134=CARTESIAN_POINT ( 'NONE',  ( 3.249999999999999556, 6.750000000000000000, -3.500000000000000000 ) ) ;
#13136=CARTESIAN_POINT ( 'NONE',  ( -3.249999999999999112, 0.6875000000000000000, -2.153805922287440833 ) ) ;
#13138=CARTESIAN_POINT ( 'NONE',  ( -3.249999999999999112, 5.812500000000000888, -4.846194077712558723 ) ) ;
#13143=CARTESIAN_POINT ( 'NONE',  ( 3.249999999999998668, 0.6875000000000000000, -4.846194077712560500 ) ) ;
#13144=CARTESIAN_POINT ( 'NONE',  ( 1.553300858899105963, 1.062500000000000444, -7.249999999999999112 ) ) ;
#13145=CARTESIAN_POINT ( 'NONE',  ( -2.651650429449553314, 7.375000000000000888, -6.151650429449552426 ) ) ;
#13148=CARTESIAN_POINT ( 'NONE',  ( 1.553300858899109516, 4.437500000000001776, 0.2499999999999993616 ) ) ;
#13154=CARTESIAN_POINT ( 'NONE',  ( -2.298097038856278473, 12.12500000000000000, -1.201902961143720416 ) ) ;
#13159=CARTESIAN_POINT ( 'NONE',  ( -3.750000000000000000, 8.687499999999998224, -1.946699141100893149 ) ) ;
#13163=CARTESIAN_POINT ( 'NONE',  ( -3.750000000000000000, 8.250000000000000000, -3.499999999999999112 ) ) ;
#13164=CARTESIAN_POINT ( 'NONE',  ( -3.749999999999999556, 3.750000000000000444, -3.499999999999999112 ) ) ;
#13168=CARTESIAN_POINT ( 'NONE',  ( 2.298097038856279362, 3.375000000000000444, -1.201902961143720860 ) ) ;
#13171=( NAMED_UNIT ( * ) PLANE_ANGLE_UNIT ( ) SI_UNIT ( $, .RADIAN. ) );
#13172=CARTESIAN_POINT ( 'NONE',  ( -3.980102097228897245E-16, 6.500000000000000888, -6.749999999999999112 ) ) ;
#13181=CARTESIAN_POINT ( 'NONE',  ( -3.249999999999999556, 14.25000000000000000, -3.499999999999999556 ) ) ;
#13185=CARTESIAN_POINT ( 'NONE',  ( 0.000000000000000000, 13.50000000000000355, 0.2499999999999998057 ) ) ;
#13186=CARTESIAN_POINT ( 'NONE',  ( -3.249999999999999112, 8.687499999999998224, -2.153805922287440833 ) ) ;
#13189=CARTESIAN_POINT ( 'NONE',  ( 2.298097038856279362, 7.875000000000000000, -1.201902961143720860 ) ) ;
#13200=CARTESIAN_POINT ( 'NONE',  ( 3.249999999999999556, 1.750000000000000000, -3.500000000000000000 ) ) ;
#13204=CARTESIAN_POINT ( 'NONE',  ( 1.553300858899105963, 15.06250000000000178, -7.249999999999999112 ) ) ;
#13209=CARTESIAN_POINT ( 'NONE',  ( -2.298097038856278029, 1.625000000000000000, -1.201902961143720638 ) ) ;
#13217=CARTESIAN_POINT ( 'NONE',  ( -3.249999999999999556, 8.250000000000000000, -3.499999999999999556 ) ) ;
#13219=CARTESIAN_POINT ( 'NONE',  ( 2.298097038856278473, 13.62500000000000000, -5.798097038856279362 ) ) ;
#13220=CARTESIAN_POINT ( 'NONE',  ( 3.249999999999999556, 8.250000000000000000, -3.500000000000000000 ) ) ;
#13222=CARTESIAN_POINT ( 'NONE',  ( 0.000000000000000000, -0.2105996885190176415, -0.1347136637304948981 ) ) ;
#13224=CARTESIAN_POINT ( 'NONE',  ( -2.298097038856278473, 2.125000000000000000, -1.201902961143720416 ) ) ;
#13225=CARTESIAN_POINT ( 'NONE',  ( -1.553300858899107073, 2.937500000000000444, -7.249999999999999112 ) ) ;
#13228=CARTESIAN_POINT ( 'NONE',  ( -3.750000000000000000, 5.312500000000000888, -5.053300858899105741 ) ) ;
#13231=CARTESIAN_POINT ( 'NONE',  ( -3.750000000000000000, 4.812500000000001776, -5.053300858899105741 ) ) ;
#13235=CARTESIAN_POINT ( 'NONE',  ( 3.249999999999999112, 10.81250000000000178, -2.153805922287439945 ) ) ;
#13237=CARTESIAN_POINT ( 'NONE',  ( 3.249999999999998668, 14.68750000000000000, -4.846194077712560500 ) ) ;
#13241=CARTESIAN_POINT ( 'NONE',  ( 2.651650429449552870, 11.12500000000000000, -6.151650429449555091 ) ) ;
#13242=VERTEX_POINT ( 'NONE', #2262 ) ;
#13245=CARTESIAN_POINT ( 'NONE',  ( 3.750000000000000000, 10.75000000000000000, -3.500000000000000444 ) ) ;
#13246=CARTESIAN_POINT ( 'NONE',  ( 0.000000000000000000, 6.500000000000000000, 0.2499999999999998057 ) ) ;
#13247=LINE ( 'NONE', #1254, #4046 ) ;
#13249=CARTESIAN_POINT ( 'NONE',  ( -3.249999999999999556, 5.750000000000000000, -3.500000000000000000 ) ) ;
#13251=CARTESIAN_POINT ( 'NONE',  ( -1.553300858899106629, 10.06250000000000000, 0.2500000000000002220 ) ) ;
#13254=CARTESIAN_POINT ( 'NONE',  ( 1.346194077712558057, 8.562500000000001776, -6.750000000000000000 ) ) ;
#13259=DIRECTION ( 'NONE',  ( -1.000000000000000000, 0.000000000000000000, -0.000000000000000000 ) ) ;
#13264=CARTESIAN_POINT ( 'NONE',  ( -3.750000000000000000, 11.81250000000000178, -5.053300858899105741 ) ) ;
#13265=CARTESIAN_POINT ( 'NONE',  ( 1.346194077712558279, 7.062499999999999112, -6.750000000000000888 ) ) ;
#13266=CARTESIAN_POINT ( 'NONE',  ( 1.346194077712558279, 9.062500000000000000, -6.750000000000000888 ) ) ;
#13269=CARTESIAN_POINT ( 'NONE',  ( -1.346194077712559389, 7.437500000000000888, -6.749999999999999112 ) ) ;
#13280=CARTESIAN_POINT ( 'NONE',  ( 1.346194077712561166, 14.43750000000000178, -0.2500000000000011102 ) ) ;
#13281=CARTESIAN_POINT ( 'NONE',  ( -3.749999999999999556, 13.31250000000000000, -5.053300858899104853 ) ) ;
#13283=CARTESIAN_POINT ( 'NONE',  ( 3.749999999999998668, 13.18750000000000000, -5.053300858899108405 ) ) ;
#13286=CARTESIAN_POINT ( 'NONE',  ( -1.346194077712558945, 2.562500000000000444, -0.2500000000000002220 ) ) ;
#13291=ORIENTED_EDGE ( 'NONE', *, *, #4932, .T. ) ;
#13293=CARTESIAN_POINT ( 'NONE',  ( -3.249999999999999556, 6.187500000000000000, -2.153805922287440833 ) ) ;
#13296=CARTESIAN_POINT ( 'NONE',  ( 0.000000000000000000, 13.00000000000000178, -0.2500000000000002220 ) ) ;
#13297=CARTESIAN_POINT ( 'NONE',  ( 0.000000000000000000, 10.49999999999999822, -0.2500000000000002220 ) ) ;
#13299=DIRECTION ( 'NONE',  ( -0.000000000000000000, -1.000000000000000000, -0.000000000000000000 ) ) ;
#13301=CARTESIAN_POINT ( 'NONE',  ( -1.346194077712559389, 5.062500000000001776, -0.2500000000000002220 ) ) ;
#13302=CARTESIAN_POINT ( 'NONE',  ( 1.346194077712558279, 15.06250000000000178, -6.750000000000000888 ) ) ;
#13304=CARTESIAN_POINT ( 'NONE',  ( 3.749999999999999556, 6.812500000000000000, -1.946699141100892261 ) ) ;
#13306=CARTESIAN_POINT ( 'NONE',  ( 3.749999999999999556, 5.250000000000000000, -3.500000000000000444 ) ) ;
#13315=CARTESIAN_POINT ( 'NONE',  ( 2.651650429449554203, 13.37500000000000000, -0.8483495705504471296 ) ) ;
#13319=CARTESIAN_POINT ( 'NONE',  ( 2.651650429449553759, 10.87500000000000178, -0.8483495705504471296 ) ) ;
#13320=CARTESIAN_POINT ( 'NONE',  ( -3.749999999999999556, 7.750000000000000888, -3.499999999999999112 ) ) ;
#13324=CARTESIAN_POINT ( 'NONE',  ( -1.346194077712559167, 5.937500000000000000, -6.749999999999999112 ) ) ;
#13327=CARTESIAN_POINT ( 'NONE',  ( -2.651650429449552870, 10.12500000000000000, -0.8483495705504462414 ) ) ;
#13330=CARTESIAN_POINT ( 'NONE',  ( -3.980102097228897245E-16, 9.500000000000000000, -6.749999999999999112 ) ) ;
#13341=CARTESIAN_POINT ( 'NONE',  ( 3.749999999999999556, 13.25000000000000178, -3.500000000000000444 ) ) ;
#13342=CARTESIAN_POINT ( 'NONE',  ( -3.980102097228897738E-16, 13.00000000000000000, -6.749999999999999112 ) ) ;
#13343=CARTESIAN_POINT ( 'NONE',  ( 1.346194077712558279, 11.06250000000000178, -6.750000000000000888 ) ) ;
#13346=CARTESIAN_POINT ( 'NONE',  ( -3.249999999999999556, 8.187500000000000000, -2.153805922287440833 ) ) ;
#13355=CARTESIAN_POINT ( 'NONE',  ( -3.980102097228897245E-16, 9.500000000000000000, -6.749999999999999112 ) ) ;
#13356=CARTESIAN_POINT ( 'NONE',  ( 0.000000000000000000, 0.000000000000000000, -0.2500000000000002220 ) ) ;
#13357=CARTESIAN_POINT ( 'NONE',  ( 3.750000000000000000, 11.75000000000000000, -3.500000000000000444 ) ) ;
#13362=CARTESIAN_POINT ( 'NONE',  ( 1.553300858899108849, 1.937500000000000000, 0.2499999999999993616 ) ) ;
#13366=CARTESIAN_POINT ( 'NONE',  ( 1.553300858899108849, 0.9375000000000000000, 0.2499999999999993616 ) ) ;
#13373=CARTESIAN_POINT ( 'NONE',  ( 3.249999999999999112, 6.812500000000000000, -2.153805922287439945 ) ) ;
#13375=CARTESIAN_POINT ( 'NONE',  ( 2.298097038856279362, 14.87500000000000178, -1.201902961143720860 ) ) ;
#13377=CARTESIAN_POINT ( 'NONE',  ( -3.249999999999999112, 10.68750000000000178, -2.153805922287440833 ) ) ;
#13381=CARTESIAN_POINT ( 'NONE',  ( -3.980102097228897245E-16, 3.500000000000000000, -6.749999999999999112 ) ) ;
#13382=CARTESIAN_POINT ( 'NONE',  ( -2.651650429449552870, 3.875000000000000444, -6.151650429449552426 ) ) ;
#13383=CARTESIAN_POINT ( 'NONE',  ( 1.553300858899105963, 10.56250000000000000, -7.250000000000000000 ) ) ;
#13386=CARTESIAN_POINT ( 'NONE',  ( 1.553300858899105963, 5.062500000000000000, -7.250000000000000888 ) ) ;
#13396=CARTESIAN_POINT ( 'NONE',  ( -1.346194077712558945, 0.5625000000000003331, -0.2500000000000002220 ) ) ;
#13400=CARTESIAN_POINT ( 'NONE',  ( 1.553300858899105963, 8.562500000000001776, -7.250000000000000888 ) ) ;
#13401=CARTESIAN_POINT ( 'NONE',  ( -2.651650429449552870, 6.875000000000000000, -6.151650429449552426 ) ) ;
#13406=CARTESIAN_POINT ( 'NONE',  ( -2.298097038856279362, 4.875000000000000000, -5.798097038856278473 ) ) ;
#13408=CARTESIAN_POINT ( 'NONE',  ( 3.750000000000000000, 10.75000000000000000, -3.500000000000000444 ) ) ;
#13414=CARTESIAN_POINT ( 'NONE',  ( 2.298097038856279362, 7.875000000000000000, -1.201902961143720860 ) ) ;
#13425=CARTESIAN_POINT ( 'NONE',  ( 1.553300858899105963, 12.06250000000000000, -7.249999999999999112 ) ) ;
#13427=CARTESIAN_POINT ( 'NONE',  ( -1.346194077712559167, 12.93750000000000178, -6.749999999999999112 ) ) ;
#13428=CARTESIAN_POINT ( 'NONE',  ( 1.346194077712561166, 11.43750000000000178, -0.2500000000000011102 ) ) ;
#13431=CARTESIAN_POINT ( 'NONE',  ( 1.346194077712560944, 8.937500000000001776, -0.2500000000000010547 ) ) ;
#13440=CARTESIAN_POINT ( 'NONE',  ( 0.000000000000000000, 2.000000000000000000, -0.2500000000000002220 ) ) ;
#13441=CARTESIAN_POINT ( 'NONE',  ( -3.749999999999999556, 13.18749999999999822, -1.946699141100892927 ) ) ;
#13446=CARTESIAN_POINT ( 'NONE',  ( 1.553300858899108849, 0.9374999999999998890, 0.2499999999999993616 ) ) ;
#13454=CARTESIAN_POINT ( 'NONE',  ( 2.298097038856278473, 8.625000000000000000, -5.798097038856279362 ) ) ;
#13456=CARTESIAN_POINT ( 'NONE',  ( -2.298097038856278918, 14.37500000000000000, -5.798097038856277585 ) ) ;
#13457=CARTESIAN_POINT ( 'NONE',  ( 3.249999999999999556, 9.249999999999998224, -3.500000000000000000 ) ) ;
#13461=CARTESIAN_POINT ( 'NONE',  ( 0.000000000000000000, 4.000000000000000000, -0.2500000000000002220 ) ) ;
#13463=CARTESIAN_POINT ( 'NONE',  ( 0.000000000000000000, 6.500000000000000000, 0.2499999999999998057 ) ) ;
#13464=CARTESIAN_POINT ( 'NONE',  ( 2.651650429449553759, 9.875000000000000000, -0.8483495705504471296 ) ) ;
#13467=CARTESIAN_POINT ( 'NONE',  ( -2.651650429449552870, 10.62500000000000000, -0.8483495705504463524 ) ) ;
#13472=CARTESIAN_POINT ( 'NONE',  ( -0.3766621274091725424, 0.2144981952514214973, -6.953972463291595574 ) ) ;
#13476=CARTESIAN_POINT ( 'NONE',  ( 3.749999999999999112, 14.18750000000000178, -5.053300858899108405 ) ) ;
#13480=CARTESIAN_POINT ( 'NONE',  ( -3.749999999999999556, 10.31250000000000000, -5.053300858899104853 ) ) ;
#13481=CARTESIAN_POINT ( 'NONE',  ( 0.000000000000000000, 8.500000000000000000, 0.2499999999999998057 ) ) ;
#13485=CARTESIAN_POINT ( 'NONE',  ( 0.000000000000000000, 6.500000000000000000, -0.2500000000000002220 ) ) ;
#13486=CARTESIAN_POINT ( 'NONE',  ( -3.749999999999999556, 14.18750000000000000, -1.946699141100892927 ) ) ;
#13491=CARTESIAN_POINT ( 'NONE',  ( -3.249999999999999556, 11.18749999999999822, -2.153805922287440833 ) ) ;
#13502=CARTESIAN_POINT ( 'NONE',  ( 3.749999999999998668, 13.18750000000000000, -5.053300858899108405 ) ) ;
#13503=CARTESIAN_POINT ( 'NONE',  ( 0.000000000000000000, 11.50000000000000000, -0.2500000000000002220 ) ) ;
#13504=ADVANCED_FACE ( 'NONE', ( #11266 ), #6399, .F. ) ;
#13505=CARTESIAN_POINT ( 'NONE',  ( 3.249999999999999556, 1.750000000000000000, -3.500000000000000000 ) ) ;
#13507=CARTESIAN_POINT ( 'NONE',  ( 1.346194077712560944, 12.93750000000000000, -0.2500000000000010547 ) ) ;
#13515=CARTESIAN_POINT ( 'NONE',  ( -3.249999999999999556, 1.312500000000000444, -4.846194077712557835 ) ) ;
#13516=CARTESIAN_POINT ( 'NONE',  ( -4.592425496802573972E-16, 12.50000000000000000, -7.249999999999999112 ) ) ;
#13521=CARTESIAN_POINT ( 'NONE',  ( -1.553300858899107295, 2.437500000000000444, -7.250000000000000000 ) ) ;
#13529=CARTESIAN_POINT ( 'NONE',  ( -3.249999999999999556, 9.312500000000000000, -4.846194077712557835 ) ) ;
#13531=CARTESIAN_POINT ( 'NONE',  ( -3.249999999999999556, 4.750000000000000000, -3.500000000000000000 ) ) ;
#13532=CARTESIAN_POINT ( 'NONE',  ( 1.346194077712561166, 11.43750000000000178, -0.2500000000000011102 ) ) ;
#13535=CARTESIAN_POINT ( 'NONE',  ( -2.298097038856278473, 6.125000000000000000, -1.201902961143720416 ) ) ;
#13536=CARTESIAN_POINT ( 'NONE',  ( -3.750000000000000000, 3.812500000000000000, -5.053300858899105741 ) ) ;
#13537=CARTESIAN_POINT ( 'NONE',  ( 3.749999999999999112, 8.687500000000000000, -5.053300858899108405 ) ) ;
#13540=CARTESIAN_POINT ( 'NONE',  ( -4.592425496802573972E-16, 11.00000000000000000, -7.250000000000000000 ) ) ;
#13547=CARTESIAN_POINT ( 'NONE',  ( -3.750000000000000000, 13.68750000000000178, -1.946699141100893149 ) ) ;
#13551=CARTESIAN_POINT ( 'NONE',  ( 2.651650429449553314, 8.375000000000000000, -0.8483495705504476847 ) ) ;
#13553=CARTESIAN_POINT ( 'NONE',  ( -1.346194077712559167, 6.937500000000001776, -6.749999999999999112 ) ) ;
#13554=CARTESIAN_POINT ( 'NONE',  ( 3.749999999999999556, 0.2500000000000001110, -3.500000000000000444 ) ) ;
#13559=CARTESIAN_POINT ( 'NONE',  ( -3.980102097228897245E-16, 11.50000000000000000, -6.749999999999999112 ) ) ;
#13560=CARTESIAN_POINT ( 'NONE',  ( -0.3766621274091715987, -0.2500000000000000000, -6.863050255469941519 ) ) ;
#13568=CARTESIAN_POINT ( 'NONE',  ( 3.749999999999998668, 1.687500000000000000, -5.053300858899107517 ) ) ;
#13569=CARTESIAN_POINT ( 'NONE',  ( 2.298097038856279362, 9.374999999999998224, -1.201902961143720860 ) ) ;
#13570=CARTESIAN_POINT ( 'NONE',  ( 2.298097038856278473, 0.6250000000000000000, -5.798097038856279362 ) ) ;
#13573=CARTESIAN_POINT ( 'NONE',  ( -2.298097038856278918, 11.37500000000000000, -5.798097038856277585 ) ) ;
#13577=CARTESIAN_POINT ( 'NONE',  ( 0.3766621274091715987, 0.5000000000000000000, -7.146945437571387671 ) ) ;
#13579=EDGE_CURVE ( 'NONE', #12717, #14660, #7192, .T. ) ;
#13583=CARTESIAN_POINT ( 'NONE',  ( 2.298097038856278473, 3.625000000000000000, -5.798097038856279362 ) ) ;
#13585=CARTESIAN_POINT ( 'NONE',  ( -1.553300858899106629, 12.06250000000000000, 0.2500000000000002220 ) ) ;
#13591=CARTESIAN_POINT ( 'NONE',  ( 3.749999999999999112, 1.812500000000000222, -1.946699141100892039 ) ) ;
#13599=ORIENTED_EDGE ( 'NONE', *, *, #3097, .F. ) ;
#13604=CARTESIAN_POINT ( 'NONE',  ( -0.3766621274091715987, 0.5000000000000000000, -6.863050255469941519 ) ) ;
#13605=CARTESIAN_POINT ( 'NONE',  ( -1.346194077712559167, 2.937500000000000444, -6.749999999999999112 ) ) ;
#13606=CARTESIAN_POINT ( 'NONE',  ( -3.980102097228897738E-16, 11.00000000000000000, -6.749999999999999112 ) ) ;
#13610=CARTESIAN_POINT ( 'NONE',  ( 3.249999999999999112, 4.812500000000000888, -2.153805922287439945 ) ) ;
#13611=CARTESIAN_POINT ( 'NONE',  ( 3.749999999999998668, 4.187500000000000888, -5.053300858899108405 ) ) ;
#13613=CARTESIAN_POINT ( 'NONE',  ( -3.750000000000000000, 9.187500000000000000, -1.946699141100892927 ) ) ;
#13617=CARTESIAN_POINT ( 'NONE',  ( -3.750000000000000000, 8.687499999999998224, -1.946699141100893149 ) ) ;
#13623=CARTESIAN_POINT ( 'NONE',  ( 3.249999999999999556, 0.7500000000000000000, -3.500000000000000000 ) ) ;
#13624=UNCERTAINTY_MEASURE_WITH_UNIT (LENGTH_MEASURE( 1.000000000000000082E-05 ), #892, 'distance_accuracy_value', 'NONE');
#13626=CARTESIAN_POINT ( 'NONE',  ( -2.298097038856278029, -0.3749999999999998890, -1.201902961143720638 ) ) ;
#13631=CARTESIAN_POINT ( 'NONE',  ( -3.249999999999999112, 8.812500000000001776, -4.846194077712558723 ) ) ;
#13633=CARTESIAN_POINT ( 'NONE',  ( -2.651650429449553314, 12.37500000000000000, -6.151650429449552426 ) ) ;
#13636=CARTESIAN_POINT ( 'NONE',  ( 0.000000000000000000, 13.00000000000000178, -0.2500000000000002220 ) ) ;
#13639=CARTESIAN_POINT ( 'NONE',  ( -1.346194077712559389, 7.062500000000000000, -0.2500000000000002220 ) ) ;
#13646=CARTESIAN_POINT ( 'NONE',  ( 1.553300858899108849, 2.937500000000000444, 0.2499999999999993616 ) ) ;
#13647=CARTESIAN_POINT ( 'NONE',  ( -3.249999999999999556, 14.75000000000000000, -3.500000000000000000 ) ) ;
#13648=CARTESIAN_POINT ( 'NONE',  ( -1.346194077712559167, 12.93750000000000178, -6.749999999999999112 ) ) ;
#13650=CARTESIAN_POINT ( 'NONE',  ( -3.980102097228897245E-16, 11.50000000000000000, -6.749999999999999112 ) ) ;
#13655=PLANE ( 'NONE',  #9926 ) ;
#13662=CARTESIAN_POINT ( 'NONE',  ( 3.249999999999999556, 2.750000000000000000, -3.500000000000000000 ) ) ;
#13664=CARTESIAN_POINT ( 'NONE',  ( 3.749999999999999112, 3.187500000000000444, -5.053300858899108405 ) ) ;
#13668=CARTESIAN_POINT ( 'NONE',  ( -4.592425496802573972E-16, 3.500000000000000000, -7.249999999999999112 ) ) ;
#13672=CARTESIAN_POINT ( 'NONE',  ( 1.553300858899108849, 1.937500000000000000, 0.2499999999999993616 ) ) ;
#13679=VECTOR ( 'NONE', #12724, 1000.000000000000000 ) ;
#13680=CARTESIAN_POINT ( 'NONE',  ( 2.298097038856278029, 3.125000000000000444, -5.798097038856279362 ) ) ;
#13685=CARTESIAN_POINT ( 'NONE',  ( 1.553300858899105963, 6.062500000000000000, -7.249999999999999112 ) ) ;
#13686=CARTESIAN_POINT ( 'NONE',  ( 1.553300858899105963, 8.562500000000000000, -7.250000000000000000 ) ) ;
#13689=CARTESIAN_POINT ( 'NONE',  ( 3.750000000000000000, 10.31250000000000000, -1.946699141100892705 ) ) ;
#13698=CARTESIAN_POINT ( 'NONE',  ( 1.346194077712561166, 3.437500000000000444, -0.2500000000000011102 ) ) ;
#13699=ORIENTED_EDGE ( 'NONE', *, *, #11469, .F. ) ;
#13707=CARTESIAN_POINT ( 'NONE',  ( -2.298097038856278029, 9.624999999999998224, -1.201902961143720638 ) ) ;
#13709=CARTESIAN_POINT ( 'NONE',  ( 3.749999999999998668, 12.68750000000000178, -5.053300858899107517 ) ) ;
#13712=CARTESIAN_POINT ( 'NONE',  ( -2.298097038856278918, 11.37500000000000000, -5.798097038856277585 ) ) ;
#13713=LINE ( 'NONE', #13560, #1908 ) ;
#13715=CARTESIAN_POINT ( 'NONE',  ( 3.249999999999999556, 7.750000000000000000, -3.500000000000000000 ) ) ;
#13721=CARTESIAN_POINT ( 'NONE',  ( 3.749999999999999112, 15.31250000000000355, -1.946699141100893149 ) ) ;
#13722=CARTESIAN_POINT ( 'NONE',  ( -3.750000000000000000, 0.8124999999999997780, -5.053300858899105741 ) ) ;
#13723=CARTESIAN_POINT ( 'NONE',  ( -2.298097038856278029, 13.62500000000000000, -1.201902961143720638 ) ) ;
#13725=CARTESIAN_POINT ( 'NONE',  ( -1.346194077712559389, 11.43750000000000000, -6.749999999999999112 ) ) ;
#13735=CARTESIAN_POINT ( 'NONE',  ( -2.298097038856278918, 6.375000000000000888, -5.798097038856277585 ) ) ;
#13737=CARTESIAN_POINT ( 'NONE',  ( -2.651650429449553314, -0.1249999999999999029, -6.151650429449552426 ) ) ;
#13741=CARTESIAN_POINT ( 'NONE',  ( -3.750000000000000000, 7.250000000000000000, -3.499999999999999112 ) ) ;
#13745=CARTESIAN_POINT ( 'NONE',  ( -2.651650429449552870, 3.125000000000000000, -0.8483495705504462414 ) ) ;
#13752=CARTESIAN_POINT ( 'NONE',  ( 2.298097038856278029, 5.125000000000000000, -5.798097038856279362 ) ) ;
#13755=CARTESIAN_POINT ( 'NONE',  ( -1.553300858899106629, 8.562500000000001776, 0.2499999999999998335 ) ) ;
#13756=CARTESIAN_POINT ( 'NONE',  ( 1.553300858899108849, 12.93750000000000355, 0.2499999999999993616 ) ) ;
#13760=CARTESIAN_POINT ( 'NONE',  ( -3.750000000000000000, 9.687500000000000000, -1.946699141100893149 ) ) ;
#13769=CARTESIAN_POINT ( 'NONE',  ( -3.980102097228897738E-16, 1.000000000000000000, -6.749999999999999112 ) ) ;
#13774=CARTESIAN_POINT ( 'NONE',  ( -2.298097038856278473, 10.12500000000000000, -1.201902961143720416 ) ) ;
#13777=CARTESIAN_POINT ( 'NONE',  ( -1.346194077712558945, 7.562500000000000888, -0.2500000000000002220 ) ) ;
#13778=CARTESIAN_POINT ( 'NONE',  ( -1.553300858899107073, -0.06249999999999988898, -7.249999999999999112 ) ) ;
#13779=CARTESIAN_POINT ( 'NONE',  ( 0.000000000000000000, -0.2105996885190176415, -0.1347136637304948981 ) ) ;
#13781=CARTESIAN_POINT ( 'NONE',  ( 2.298097038856279362, 12.87500000000000178, -1.201902961143720860 ) ) ;
#13785=CARTESIAN_POINT ( 'NONE',  ( -3.249999999999999556, 9.250000000000000000, -3.499999999999999556 ) ) ;
#13791=CARTESIAN_POINT ( 'NONE',  ( -3.750000000000000000, 1.250000000000000000, -3.499999999999999112 ) ) ;
#13792=CARTESIAN_POINT ( 'NONE',  ( -4.592425496802573972E-16, 2.000000000000000000, -7.250000000000000000 ) ) ;
#13793=CARTESIAN_POINT ( 'NONE',  ( -3.980102097228897738E-16, 13.00000000000000000, -6.749999999999999112 ) ) ;
#13795=CARTESIAN_POINT ( 'NONE',  ( -3.249999999999999556, 10.25000000000000000, -3.499999999999999556 ) ) ;
#13805=CARTESIAN_POINT ( 'NONE',  ( -3.249999999999999556, 12.18750000000000000, -2.153805922287440833 ) ) ;
#13807=CARTESIAN_POINT ( 'NONE',  ( 1.346194077712558057, 5.562500000000000000, -6.750000000000000000 ) ) ;
#13809=CARTESIAN_POINT ( 'NONE',  ( 1.553300858899105963, 1.062500000000000444, -7.250000000000000888 ) ) ;
#13810=EDGE_LOOP ( 'NONE', ( #2201, #6191, #4988, #6109, #11609, #12658, #4929, #8773 ) ) ;
#13812=CARTESIAN_POINT ( 'NONE',  ( -3.980102097228897245E-16, 0.5000000000000000000, -6.749999999999999112 ) ) ;
#13813=CARTESIAN_POINT ( 'NONE',  ( 3.749999999999998668, 5.687500000000000000, -5.053300858899107517 ) ) ;
#13821=CARTESIAN_POINT ( 'NONE',  ( 0.000000000000000000, 3.500000000000000000, -0.2500000000000002220 ) ) ;
#13823=EDGE_CURVE ( 'NONE', #4833, #5493, #6231, .T. ) ;
#13825=CARTESIAN_POINT ( 'NONE',  ( 2.651650429449552870, 10.12500000000000000, -6.151650429449553314 ) ) ;
#13826=CARTESIAN_POINT ( 'NONE',  ( -2.651650429449553314, 13.37500000000000000, -6.151650429449552426 ) ) ;
#13829=ORIENTED_EDGE ( 'NONE', *, *, #5371, .F. ) ;
#13831=CARTESIAN_POINT ( 'NONE',  ( 2.298097038856278029, 1.124999999999999778, -5.798097038856279362 ) ) ;
#13839=CARTESIAN_POINT ( 'NONE',  ( 0.000000000000000000, 0.000000000000000000, -0.2500000000000002220 ) ) ;
#13842=CARTESIAN_POINT ( 'NONE',  ( -1.346194077712558945, 2.562500000000000444, -0.2500000000000002220 ) ) ;
#13849=AXIS2_PLACEMENT_3D ( 'NONE', #11041, #4246, #5166 ) ;
#13853=CARTESIAN_POINT ( 'NONE',  ( 3.249999999999998224, 13.31250000000000178, -2.153805922287439945 ) ) ;
#13855=CARTESIAN_POINT ( 'NONE',  ( 3.750000000000000000, 3.312500000000000000, -1.946699141100892705 ) ) ;
#13859=CARTESIAN_POINT ( 'NONE',  ( -1.346194077712559389, 14.06249999999999822, -0.2500000000000002220 ) ) ;
#13862=CARTESIAN_POINT ( 'NONE',  ( 3.249999999999999556, 9.750000000000000000, -3.500000000000000000 ) ) ;
#13868=CARTESIAN_POINT ( 'NONE',  ( -2.651650429449553314, 2.375000000000000000, -6.151650429449552426 ) ) ;
#13869=CARTESIAN_POINT ( 'NONE',  ( -1.346194077712559167, 14.93750000000000000, -6.749999999999999112 ) ) ;
#13874=CARTESIAN_POINT ( 'NONE',  ( -1.346194077712558945, 0.5625000000000001110, -0.2500000000000002220 ) ) ;
#13881=CARTESIAN_POINT ( 'NONE',  ( -3.249999999999999556, 3.187500000000000000, -2.153805922287440833 ) ) ;
#13888=CARTESIAN_POINT ( 'NONE',  ( 3.249999999999998668, 9.687500000000000000, -4.846194077712560500 ) ) ;
#13890=ORIENTED_EDGE ( 'NONE', *, *, #12128, .T. ) ;
#13891=CARTESIAN_POINT ( 'NONE',  ( 2.298097038856278473, 2.625000000000000000, -5.798097038856279362 ) ) ;
#13893=CARTESIAN_POINT ( 'NONE',  ( -3.750000000000000000, 2.687500000000000888, -1.946699141100893149 ) ) ;
#13894=CARTESIAN_POINT ( 'NONE',  ( 1.346194077712561166, 6.437500000000000888, -0.2500000000000011102 ) ) ;
#13895=VERTEX_POINT ( 'NONE', #4370 ) ;
#13900=CARTESIAN_POINT ( 'NONE',  ( 2.298097038856278473, 11.62500000000000000, -5.798097038856279362 ) ) ;
#13901=CARTESIAN_POINT ( 'NONE',  ( -2.651650429449553314, 4.375000000000000000, -6.151650429449552426 ) ) ;
#13909=CARTESIAN_POINT ( 'NONE',  ( -3.249999999999999112, 5.687500000000000888, -2.153805922287440833 ) ) ;
#13912=CARTESIAN_POINT ( 'NONE',  ( -3.750000000000000000, 7.812500000000000000, -5.053300858899105741 ) ) ;
#13913=CARTESIAN_POINT ( 'NONE',  ( 3.750000000000000000, 14.75000000000000178, -3.500000000000000444 ) ) ;
#13917=CARTESIAN_POINT ( 'NONE',  ( -3.750000000000000000, 12.68750000000000000, -1.946699141100893149 ) ) ;
#13922=DIRECTION ( 'NONE',  ( 0.000000000000000000, -0.000000000000000000, 1.000000000000000000 ) ) ;
#13925=CARTESIAN_POINT ( 'NONE',  ( 1.346194077712558279, 1.062500000000000444, -6.750000000000000888 ) ) ;
#13932=CARTESIAN_POINT ( 'NONE',  ( 3.249999999999998224, 12.31250000000000178, -2.153805922287439945 ) ) ;
#13934=CARTESIAN_POINT ( 'NONE',  ( -3.750000000000000000, 2.687500000000000888, -1.946699141100893149 ) ) ;
#13935=CARTESIAN_POINT ( 'NONE',  ( 0.000000000000000000, 0.000000000000000000, -0.2500000000000002220 ) ) ;
#13940=CARTESIAN_POINT ( 'NONE',  ( 1.346194077712558057, 9.562500000000000000, -6.750000000000000000 ) ) ;
#13947=CARTESIAN_POINT ( 'NONE',  ( 0.000000000000000000, 5.000000000000000000, 0.2500000000000002220 ) ) ;
#13948=CARTESIAN_POINT ( 'NONE',  ( 1.553300858899109071, 1.437500000000000000, 0.2499999999999989175 ) ) ;
#13951=CARTESIAN_POINT ( 'NONE',  ( 2.298097038856278029, 2.125000000000000000, -5.798097038856279362 ) ) ;
#13956=CARTESIAN_POINT ( 'NONE',  ( 2.298097038856279362, 5.875000000000000000, -1.201902961143720860 ) ) ;
#13964=CARTESIAN_POINT ( 'NONE',  ( 3.249999999999998668, 12.68750000000000178, -4.846194077712560500 ) ) ;
#13967=CARTESIAN_POINT ( 'NONE',  ( -3.750000000000000000, 11.81250000000000178, -5.053300858899105741 ) ) ;
#13969=CARTESIAN_POINT ( 'NONE',  ( 2.651650429449554203, 1.375000000000000000, -0.8483495705504471296 ) ) ;
#13970=CARTESIAN_POINT ( 'NONE',  ( -1.346194077712558945, 7.562500000000000888, -0.2500000000000002220 ) ) ;
#13973=CARTESIAN_POINT ( 'NONE',  ( 2.298097038856279362, 4.875000000000000000, -1.201902961143720860 ) ) ;
#13974=CARTESIAN_POINT ( 'NONE',  ( 3.750000000000000000, 4.750000000000000000, -3.500000000000000444 ) ) ;
#13982=CARTESIAN_POINT ( 'NONE',  ( -1.346194077712558945, 6.562500000000000888, -0.2500000000000002220 ) ) ;
#13984=CARTESIAN_POINT ( 'NONE',  ( 2.651650429449552870, 8.125000000000000000, -6.151650429449553314 ) ) ;
#13985=CARTESIAN_POINT ( 'NONE',  ( -3.750000000000000000, 13.25000000000000000, -3.499999999999999112 ) ) ;
#13988=CARTESIAN_POINT ( 'NONE',  ( 0.000000000000000000, 12.50000000000000178, 0.2500000000000002220 ) ) ;
#13995=CARTESIAN_POINT ( 'NONE',  ( -3.249999999999999556, 4.312500000000000888, -4.846194077712557835 ) ) ;
#13997=CARTESIAN_POINT ( 'NONE',  ( 2.298097038856278029, 3.125000000000000444, -5.798097038856279362 ) ) ;
#14004=CARTESIAN_POINT ( 'NONE',  ( 1.346194077712558279, 11.06250000000000178, -6.750000000000000888 ) ) ;
#14006=CARTESIAN_POINT ( 'NONE',  ( -3.750000000000000000, 1.687500000000000222, -1.946699141100893149 ) ) ;
#14012=CARTESIAN_POINT ( 'NONE',  ( 2.298097038856278473, 13.62500000000000000, -5.798097038856279362 ) ) ;
#14017=DIRECTION ( 'NONE',  ( -1.000000000000000000, -0.000000000000000000, -0.000000000000000000 ) ) ;
#14018=CARTESIAN_POINT ( 'NONE',  ( -3.750000000000000000, 3.250000000000000444, -3.499999999999999112 ) ) ;
#14019=CARTESIAN_POINT ( 'NONE',  ( -3.749999999999999556, 2.750000000000000444, -3.499999999999999112 ) ) ;
#14022=CARTESIAN_POINT ( 'NONE',  ( -3.980102097228897738E-16, 2.000000000000000000, -6.749999999999999112 ) ) ;
#14026=CARTESIAN_POINT ( 'NONE',  ( 1.346194077712558057, 4.562500000000000888, -6.750000000000000000 ) ) ;
#14033=CARTESIAN_POINT ( 'NONE',  ( 3.249999999999998668, 10.68750000000000000, -4.846194077712560500 ) ) ;
#14036=CARTESIAN_POINT ( 'NONE',  ( 2.651650429449552870, 10.12500000000000000, -6.151650429449555091 ) ) ;
#14038=CARTESIAN_POINT ( 'NONE',  ( -2.651650429449552870, 7.625000000000001776, -0.8483495705504463524 ) ) ;
#14039=CARTESIAN_POINT ( 'NONE',  ( -2.298097038856278029, 6.625000000000000888, -1.201902961143720638 ) ) ;
#14042=CARTESIAN_POINT ( 'NONE',  ( 2.298097038856278473, 3.625000000000000000, -5.798097038856279362 ) ) ;
#14044=CARTESIAN_POINT ( 'NONE',  ( -1.553300858899106629, 5.062500000000001776, 0.2500000000000002220 ) ) ;
#14047=LINE ( 'NONE', #10558, #14856 ) ;
#14052=CARTESIAN_POINT ( 'NONE',  ( -3.249999999999999112, 8.812500000000001776, -4.846194077712558723 ) ) ;
#14055=CARTESIAN_POINT ( 'NONE',  ( -3.750000000000000000, 8.687500000000003553, -1.946699141100893149 ) ) ;
#14057=CARTESIAN_POINT ( 'NONE',  ( -3.750000000000000000, 13.31250000000000000, -5.053300858899105741 ) ) ;
#14061=CARTESIAN_POINT ( 'NONE',  ( 3.249999999999999556, 0.2500000000000001110, -3.500000000000000000 ) ) ;
#14067=CARTESIAN_POINT ( 'NONE',  ( 3.249999999999999556, 1.750000000000000000, -3.500000000000000000 ) ) ;
#14069=CARTESIAN_POINT ( 'NONE',  ( -2.298097038856279362, 4.875000000000000000, -5.798097038856278473 ) ) ;
#14075=FACE_OUTER_BOUND ( 'NONE', #4583, .T. ) ;
#14076=CARTESIAN_POINT ( 'NONE',  ( 1.346194077712558279, 12.06250000000000000, -6.750000000000000888 ) ) ;
#14077=VECTOR ( 'NONE', #5731, 1000.000000000000000 ) ;
#14079=CARTESIAN_POINT ( 'NONE',  ( 3.749999999999999556, 3.250000000000000000, -3.500000000000000444 ) ) ;
#14085=CARTESIAN_POINT ( 'NONE',  ( 1.346194077712558057, 14.56250000000000000, -6.750000000000000000 ) ) ;
#14094=CARTESIAN_POINT ( 'NONE',  ( -4.592425496802573972E-16, 3.500000000000000000, -7.249999999999999112 ) ) ;
#14095=CARTESIAN_POINT ( 'NONE',  ( -4.592425496802573972E-16, 5.999999999999999112, -7.250000000000000000 ) ) ;
#14098=CARTESIAN_POINT ( 'NONE',  ( -3.249999999999999556, 14.18750000000000000, -2.153805922287440833 ) ) ;
#14105=CARTESIAN_POINT ( 'NONE',  ( 3.249999999999998668, 3.687500000000000444, -4.846194077712560500 ) ) ;
#14111=CARTESIAN_POINT ( 'NONE',  ( -3.249999999999999556, 13.18750000000000000, -2.153805922287440833 ) ) ;
#14116=CARTESIAN_POINT ( 'NONE',  ( -4.592425496802573972E-16, 6.000000000000000888, -7.250000000000000000 ) ) ;
#14117=CARTESIAN_POINT ( 'NONE',  ( 3.249999999999998224, 6.187500000000001776, -4.846194077712561388 ) ) ;
#14120=CARTESIAN_POINT ( 'NONE',  ( 2.298097038856278473, 1.625000000000000222, -5.798097038856279362 ) ) ;
#14122=CARTESIAN_POINT ( 'NONE',  ( 1.553300858899105963, 10.56250000000000000, -7.250000000000000888 ) ) ;
#14131=CARTESIAN_POINT ( 'NONE',  ( -3.249999999999999112, 7.812500000000000000, -4.846194077712558723 ) ) ;
#14134=CARTESIAN_POINT ( 'NONE',  ( -4.592425496802573972E-16, 12.00000000000000178, -7.250000000000000000 ) ) ;
#14138=CARTESIAN_POINT ( 'NONE',  ( 3.749999999999999556, 14.25000000000000178, -3.500000000000000444 ) ) ;
#14141=CARTESIAN_POINT ( 'NONE',  ( 2.298097038856279362, 14.87500000000000178, -1.201902961143720860 ) ) ;
#14146=CARTESIAN_POINT ( 'NONE',  ( 2.298097038856278473, 1.625000000000000222, -5.798097038856279362 ) ) ;
#14150=CARTESIAN_POINT ( 'NONE',  ( 2.298097038856278029, 8.125000000000000000, -5.798097038856279362 ) ) ;
#14156=CARTESIAN_POINT ( 'NONE',  ( 2.298097038856279362, 0.8750000000000000000, -1.201902961143720860 ) ) ;
#14157=CARTESIAN_POINT ( 'NONE',  ( 1.346194077712561166, 12.43750000000000000, -0.2500000000000011102 ) ) ;
#14158=CARTESIAN_POINT ( 'NONE',  ( 0.000000000000000000, 6.000000000000000000, 0.2500000000000002220 ) ) ;
#14159=CARTESIAN_POINT ( 'NONE',  ( 0.2518559594811072277, 0.3124778193275194460, -7.146945437571262438 ) ) ;
#14160=CARTESIAN_POINT ( 'NONE',  ( -2.651650429449552870, 3.625000000000000888, -0.8483495705504463524 ) ) ;
#14166=CARTESIAN_POINT ( 'NONE',  ( 3.249999999999999556, 10.75000000000000000, -3.500000000000000000 ) ) ;
#14174=CARTESIAN_POINT ( 'NONE',  ( 1.553300858899105963, 5.562500000000000000, -7.250000000000000888 ) ) ;
#14176=CARTESIAN_POINT ( 'NONE',  ( 2.651650429449552870, 3.125000000000000444, -6.151650429449553314 ) ) ;
#14178=ORIENTED_EDGE ( 'NONE', *, *, #1492, .T. ) ;
#14179=CARTESIAN_POINT ( 'NONE',  ( -3.980102097228897245E-16, 13.50000000000000000, -6.749999999999999112 ) ) ;
#14183=CARTESIAN_POINT ( 'NONE',  ( -1.346194077712559389, 3.437500000000000000, -6.749999999999999112 ) ) ;
#14190=CARTESIAN_POINT ( 'NONE',  ( 0.000000000000000000, 15.00000000000000000, -0.2500000000000002220 ) ) ;
#14194=CARTESIAN_POINT ( 'NONE',  ( -2.651650429449553314, 5.875000000000001776, -6.151650429449552426 ) ) ;
#14195=CARTESIAN_POINT ( 'NONE',  ( -3.249999999999999556, 6.750000000000001776, -3.500000000000000000 ) ) ;
#14199=CARTESIAN_POINT ( 'NONE',  ( -3.249999999999999556, 2.312500000000000888, -4.846194077712557835 ) ) ;
#14207=CARTESIAN_POINT ( 'NONE',  ( 1.553300858899109071, 13.43750000000000355, 0.2499999999999989175 ) ) ;
#14209=EDGE_CURVE ( 'NONE', #2112, #4560, #15143, .T. ) ;
#14212=CARTESIAN_POINT ( 'NONE',  ( -3.980102097228897738E-16, 4.000000000000000888, -6.749999999999999112 ) ) ;
#14221=CARTESIAN_POINT ( 'NONE',  ( -3.249999999999999556, 3.187500000000000444, -2.153805922287440833 ) ) ;
#14223=CARTESIAN_POINT ( 'NONE',  ( 2.298097038856278029, 6.125000000000000000, -5.798097038856279362 ) ) ;
#14229=CARTESIAN_POINT ( 'NONE',  ( -3.249999999999999556, 2.187500000000000444, -2.153805922287440833 ) ) ;
#14230=CARTESIAN_POINT ( 'NONE',  ( 1.553300858899105963, 2.062500000000000000, -7.249999999999999112 ) ) ;
#14231=CARTESIAN_POINT ( 'NONE',  ( 3.749999999999999556, 3.812500000000000000, -1.946699141100892261 ) ) ;
#14233=CARTESIAN_POINT ( 'NONE',  ( -3.750000000000000000, 7.687500000000000888, -1.946699141100893149 ) ) ;
#14238=CARTESIAN_POINT ( 'NONE',  ( -3.249999999999999556, 13.31250000000000000, -4.846194077712557835 ) ) ;
#14245=CARTESIAN_POINT ( 'NONE',  ( 3.750000000000000000, 4.750000000000000000, -3.500000000000000444 ) ) ;
#14246=CARTESIAN_POINT ( 'NONE',  ( 3.749999999999999556, 4.249999999999999112, -3.500000000000000444 ) ) ;
#14250=CARTESIAN_POINT ( 'NONE',  ( -3.249999999999999112, 5.687500000000000888, -2.153805922287440833 ) ) ;
#14258=CARTESIAN_POINT ( 'NONE',  ( -2.298097038856278918, 7.375000000000000888, -5.798097038856277585 ) ) ;
#14265=CARTESIAN_POINT ( 'NONE',  ( -2.298097038856278918, 13.37500000000000000, -5.798097038856277585 ) ) ;
#14269=CARTESIAN_POINT ( 'NONE',  ( 1.553300858899105963, 5.062500000000000000, -7.250000000000000888 ) ) ;
#14270=CARTESIAN_POINT ( 'NONE',  ( -3.249999999999999112, 8.812500000000001776, -4.846194077712558723 ) ) ;
#14273=CARTESIAN_POINT ( 'NONE',  ( 3.249999999999998668, 1.687500000000000000, -4.846194077712560500 ) ) ;
#14280=CARTESIAN_POINT ( 'NONE',  ( -1.553300858899106629, 14.56250000000000000, 0.2499999999999998335 ) ) ;
#14284=CARTESIAN_POINT ( 'NONE',  ( -2.298097038856278029, 2.625000000000000000, -1.201902961143720638 ) ) ;
#14287=CARTESIAN_POINT ( 'NONE',  ( 0.000000000000000000, 15.00000000000000000, -0.2500000000000002220 ) ) ;
#14292=CARTESIAN_POINT ( 'NONE',  ( 2.298097038856279362, 2.875000000000000000, -1.201902961143720860 ) ) ;
#14295=CARTESIAN_POINT ( 'NONE',  ( -3.249999999999999556, 12.25000000000000000, -3.499999999999999556 ) ) ;
#14296=CARTESIAN_POINT ( 'NONE',  ( -3.980102097228897245E-16, 11.50000000000000000, -6.749999999999999112 ) ) ;
#14297=CARTESIAN_POINT ( 'NONE',  ( -3.249999999999999556, 5.750000000000000888, -3.500000000000000000 ) ) ;
#14302=CARTESIAN_POINT ( 'NONE',  ( -1.346194077712559389, 0.4375000000000000555, -6.749999999999999112 ) ) ;
#14303=CARTESIAN_POINT ( 'NONE',  ( -4.592425496802573972E-16, 1.000000000000000000, -7.250000000000000000 ) ) ;
#14304=CARTESIAN_POINT ( 'NONE',  ( 1.553300858899105963, 3.562500000000000000, -7.250000000000000000 ) ) ;
#14306=CARTESIAN_POINT ( 'NONE',  ( 3.750000000000000000, 4.312500000000000000, -1.946699141100892705 ) ) ;
#14311=CARTESIAN_POINT ( 'NONE',  ( -2.298097038856278473, 14.12500000000000000, -1.201902961143720416 ) ) ;
#14317=CARTESIAN_POINT ( 'NONE',  ( 1.553300858899109516, 10.43750000000000178, 0.2499999999999993616 ) ) ;
#14321=CARTESIAN_POINT ( 'NONE',  ( -1.553300858899107295, 10.43750000000000000, -7.250000000000000000 ) ) ;
#14322=CARTESIAN_POINT ( 'NONE',  ( 3.749999999999999112, 3.312500000000000000, -1.946699141100893149 ) ) ;
#14327=CARTESIAN_POINT ( 'NONE',  ( 0.000000000000000000, 4.499999999999999112, -0.2500000000000002220 ) ) ;
#14333=CARTESIAN_POINT ( 'NONE',  ( 3.249999999999998668, 9.687500000000000000, -4.846194077712560500 ) ) ;
#14340=CARTESIAN_POINT ( 'NONE',  ( 3.249999999999999556, 13.75000000000000000, -3.500000000000000000 ) ) ;
#14345=CARTESIAN_POINT ( 'NONE',  ( 2.651650429449554203, 4.375000000000000888, -0.8483495705504471296 ) ) ;
#14347=CARTESIAN_POINT ( 'NONE',  ( -2.298097038856278029, 9.624999999999998224, -1.201902961143720638 ) ) ;
#14353=CARTESIAN_POINT ( 'NONE',  ( -3.249999999999999556, 5.250000000000000000, -3.499999999999999556 ) ) ;
#14362=EDGE_LOOP ( 'NONE', ( #6281, #13291, #10268 ) ) ;
#14363=CARTESIAN_POINT ( 'NONE',  ( 2.298097038856279362, 9.875000000000000000, -1.201902961143720860 ) ) ;
#14364=CARTESIAN_POINT ( 'NONE',  ( 0.000000000000000000, 13.50000000000000178, -0.2500000000000002220 ) ) ;
#14369=CARTESIAN_POINT ( 'NONE',  ( 1.553300858899105963, 12.06250000000000000, -7.249999999999999112 ) ) ;
#14372=CARTESIAN_POINT ( 'NONE',  ( 3.249999999999998224, 3.187500000000000444, -4.846194077712561388 ) ) ;
#14380=CARTESIAN_POINT ( 'NONE',  ( 1.346194077712560944, 8.937500000000001776, -0.2500000000000011102 ) ) ;
#14382=CARTESIAN_POINT ( 'NONE',  ( -2.298097038856278918, 12.37500000000000000, -5.798097038856277585 ) ) ;
#14383=CARTESIAN_POINT ( 'NONE',  ( -1.346194077712559167, 7.937500000000001776, -6.749999999999999112 ) ) ;
#14385=DIRECTION ( 'NONE',  ( 0.000000000000000000, 0.000000000000000000, 1.000000000000000000 ) ) ;
#14387=CARTESIAN_POINT ( 'NONE',  ( 3.249999999999999556, 2.750000000000000000, -3.500000000000000000 ) ) ;
#14388=CARTESIAN_POINT ( 'NONE',  ( -2.651650429449552870, 0.8750000000000000000, -6.151650429449552426 ) ) ;
#14389=CARTESIAN_POINT ( 'NONE',  ( -2.651650429449553314, 5.375000000000000000, -6.151650429449552426 ) ) ;
#14392=CARTESIAN_POINT ( 'NONE',  ( -3.750000000000000000, 6.687500000000000888, -1.946699141100893149 ) ) ;
#14395=AXIS2_PLACEMENT_3D ( 'NONE', #3960, #8822, #7506 ) ;
#14398=CARTESIAN_POINT ( 'NONE',  ( -0.3766621274091715987, 0.5000000000000000000, 0.1491815183709511716 ) ) ;
#14403=CARTESIAN_POINT ( 'NONE',  ( -1.553300858899107073, 10.93750000000000000, -7.249999999999999112 ) ) ;
#14407=CARTESIAN_POINT ( 'NONE',  ( 2.651650429449552870, 10.62500000000000000, -6.151650429449554203 ) ) ;
#14408=CARTESIAN_POINT ( 'NONE',  ( 2.651650429449552870, 8.125000000000000000, -6.151650429449553314 ) ) ;
#14410=ORIENTED_EDGE ( 'NONE', *, *, #5243, .F. ) ;
#14413=CARTESIAN_POINT ( 'NONE',  ( 3.249999999999999556, 5.249999999999999112, -3.500000000000000000 ) ) ;
#14415=CARTESIAN_POINT ( 'NONE',  ( 1.553300858899105963, 8.562500000000001776, -7.250000000000000888 ) ) ;
#14419=CARTESIAN_POINT ( 'NONE',  ( -3.249999999999999556, 7.312500000000000888, -4.846194077712557835 ) ) ;
#14432=CARTESIAN_POINT ( 'NONE',  ( -1.553300858899106629, 14.56250000000000000, 0.2499999999999998335 ) ) ;
#14433=CARTESIAN_POINT ( 'NONE',  ( -3.249999999999999112, 6.812500000000000000, -4.846194077712558723 ) ) ;
#14435=CARTESIAN_POINT ( 'NONE',  ( -2.298097038856279362, 11.87500000000000000, -5.798097038856278473 ) ) ;
#14438=CARTESIAN_POINT ( 'NONE',  ( 2.298097038856278473, 5.625000000000000000, -5.798097038856279362 ) ) ;
#14449=CARTESIAN_POINT ( 'NONE',  ( -2.298097038856278918, 0.3750000000000000000, -5.798097038856277585 ) ) ;
#14451=CARTESIAN_POINT ( 'NONE',  ( 1.553300858899105963, 11.56249999999999822, -7.250000000000000888 ) ) ;
#14453=CARTESIAN_POINT ( 'NONE',  ( 0.000000000000000000, 13.50000000000000355, 0.2499999999999998057 ) ) ;
#14456=CARTESIAN_POINT ( 'NONE',  ( -3.249999999999999112, 1.687500000000000222, -2.153805922287440833 ) ) ;
#14460=DIRECTION ( 'NONE',  ( 0.000000000000000000, 0.000000000000000000, 1.000000000000000000 ) ) ;
#14462=ORIENTED_EDGE ( 'NONE', *, *, #12738, .F. ) ;
#14464=CARTESIAN_POINT ( 'NONE',  ( 0.000000000000000000, 9.000000000000001776, -0.2500000000000002220 ) ) ;
#14466=CARTESIAN_POINT ( 'NONE',  ( 3.249999999999998668, 14.68750000000000000, -4.846194077712560500 ) ) ;
#14467=CARTESIAN_POINT ( 'NONE',  ( -3.249999999999999556, 9.750000000000000000, -3.500000000000000000 ) ) ;
#14469=CARTESIAN_POINT ( 'NONE',  ( -0.2510664901725777054, -0.2041261725989376163, -0.1347136637304948981 ) ) ;
#14471=CARTESIAN_POINT ( 'NONE',  ( -1.346194077712559389, 3.437500000000000000, -6.749999999999999112 ) ) ;
#14472=CARTESIAN_POINT ( 'NONE',  ( 3.749999999999998668, 2.187500000000000000, -5.053300858899108405 ) ) ;
#14473=CARTESIAN_POINT ( 'NONE',  ( -4.592425496802573972E-16, 5.500000000000000000, -7.249999999999999112 ) ) ;
#14475=CARTESIAN_POINT ( 'NONE',  ( -4.592425496802573972E-16, 8.000000000000000000, -7.250000000000000000 ) ) ;
#14485=CARTESIAN_POINT ( 'NONE',  ( 2.651650429449554203, 10.37500000000000000, -0.8483495705504471296 ) ) ;
#14489=CARTESIAN_POINT ( 'NONE',  ( -1.553300858899106629, 9.062499999999998224, 0.2500000000000002220 ) ) ;
#14490=CARTESIAN_POINT ( 'NONE',  ( -2.651650429449552870, 7.625000000000000000, -0.8483495705504467965 ) ) ;
#14494=CARTESIAN_POINT ( 'NONE',  ( -3.980102097228897738E-16, 4.000000000000000000, -6.749999999999999112 ) ) ;
#14495=CARTESIAN_POINT ( 'NONE',  ( -3.750000000000000000, 10.25000000000000000, -3.499999999999999112 ) ) ;
#14498=CARTESIAN_POINT ( 'NONE',  ( 3.249999999999998668, 7.687500000000000000, -4.846194077712560500 ) ) ;
#14510=CARTESIAN_POINT ( 'NONE',  ( -3.749999999999999556, 11.75000000000000178, -3.499999999999999112 ) ) ;
#14511=CARTESIAN_POINT ( 'NONE',  ( 1.346194077712558279, 11.06250000000000178, -6.750000000000000888 ) ) ;
#14512=CARTESIAN_POINT ( 'NONE',  ( -3.249999999999999556, 9.750000000000000000, -3.500000000000000000 ) ) ;
#14516=CARTESIAN_POINT ( 'NONE',  ( 3.249999999999999556, 7.750000000000000000, -3.500000000000000000 ) ) ;
#14523=CARTESIAN_POINT ( 'NONE',  ( 0.000000000000000000, 10.00000000000000000, -0.2500000000000002220 ) ) ;
#14524=CARTESIAN_POINT ( 'NONE',  ( -2.298097038856279362, 13.87500000000000178, -5.798097038856278473 ) ) ;
#14525=CARTESIAN_POINT ( 'NONE',  ( 2.651650429449553759, 14.87500000000000178, -0.8483495705504471296 ) ) ;
#14528=CARTESIAN_POINT ( 'NONE',  ( -2.651650429449553314, 1.375000000000000000, -6.151650429449552426 ) ) ;
#14530=CARTESIAN_POINT ( 'NONE',  ( -0.3766621274091715987, 0.2398196381212478467, -0.1347136637304948426 ) ) ;
#14538=CARTESIAN_POINT ( 'NONE',  ( 2.298097038856279362, 6.875000000000000000, -1.201902961143720860 ) ) ;
#14540=CARTESIAN_POINT ( 'NONE',  ( -3.249999999999999556, 12.18750000000000000, -2.153805922287440833 ) ) ;
#14541=EDGE_CURVE ( 'NONE', #11999, #5680, #12160, .T. ) ;
#14542=CARTESIAN_POINT ( 'NONE',  ( -1.346194077712558945, 10.56249999999999822, -0.2500000000000002220 ) ) ;
#14545=CARTESIAN_POINT ( 'NONE',  ( -2.298097038856278918, 0.3750000000000000000, -5.798097038856277585 ) ) ;
#14548=CARTESIAN_POINT ( 'NONE',  ( -2.298097038856278473, 4.125000000000000000, -1.201902961143720416 ) ) ;
#14549=CARTESIAN_POINT ( 'NONE',  ( 3.749999999999999556, 3.250000000000000000, -3.500000000000000444 ) ) ;
#14550=CARTESIAN_POINT ( 'NONE',  ( -3.750000000000000000, 10.18750000000000000, -1.946699141100892927 ) ) ;
#14552=CARTESIAN_POINT ( 'NONE',  ( -3.749999999999999556, 7.750000000000000888, -3.499999999999999112 ) ) ;
#14557=CARTESIAN_POINT ( 'NONE',  ( 2.298097038856278473, 14.62500000000000000, -5.798097038856279362 ) ) ;
#14560=CARTESIAN_POINT ( 'NONE',  ( -4.592425496802573972E-16, 13.00000000000000000, -7.250000000000000000 ) ) ;
#14564=CARTESIAN_POINT ( 'NONE',  ( -2.651650429449552870, 9.125000000000000000, -0.8483495705504462414 ) ) ;
#14565=CARTESIAN_POINT ( 'NONE',  ( -2.651650429449552870, 7.874999999999999112, -6.151650429449552426 ) ) ;
#14568=CARTESIAN_POINT ( 'NONE',  ( 3.249999999999998224, 6.312500000000000000, -2.153805922287439945 ) ) ;
#14569=CARTESIAN_POINT ( 'NONE',  ( 3.749999999999998668, 11.68750000000000000, -5.053300858899107517 ) ) ;
#14572=CARTESIAN_POINT ( 'NONE',  ( -1.346194077712559389, 9.437500000000000000, -6.749999999999999112 ) ) ;
#14584=CARTESIAN_POINT ( 'NONE',  ( 2.651650429449553314, 13.37500000000000000, -0.8483495705504476847 ) ) ;
#14585=CARTESIAN_POINT ( 'NONE',  ( -1.346194077712558945, 11.56250000000000178, -0.2500000000000002220 ) ) ;
#14586=CARTESIAN_POINT ( 'NONE',  ( 2.298097038856278029, 12.12500000000000000, -5.798097038856279362 ) ) ;
#14589=CARTESIAN_POINT ( 'NONE',  ( 3.249999999999999112, 8.812500000000000000, -2.153805922287439945 ) ) ;
#14599=VECTOR ( 'NONE', #6132, 1000.000000000000000 ) ;
#14601=CARTESIAN_POINT ( 'NONE',  ( 3.249999999999999112, 0.8125000000000001110, -2.153805922287439945 ) ) ;
#14602=CARTESIAN_POINT ( 'NONE',  ( -2.651650429449552870, 12.12500000000000000, -0.8483495705504462414 ) ) ;
#14607=CARTESIAN_POINT ( 'NONE',  ( 1.553300858899105963, 2.562500000000000444, -7.250000000000000888 ) ) ;
#14612=CARTESIAN_POINT ( 'NONE',  ( -4.592425496802573972E-16, 1.500000000000000000, -7.249999999999999112 ) ) ;
#14619=CARTESIAN_POINT ( 'NONE',  ( -3.249999999999999556, 8.187500000000000000, -2.153805922287440833 ) ) ;
#14621=CARTESIAN_POINT ( 'NONE',  ( 3.249999999999999556, 13.75000000000000000, -3.500000000000000000 ) ) ;
#14623=CARTESIAN_POINT ( 'NONE',  ( 1.346194077712558279, 11.06250000000000178, -6.750000000000000888 ) ) ;
#14627=CARTESIAN_POINT ( 'NONE',  ( -3.249999999999999556, 3.312500000000000000, -4.846194077712557835 ) ) ;
#14628=CARTESIAN_POINT ( 'NONE',  ( -3.749999999999999556, 6.750000000000000888, -3.499999999999999112 ) ) ;
#14629=CARTESIAN_POINT ( 'NONE',  ( -2.651650429449552870, 8.125000000000000000, -0.8483495705504462414 ) ) ;
#14631=CARTESIAN_POINT ( 'NONE',  ( 1.553300858899105963, 11.06250000000000178, -7.250000000000000888 ) ) ;
#14641=CARTESIAN_POINT ( 'NONE',  ( 0.000000000000000000, 0.5000000000000001110, -0.2500000000000002220 ) ) ;
#14645=CARTESIAN_POINT ( 'NONE',  ( 2.651650429449552870, 8.625000000000000000, -6.151650429449554203 ) ) ;
#14646=CARTESIAN_POINT ( 'NONE',  ( -1.553300858899107073, 9.937500000000001776, -7.249999999999999112 ) ) ;
#14649=CARTESIAN_POINT ( 'NONE',  ( 3.249999999999998224, 7.187500000000000888, -4.846194077712561388 ) ) ;
#14650=CARTESIAN_POINT ( 'NONE',  ( 2.651650429449552870, 8.625000000000000000, -6.151650429449554203 ) ) ;
#14653=CARTESIAN_POINT ( 'NONE',  ( 2.298097038856278473, 11.62500000000000000, -5.798097038856279362 ) ) ;
#14660=VERTEX_POINT ( 'NONE', #14530 ) ;
#14664=CARTESIAN_POINT ( 'NONE',  ( -2.651650429449552870, 12.87500000000000178, -6.151650429449552426 ) ) ;
#14666=CARTESIAN_POINT ( 'NONE',  ( 2.298097038856279362, 11.37500000000000178, -1.201902961143720860 ) ) ;
#14667=CARTESIAN_POINT ( 'NONE',  ( 2.298097038856279362, 1.875000000000000000, -1.201902961143720860 ) ) ;
#14670=CARTESIAN_POINT ( 'NONE',  ( 3.249999999999999112, 7.812500000000000000, -2.153805922287439945 ) ) ;
#14679=EDGE_LOOP ( 'NONE', ( #11773, #8838, #14178, #14871 ) ) ;
#14680=CARTESIAN_POINT ( 'NONE',  ( 3.249999999999999556, 0.7500000000000000000, -3.500000000000000000 ) ) ;
#14681=CARTESIAN_POINT ( 'NONE',  ( 2.651650429449552870, 14.62500000000000000, -6.151650429449554203 ) ) ;
#14686=CARTESIAN_POINT ( 'NONE',  ( -3.749999999999999556, 2.312500000000000888, -5.053300858899104853 ) ) ;
#14689=CARTESIAN_POINT ( 'NONE',  ( 1.553300858899105963, 2.562500000000000444, -7.250000000000000000 ) ) ;
#14690=MECHANICAL_CONTEXT ( 'NONE', #4821, 'mechanical' ) ;
#14695=CARTESIAN_POINT ( 'NONE',  ( 1.346194077712560944, 7.937500000000000000, -0.2500000000000011102 ) ) ;
#14697=CARTESIAN_POINT ( 'NONE',  ( 1.346194077712561166, 3.437500000000000444, -0.2500000000000011102 ) ) ;
#14698=CARTESIAN_POINT ( 'NONE',  ( 2.298097038856278029, 10.12500000000000000, -5.798097038856279362 ) ) ;
#14703=CARTESIAN_POINT ( 'NONE',  ( 3.249999999999998668, 6.687500000000000888, -4.846194077712560500 ) ) ;
#14705=CARTESIAN_POINT ( 'NONE',  ( -3.749999999999999556, 5.750000000000000000, -3.499999999999999112 ) ) ;
#14706=CARTESIAN_POINT ( 'NONE',  ( 3.749999999999999556, 10.81250000000000178, -1.946699141100892261 ) ) ;
#14709=CARTESIAN_POINT ( 'NONE',  ( 0.000000000000000000, 9.500000000000000000, 0.2500000000000002220 ) ) ;
#14718=CARTESIAN_POINT ( 'NONE',  ( -3.749999999999999556, 12.74999999999999822, -3.499999999999999112 ) ) ;
#14721=CARTESIAN_POINT ( 'NONE',  ( -0.3766621274091715987, 0.2004420829692335482, 0.1491815183709511161 ) ) ;
#14722=CARTESIAN_POINT ( 'NONE',  ( -3.749999999999999556, 11.31249999999999822, -5.053300858899104853 ) ) ;
#14723=CARTESIAN_POINT ( 'NONE',  ( 2.651650429449552870, 9.125000000000001776, -6.151650429449553314 ) ) ;
#14726=CARTESIAN_POINT ( 'NONE',  ( 3.249999999999999556, 7.250000000000000000, -3.500000000000000000 ) ) ;
#14728=CARTESIAN_POINT ( 'NONE',  ( -4.592425496802573972E-16, 13.50000000000000000, -7.249999999999999112 ) ) ;
#14732=CARTESIAN_POINT ( 'NONE',  ( -3.249999999999999556, 12.18750000000000000, -2.153805922287440833 ) ) ;
#14742=CARTESIAN_POINT ( 'NONE',  ( 0.000000000000000000, 11.50000000000000000, 0.2499999999999998057 ) ) ;
#14743=CARTESIAN_POINT ( 'NONE',  ( 3.249999999999999556, 12.25000000000000000, -3.500000000000000000 ) ) ;
#14744=CARTESIAN_POINT ( 'NONE',  ( 2.298097038856279362, 13.37500000000000000, -1.201902961143720860 ) ) ;
#14747=CARTESIAN_POINT ( 'NONE',  ( -2.298097038856278473, 11.12500000000000000, -1.201902961143720416 ) ) ;
#14757=CARTESIAN_POINT ( 'NONE',  ( 3.249999999999998668, 5.687500000000000000, -4.846194077712560500 ) ) ;
#14758=( BOUNDED_CURVE ( )  B_SPLINE_CURVE ( 2, ( #13839, #4483, #1868, #7954, #3321, #9191, #930, #8031, #5632, #10052, #5338, #14791, #13623, #3024, #7731, #6573, #11285, #7019, #7083, #2463, #70, #8402, #9422, #10656, #13051, #1220, #14146, #3548, #14067, #11804, #145, #8255, #5711, #9345, #2238, #5930, #4782, #15314, #2387, #15167, #10508, #8103, #3469, #9566, #4855, #5856, #14292, #2319, #10430, #10731, #9496, #14221, #3622, #7160, #4562, #3693, #11732, #8325, #11882, #1304, #6007, #4709, #11583, #9271, #8180, #2167, #1153, #6869, #1001, #13995, #12982, #3393, #12828, #6946, #4634, #11662, #1081, #5787, #15242, #12906, #10575, #11959, #6250, #4096, #5094, #10802, #7322, #5248, #2697, #385, #8637, #3778, #8558, #1616, #6163, #9807, #7246, #2544, #12035, #13293, #4931, #1687, #10883, #1456, #7396, #9881, #3860, #303, #13134, #13373, #14538, #10967, #6398, #8486, #6328, #1383, #533, #1536, #12119, #3935, #5016, #12277, #2778, #9956, #9735, #7482, #12200, #14695, #11112, #6085, #11043, #14619, #13217, #459, #216, #5169, #4017, #8718, #13454, #2858, #7558, #9648, #2619, #14380, #14464, #8070, #5321, #4527, #6768, #13529, #616, #12720, #11191, #10397, #11481, #13888, #2282, #15053, #8799, #2927, #15279, #5753, #6988, #7631, #12347, #15208, #1765, #12793, #5823, #10546, #9309, #14033, #2131, #12642, #6475, #6834, #10034, #10314, #7922, #4375, #11550, #3205, #9160, #14771, #2056, #3429, #2200, #899, #8141, #9084, #966, #5600, #9236, #3284, #11627, #13805, #4447, #4601, #12870, #11704, #7999, #5673, #15132, #13964, #3359, #6907, #1122, #1045, #10475, #10930, #11844, #14111, #1269, #5974, #14265, #7365, #9695, #1191, #10615, #4671, #14340, #6053, #3664, #7288, #7055, #3825, #3513, #37, #13181, #8220, #7206, #1504, #189, #10697, #8448, #13023, #8526, #6215, #8365, #113, #14190 ),
 .UNSPECIFIED., .F., .F. ) 
 B_SPLINE_CURVE_WITH_KNOTS ( ( 3, 2, 2, 2, 2, 2, 2, 2, 2, 2, 2, 2, 2, 2, 2, 2, 2, 2, 2, 2, 2, 2, 2, 2, 2, 2, 2, 2, 2, 2, 2, 2, 2, 2, 2, 2, 2, 2, 2, 2, 2, 2, 2, 2, 2, 2, 2, 2, 2, 2, 2, 2, 2, 2, 2, 2, 2, 2, 2, 2, 2, 2, 2, 2, 2, 2, 2, 2, 2, 2, 2, 2, 2, 2, 2, 2, 2, 2, 2, 2, 2, 2, 2, 2, 2, 2, 2, 2, 2, 2, 2, 2, 2, 2, 2, 2, 2, 2, 2, 2, 2, 2, 2, 2, 2, 2, 2, 2, 2, 2, 2, 2, 2, 2, 2, 2, 2, 2, 2, 2, 3 ),
 ( 0.000000000000000000, 0.008333333333333333218, 0.01666666666666666644, 0.02500000000000000139, 0.03333333333333333287, 0.04166666666666666435, 0.05000000000000000278, 0.05833333333333333426, 0.06666666666666666574, 0.07499999999999999722, 0.08333333333333332871, 0.09166666666666666019, 0.1000000000000000056, 0.1083333333333333370, 0.1166666666666666685, 0.1250000000000000000, 0.1333333333333333315, 0.1416666666666666630, 0.1499999999999999944, 0.1583333333333333259, 0.1666666666666666574, 0.1749999999999999889, 0.1833333333333333204, 0.1916666666666666519, 0.2000000000000000111, 0.2083333333333333426, 0.2166666666666666741, 0.2250000000000000056, 0.2333333333333333370, 0.2416666666666666685, 0.2500000000000000000, 0.2583333333333333037, 0.2666666666666666630, 0.2750000000000000222, 0.2833333333333333259, 0.2916666666666666852, 0.2999999999999999889, 0.3083333333333333481, 0.3166666666666666519, 0.3250000000000000111, 0.3333333333333333148, 0.3416666666666666741, 0.3499999999999999778, 0.3583333333333333370, 0.3666666666666666408, 0.3750000000000000000, 0.3833333333333333037, 0.3916666666666666630, 0.4000000000000000222, 0.4083333333333333259, 0.4166666666666666852, 0.4249999999999999889, 0.4333333333333333481, 0.4416666666666666519, 0.4500000000000000111, 0.4583333333333333148, 0.4666666666666666741, 0.4749999999999999778, 0.4833333333333333370, 0.4916666666666666408, 0.5000000000000000000, 0.5083333333333333037, 0.5166666666666666075, 0.5250000000000000222, 0.5333333333333333259, 0.5416666666666666297, 0.5500000000000000444, 0.5583333333333333481, 0.5666666666666666519, 0.5749999999999999556, 0.5833333333333333703, 0.5916666666666666741, 0.5999999999999999778, 0.6083333333333332815, 0.6166666666666666963, 0.6250000000000000000, 0.6333333333333333037, 0.6416666666666666075, 0.6500000000000000222, 0.6583333333333333259, 0.6666666666666666297, 0.6750000000000000444, 0.6833333333333333481, 0.6916666666666666519, 0.6999999999999999556, 0.7083333333333333703, 0.7166666666666666741, 0.7249999999999999778, 0.7333333333333332815, 0.7416666666666666963, 0.7500000000000000000, 0.7583333333333333037, 0.7666666666666666075, 0.7750000000000000222, 0.7833333333333333259, 0.7916666666666666297, 0.8000000000000000444, 0.8083333333333333481, 0.8166666666666666519, 0.8249999999999999556, 0.8333333333333333703, 0.8416666666666666741, 0.8499999999999999778, 0.8583333333333332815, 0.8666666666666666963, 0.8750000000000000000, 0.8833333333333333037, 0.8916666666666666075, 0.9000000000000000222, 0.9083333333333333259, 0.9166666666666666297, 0.9249999999999999334, 0.9333333333333333481, 0.9416666666666666519, 0.9499999999999999556, 0.9583333333333333703, 0.9666666666666666741, 0.9749999999999999778, 0.9833333333333332815, 0.9916666666666666963, 1.000000000000000000 ),
 .UNSPECIFIED. ) 
 CURVE ( )  GEOMETRIC_REPRESENTATION_ITEM ( )  RATIONAL_B_SPLINE_CURVE ( ( 1.000000000000000000, 0.9238795325112867385, 1.000000000000000000, 0.9238795325112867385, 1.000000000000000000, 0.9238795325112867385, 1.000000000000000000, 0.9238795325112867385, 1.000000000000000000, 0.9238795325112867385, 1.000000000000000000, 0.9238795325112867385, 1.000000000000000000, 0.9238795325112867385, 1.000000000000000000, 0.9238795325112867385, 1.000000000000000000, 0.9238795325112867385, 1.000000000000000000, 0.9238795325112867385, 1.000000000000000000, 0.9238795325112867385, 1.000000000000000000, 0.9238795325112867385, 1.000000000000000000, 0.9238795325112867385, 1.000000000000000000, 0.9238795325112867385, 1.000000000000000000, 0.9238795325112867385, 1.000000000000000000, 0.9238795325112867385, 1.000000000000000000, 0.9238795325112867385, 1.000000000000000000, 0.9238795325112867385, 1.000000000000000000, 0.9238795325112867385, 1.000000000000000000, 0.9238795325112867385, 1.000000000000000000, 0.9238795325112867385, 1.000000000000000000, 0.9238795325112867385, 1.000000000000000000, 0.9238795325112867385, 1.000000000000000000, 0.9238795325112867385, 1.000000000000000000, 0.9238795325112867385, 1.000000000000000000, 0.9238795325112867385, 1.000000000000000000, 0.9238795325112867385, 1.000000000000000000, 0.9238795325112867385, 1.000000000000000000, 0.9238795325112867385, 1.000000000000000000, 0.9238795325112867385, 1.000000000000000000, 0.9238795325112867385, 1.000000000000000000, 0.9238795325112867385, 1.000000000000000000, 0.9238795325112867385, 1.000000000000000000, 0.9238795325112867385, 1.000000000000000000, 0.9238795325112867385, 1.000000000000000000, 0.9238795325112867385, 1.000000000000000000, 0.9238795325112867385, 1.000000000000000000, 0.9238795325112867385, 1.000000000000000000, 0.9238795325112867385, 1.000000000000000000, 0.9238795325112867385, 1.000000000000000000, 0.9238795325112867385, 1.000000000000000000, 0.9238795325112867385, 1.000000000000000000, 0.9238795325112867385, 1.000000000000000000, 0.9238795325112867385, 1.000000000000000000, 0.9238795325112867385, 1.000000000000000000, 0.9238795325112867385, 1.000000000000000000, 0.9238795325112867385, 1.000000000000000000, 0.9238795325112867385, 1.000000000000000000, 0.9238795325112867385, 1.000000000000000000, 0.9238795325112867385, 1.000000000000000000, 0.9238795325112867385, 1.000000000000000000, 0.9238795325112867385, 1.000000000000000000, 0.9238795325112867385, 1.000000000000000000, 0.9238795325112867385, 1.000000000000000000, 0.9238795325112867385, 1.000000000000000000, 0.9238795325112867385, 1.000000000000000000, 0.9238795325112867385, 1.000000000000000000, 0.9238795325112867385, 1.000000000000000000, 0.9238795325112867385, 1.000000000000000000, 0.9238795325112867385, 1.000000000000000000, 0.9238795325112867385, 1.000000000000000000, 0.9238795325112867385, 1.000000000000000000, 0.9238795325112867385, 1.000000000000000000, 0.9238795325112867385, 1.000000000000000000, 0.9238795325112867385, 1.000000000000000000, 0.9238795325112867385, 1.000000000000000000, 0.9238795325112867385, 1.000000000000000000, 0.9238795325112867385, 1.000000000000000000, 0.9238795325112867385, 1.000000000000000000, 0.9238795325112867385, 1.000000000000000000, 0.9238795325112867385, 1.000000000000000000, 0.9238795325112867385, 1.000000000000000000, 0.9238795325112867385, 1.000000000000000000, 0.9238795325112867385, 1.000000000000000000, 0.9238795325112867385, 1.000000000000000000, 0.9238795325112867385, 1.000000000000000000, 0.9238795325112867385, 1.000000000000000000, 0.9238795325112867385, 1.000000000000000000, 0.9238795325112867385, 1.000000000000000000, 0.9238795325112867385, 1.000000000000000000, 0.9238795325112867385, 1.000000000000000000, 0.9238795325112867385, 1.000000000000000000, 0.9238795325112867385, 1.000000000000000000, 0.9238795325112867385, 1.000000000000000000, 0.9238795325112867385, 1.000000000000000000, 0.9238795325112867385, 1.000000000000000000, 0.9238795325112867385, 1.000000000000000000, 0.9238795325112867385, 1.000000000000000000, 0.9238795325112867385, 1.000000000000000000, 0.9238795325112867385, 1.000000000000000000, 0.9238795325112867385, 1.000000000000000000, 0.9238795325112867385, 1.000000000000000000, 0.9238795325112867385, 1.000000000000000000, 0.9238795325112867385, 1.000000000000000000, 0.9238795325112867385, 1.000000000000000000, 0.9238795325112867385, 1.000000000000000000, 0.9238795325112867385, 1.000000000000000000, 0.9238795325112867385, 1.000000000000000000, 0.9238795325112867385, 1.000000000000000000, 0.9238795325112867385, 1.000000000000000000, 0.9238795325112867385, 1.000000000000000000, 0.9238795325112867385, 1.000000000000000000, 0.9238795325112867385, 1.000000000000000000, 0.9238795325112867385, 1.000000000000000000, 0.9238795325112867385, 1.000000000000000000, 0.9238795325112867385, 1.000000000000000000, 0.9238795325112867385, 1.000000000000000000, 0.9238795325112867385, 1.000000000000000000, 0.9238795325112867385, 1.000000000000000000, 0.9238795325112867385, 1.000000000000000000, 0.9238795325112867385, 1.000000000000000000, 0.9238795325112867385, 1.000000000000000000, 0.9238795325112867385, 1.000000000000000000, 0.9238795325112867385, 1.000000000000000000, 0.9238795325112867385, 1.000000000000000000, 0.9238795325112867385, 1.000000000000000000, 0.9238795325112867385, 1.000000000000000000, 0.9238795325112867385, 1.000000000000000000, 0.9238795325112867385, 1.000000000000000000, 0.9238795325112867385, 1.000000000000000000 ) ) 
 REPRESENTATION_ITEM ( '' )  );
#14759=CARTESIAN_POINT ( 'NONE',  ( 3.749999999999999112, 11.81249999999999822, -1.946699141100892039 ) ) ;
#14762=CARTESIAN_POINT ( 'NONE',  ( 0.000000000000000000, 15.50000000000000178, 0.2499999999999998057 ) ) ;
#14771=CARTESIAN_POINT ( 'NONE',  ( -1.346194077712559167, 11.43750000000000000, -6.749999999999999112 ) ) ;
#14773=CARTESIAN_POINT ( 'NONE',  ( -3.249999999999999112, 1.812499999999999778, -4.846194077712558723 ) ) ;
#14774=CARTESIAN_POINT ( 'NONE',  ( 1.346194077712561166, 9.437500000000000000, -0.2500000000000011102 ) ) ;
#14777=CARTESIAN_POINT ( 'NONE',  ( -1.346194077712559389, 5.437500000000002665, -6.749999999999999112 ) ) ;
#14778=CARTESIAN_POINT ( 'NONE',  ( 2.651650429449552870, 5.125000000000000000, -6.151650429449553314 ) ) ;
#14779=CARTESIAN_POINT ( 'NONE',  ( -1.553300858899106407, 8.062500000000000000, 0.2500000000000002220 ) ) ;
#14783=CARTESIAN_POINT ( 'NONE',  ( -2.651650429449553314, 11.87500000000000000, -6.151650429449552426 ) ) ;
#14791=CARTESIAN_POINT ( 'NONE',  ( 3.249999999999998668, 0.6875000000000000000, -4.846194077712560500 ) ) ;
#14793=CARTESIAN_POINT ( 'NONE',  ( -1.553300858899106629, 13.56250000000000000, 0.2500000000000002220 ) ) ;
#14797=CARTESIAN_POINT ( 'NONE',  ( 1.553300858899109071, 10.43750000000000178, 0.2499999999999989175 ) ) ;
#14800=CARTESIAN_POINT ( 'NONE',  ( -3.249999999999999556, 8.750000000000001776, -3.500000000000000000 ) ) ;
#14802=CARTESIAN_POINT ( 'NONE',  ( 2.651650429449552870, 12.62500000000000000, -6.151650429449554203 ) ) ;
#14805=CARTESIAN_POINT ( 'NONE',  ( 3.249999999999998668, 10.68750000000000000, -4.846194077712560500 ) ) ;
#14815=CARTESIAN_POINT ( 'NONE',  ( 0.000000000000000000, 15.50000000000000178, 0.2499999999999998057 ) ) ;
#14816=CARTESIAN_POINT ( 'NONE',  ( -2.298097038856279362, 9.875000000000000000, -5.798097038856278473 ) ) ;
#14817=CARTESIAN_POINT ( 'NONE',  ( 0.000000000000000000, 1.000000000000000000, -0.2500000000000002220 ) ) ;
#14819=CARTESIAN_POINT ( 'NONE',  ( 3.249999999999999556, 10.75000000000000000, -3.500000000000000000 ) ) ;
#14830=CARTESIAN_POINT ( 'NONE',  ( 3.249999999999999556, 3.750000000000000000, -3.500000000000000000 ) ) ;
#14832=CARTESIAN_POINT ( 'NONE',  ( 1.553300858899105963, 3.062500000000000000, -7.250000000000000888 ) ) ;
#14837=CARTESIAN_POINT ( 'NONE',  ( -1.553300858899107295, 3.437500000000000000, -7.250000000000000000 ) ) ;
#14840=CARTESIAN_POINT ( 'NONE',  ( -3.750000000000000000, 1.312500000000000222, -5.053300858899105741 ) ) ;
#14844=PLANE ( 'NONE',  #13849 ) ;
#14849=CARTESIAN_POINT ( 'NONE',  ( -1.346194077712559167, 1.937500000000000222, -6.749999999999999112 ) ) ;
#14850=CARTESIAN_POINT ( 'NONE',  ( -3.980102097228897738E-16, 13.00000000000000000, -6.749999999999999112 ) ) ;
#14855=CARTESIAN_POINT ( 'NONE',  ( -3.749999999999999556, 3.750000000000000444, -3.499999999999999112 ) ) ;
#14856=VECTOR ( 'NONE', #7001, 1000.000000000000000 ) ;
#14857=CARTESIAN_POINT ( 'NONE',  ( -4.592425496802573972E-16, 8.500000000000000000, -7.249999999999999112 ) ) ;
#14861=CARTESIAN_POINT ( 'NONE',  ( -1.553300858899106629, 8.562500000000000000, 0.2500000000000002220 ) ) ;
#14870=CARTESIAN_POINT ( 'NONE',  ( 2.651650429449554203, 12.37500000000000178, -0.8483495705504471296 ) ) ;
#14871=ORIENTED_EDGE ( 'NONE', *, *, #7532, .T. ) ;
#14876=CARTESIAN_POINT ( 'NONE',  ( -1.346194077712558945, 9.562500000000000000, -0.2500000000000002220 ) ) ;
#14878=CARTESIAN_POINT ( 'NONE',  ( 1.553300858899108849, 11.93750000000000000, 0.2499999999999993616 ) ) ;
#14881=CARTESIAN_POINT ( 'NONE',  ( 2.298097038856278473, 12.62500000000000000, -5.798097038856279362 ) ) ;
#14884=CARTESIAN_POINT ( 'NONE',  ( 0.000000000000000000, 9.000000000000001776, -0.2500000000000002220 ) ) ;
#14887=CARTESIAN_POINT ( 'NONE',  ( -3.249999999999999112, 5.687500000000000888, -2.153805922287440833 ) ) ;
#14889=CARTESIAN_POINT ( 'NONE',  ( 0.000000000000000000, 1.530808498934191509E-17, 0.000000000000000000 ) ) ;
#14891=CARTESIAN_POINT ( 'NONE',  ( -1.553300858899107295, 0.4375000000000000555, -7.250000000000000000 ) ) ;
#14892=CARTESIAN_POINT ( 'NONE',  ( -2.651650429449552870, 0.6249999999999998890, -0.8483495705504467965 ) ) ;
#14893=CARTESIAN_POINT ( 'NONE',  ( -3.249999999999999556, 1.250000000000000000, -3.499999999999999556 ) ) ;
#14896=CARTESIAN_POINT ( 'NONE',  ( 1.346194077712558057, 9.562500000000000000, -6.750000000000000000 ) ) ;
#14908=CARTESIAN_POINT ( 'NONE',  ( -2.298097038856278473, 5.125000000000000000, -1.201902961143720416 ) ) ;
#14910=CARTESIAN_POINT ( 'NONE',  ( -3.750000000000000000, 0.6875000000000000000, -1.946699141100893149 ) ) ;
#14913=CARTESIAN_POINT ( 'NONE',  ( -0.3766621274091715987, 0.5000000000000000000, 0.1491815183709511716 ) ) ;
#14915=CARTESIAN_POINT ( 'NONE',  ( -2.651650429449553314, 5.375000000000000000, -6.151650429449552426 ) ) ;
#14920=CARTESIAN_POINT ( 'NONE',  ( 3.750000000000000000, 2.750000000000000000, -3.500000000000000444 ) ) ;
#14927=CARTESIAN_POINT ( 'NONE',  ( 1.346194077712561166, 1.437500000000000000, -0.2500000000000011102 ) ) ;
#14930=CARTESIAN_POINT ( 'NONE',  ( 1.553300858899109071, 5.437500000000000888, 0.2499999999999989175 ) ) ;
#14932=CARTESIAN_POINT ( 'NONE',  ( 3.749999999999999112, 11.68750000000000000, -5.053300858899108405 ) ) ;
#14933=CARTESIAN_POINT ( 'NONE',  ( 0.3766621274091715987, -0.2500000000000000000, -7.146945437571387671 ) ) ;
#14936=CARTESIAN_POINT ( 'NONE',  ( 3.749999999999999556, 12.25000000000000000, -3.500000000000000444 ) ) ;
#14945=CARTESIAN_POINT ( 'NONE',  ( 3.249999999999998224, 4.312500000000000000, -2.153805922287439945 ) ) ;
#14953=CARTESIAN_POINT ( 'NONE',  ( -2.298097038856278029, 8.625000000000000000, -1.201902961143720638 ) ) ;
#14955=CARTESIAN_POINT ( 'NONE',  ( -2.651650429449552870, -0.3749999999999998890, -0.8483495705504463524 ) ) ;
#14958=CARTESIAN_POINT ( 'NONE',  ( 3.249999999999998668, 12.68750000000000178, -4.846194077712560500 ) ) ;
#14962=CARTESIAN_POINT ( 'NONE',  ( -1.346194077712559389, 10.43750000000000000, -6.749999999999999112 ) ) ;
#14968=CARTESIAN_POINT ( 'NONE',  ( 3.749999999999998668, 0.6875000000000000000, -5.053300858899107517 ) ) ;
#14969=CARTESIAN_POINT ( 'NONE',  ( 2.298097038856279362, 14.37500000000000000, -1.201902961143720860 ) ) ;
#14970=CARTESIAN_POINT ( 'NONE',  ( -2.298097038856278918, 1.375000000000000000, -5.798097038856277585 ) ) ;
#14972=CARTESIAN_POINT ( 'NONE',  ( 2.298097038856278473, 9.625000000000000000, -5.798097038856279362 ) ) ;
#14980=ORIENTED_EDGE ( 'NONE', *, *, #3847, .F. ) ;
#14981=CARTESIAN_POINT ( 'NONE',  ( -3.249999999999999556, 5.312500000000001776, -4.846194077712557835 ) ) ;
#14983=CARTESIAN_POINT ( 'NONE',  ( 3.750000000000000000, 1.312500000000000444, -1.946699141100892705 ) ) ;
#14987=CARTESIAN_POINT ( 'NONE',  ( 3.749999999999999112, 4.812500000000000888, -1.946699141100892039 ) ) ;
#14994=CARTESIAN_POINT ( 'NONE',  ( -1.346194077712558945, 2.562500000000000444, -0.2500000000000002220 ) ) ;
#14997=CARTESIAN_POINT ( 'NONE',  ( 2.651650429449552870, 11.12500000000000178, -6.151650429449553314 ) ) ;
#14998=CLOSED_SHELL ( 'NONE', ( #2121, #10932, #11025, #7907, #11211, #15210, #12175, #5825, #13504, #12535, #2261, #12689, #12969, #15295, #1863, #7437, #1754 ) ) ;
#14999=CARTESIAN_POINT ( 'NONE',  ( 1.553300858899105963, 11.56250000000000000, -7.250000000000000000 ) ) ;
#15003=CARTESIAN_POINT ( 'NONE',  ( -2.298097038856279362, 0.8750000000000000000, -5.798097038856278473 ) ) ;
#15015=CARTESIAN_POINT ( 'NONE',  ( -2.298097038856278029, 4.625000000000000888, -1.201902961143720638 ) ) ;
#15020=CARTESIAN_POINT ( 'NONE',  ( 2.298097038856278473, 10.62500000000000000, -5.798097038856279362 ) ) ;
#15023=CARTESIAN_POINT ( 'NONE',  ( 3.249999999999998224, 14.18750000000000178, -4.846194077712561388 ) ) ;
#15026=CARTESIAN_POINT ( 'NONE',  ( 2.651650429449553759, 14.87500000000000178, -0.8483495705504471296 ) ) ;
#15029=DIRECTION ( 'NONE',  ( 0.000000000000000000, 0.000000000000000000, 1.000000000000000000 ) ) ;
#15032=CARTESIAN_POINT ( 'NONE',  ( 2.298097038856278473, 7.625000000000000000, -5.798097038856279362 ) ) ;
#15038=CARTESIAN_POINT ( 'NONE',  ( -3.750000000000000000, 14.68750000000000178, -1.946699141100893149 ) ) ;
#15039=CARTESIAN_POINT ( 'NONE',  ( -3.249999999999999112, 13.68750000000000178, -2.153805922287440833 ) ) ;
#15042=CARTESIAN_POINT ( 'NONE',  ( -3.249999999999999556, 7.312500000000000888, -4.846194077712557835 ) ) ;
#15043=CARTESIAN_POINT ( 'NONE',  ( -3.249999999999999556, 13.31250000000000000, -4.846194077712557835 ) ) ;
#15053=CARTESIAN_POINT ( 'NONE',  ( 3.249999999999999112, 9.812500000000000000, -2.153805922287439945 ) ) ;
#15056=CARTESIAN_POINT ( 'NONE',  ( 3.249999999999999112, 4.812500000000000888, -2.153805922287439945 ) ) ;
#15058=CARTESIAN_POINT ( 'NONE',  ( -2.651650429449553314, 0.8750000000000000000, -6.151650429449552426 ) ) ;
#15059=CARTESIAN_POINT ( 'NONE',  ( -3.249999999999999112, 5.812500000000000888, -4.846194077712558723 ) ) ;
#15062=DIRECTION ( 'NONE',  ( -0.000000000000000000, -1.000000000000000000, -0.000000000000000000 ) ) ;
#15063=CARTESIAN_POINT ( 'NONE',  ( -3.749999999999999556, 5.187500000000001776, -1.946699141100892927 ) ) ;
#15071=VECTOR ( 'NONE', #6143, 1000.000000000000000 ) ;
#15072=CARTESIAN_POINT ( 'NONE',  ( 1.346194077712558279, 8.062500000000001776, -6.750000000000000888 ) ) ;
#15074=CARTESIAN_POINT ( 'NONE',  ( 3.749999999999999556, 9.250000000000001776, -3.500000000000000444 ) ) ;
#15075=CARTESIAN_POINT ( 'NONE',  ( 1.553300858899105963, 12.56250000000000000, -7.250000000000000000 ) ) ;
#15080=CARTESIAN_POINT ( 'NONE',  ( -3.749999999999999556, 12.74999999999999822, -3.499999999999999112 ) ) ;
#15087=DIRECTION ( 'NONE',  ( 0.000000000000000000, 1.000000000000000000, 0.000000000000000000 ) ) ;
#15092=CARTESIAN_POINT ( 'NONE',  ( 2.298097038856279362, 3.375000000000000444, -1.201902961143720860 ) ) ;
#15099=CARTESIAN_POINT ( 'NONE',  ( 1.346194077712558279, 13.06250000000000178, -6.750000000000000888 ) ) ;
#15102=CARTESIAN_POINT ( 'NONE',  ( -2.651650429449553314, 1.874999999999999778, -6.151650429449552426 ) ) ;
#15109=CARTESIAN_POINT ( 'NONE',  ( -3.980102097228897245E-16, 9.500000000000000000, -6.749999999999999112 ) ) ;
#15111=APPLICATION_CONTEXT ( 'configuration controlled 3d designs of mechanical parts and assemblies' ) ;
#15116=PLANE ( 'NONE',  #2575 ) ;
#15117=CARTESIAN_POINT ( 'NONE',  ( -4.592425496802573972E-16, 15.00000000000000178, -7.250000000000000000 ) ) ;
#15118=CARTESIAN_POINT ( 'NONE',  ( 3.749999999999998668, 1.187499999999999778, -5.053300858899108405 ) ) ;
#15121=CARTESIAN_POINT ( 'NONE',  ( -2.298097038856278473, 14.12500000000000000, -1.201902961143720416 ) ) ;
#15125=CARTESIAN_POINT ( 'NONE',  ( 1.346194077712558057, 5.562500000000000000, -6.750000000000000000 ) ) ;
#15132=CARTESIAN_POINT ( 'NONE',  ( 2.298097038856278473, 12.62500000000000000, -5.798097038856279362 ) ) ;
#15135=CARTESIAN_POINT ( 'NONE',  ( -2.651650429449552870, 11.62500000000000000, -0.8483495705504463524 ) ) ;
#15137=CARTESIAN_POINT ( 'NONE',  ( -1.553300858899107073, 1.937500000000000222, -7.249999999999999112 ) ) ;
#15138=CARTESIAN_POINT ( 'NONE',  ( -3.980102097228897738E-16, 6.000000000000000888, -6.749999999999999112 ) ) ;
#15141=CARTESIAN_POINT ( 'NONE',  ( 3.249999999999999556, 4.750000000000000000, -3.500000000000000000 ) ) ;
#15143=B_SPLINE_CURVE_WITH_KNOTS ( 'NONE', 3,
 ( #5722, #9508, #4721, #10667, #14159, #4571 ),
 .UNSPECIFIED., .F., .F.,
 ( 4, 2, 4 ),
 ( 0.000000000000000000, 0.0003771714294063781151, 0.0007543428588127562302 ),
 .UNSPECIFIED. ) ;
#15144=CARTESIAN_POINT ( 'NONE',  ( 2.651650429449552870, 5.625000000000000000, -6.151650429449554203 ) ) ;
#15151=CARTESIAN_POINT ( 'NONE',  ( 0.000000000000000000, 6.500000000000000000, -0.2500000000000002220 ) ) ;
#15154=CARTESIAN_POINT ( 'NONE',  ( -3.750000000000000000, 8.812500000000001776, -5.053300858899105741 ) ) ;
#15159=CARTESIAN_POINT ( 'NONE',  ( 1.553300858899109516, 14.43750000000000178, 0.2499999999999993616 ) ) ;
#15167=CARTESIAN_POINT ( 'NONE',  ( -1.346194077712559167, 2.437500000000000444, -6.749999999999999112 ) ) ;
#15171=CARTESIAN_POINT ( 'NONE',  ( -1.346194077712559167, 2.937500000000000444, -6.749999999999999112 ) ) ;
#15177=CARTESIAN_POINT ( 'NONE',  ( -3.249999999999999556, 13.75000000000000000, -3.500000000000000000 ) ) ;
#15178=VECTOR ( 'NONE', #14017, 1000.000000000000000 ) ;
#15180=CARTESIAN_POINT ( 'NONE',  ( 3.749999999999999112, 1.187500000000000222, -5.053300858899108405 ) ) ;
#15186=CARTESIAN_POINT ( 'NONE',  ( 2.298097038856279362, 11.87500000000000000, -1.201902961143720860 ) ) ;
#15193=CARTESIAN_POINT ( 'NONE',  ( -3.749999999999999556, 3.187500000000000000, -1.946699141100892927 ) ) ;
#15194=CARTESIAN_POINT ( 'NONE',  ( -2.298097038856278029, 14.62500000000000178, -1.201902961143720638 ) ) ;
#15198=CARTESIAN_POINT ( 'NONE',  ( -2.298097038856278029, 1.625000000000000000, -1.201902961143720638 ) ) ;
#15201=CARTESIAN_POINT ( 'NONE',  ( -1.346194077712559389, 4.437500000000000888, -6.749999999999999112 ) ) ;
#15207=DIRECTION ( 'NONE',  ( 1.000000000000000000, -0.000000000000000000, 0.000000000000000000 ) ) ;
#15208=CARTESIAN_POINT ( 'NONE',  ( -3.249999999999999556, 10.31250000000000000, -4.846194077712557835 ) ) ;
#15209=VERTEX_POINT ( 'NONE', #12324 ) ;
#15210=ADVANCED_FACE ( 'NONE', ( #8849 ), #7841, .F. ) ;
#15212=CARTESIAN_POINT ( 'NONE',  ( 2.651650429449554203, 9.374999999999998224, -0.8483495705504471296 ) ) ;
#15214=CARTESIAN_POINT ( 'NONE',  ( 3.749999999999999112, 4.187500000000000888, -5.053300858899108405 ) ) ;
#15216=CARTESIAN_POINT ( 'NONE',  ( 2.298097038856278029, 8.125000000000000000, -5.798097038856279362 ) ) ;
#15220=CARTESIAN_POINT ( 'NONE',  ( -1.346194077712559389, 2.062500000000000000, -0.2500000000000002220 ) ) ;
#15221=CARTESIAN_POINT ( 'NONE',  ( -1.553300858899107295, 5.437500000000002665, -7.250000000000000000 ) ) ;
#15226=DIRECTION ( 'NONE',  ( -1.000000000000000000, 0.000000000000000000, 0.000000000000000000 ) ) ;
#15228=CARTESIAN_POINT ( 'NONE',  ( -1.346194077712559167, 6.937500000000001776, -6.749999999999999112 ) ) ;
#15231=CARTESIAN_POINT ( 'NONE',  ( -3.749999999999999556, 7.750000000000000888, -3.499999999999999112 ) ) ;
#15232=CARTESIAN_POINT ( 'NONE',  ( -4.592425496802573972E-16, 11.50000000000000000, -7.249999999999999112 ) ) ;
#15235=CARTESIAN_POINT ( 'NONE',  ( -3.249999999999999556, 8.312500000000000000, -4.846194077712557835 ) ) ;
#15236=CARTESIAN_POINT ( 'NONE',  ( 3.249999999999998224, 0.1875000000000000833, -4.846194077712561388 ) ) ;
#15242=CARTESIAN_POINT ( 'NONE',  ( 2.298097038856279362, 4.875000000000000000, -1.201902961143720860 ) ) ;
#15244=CARTESIAN_POINT ( 'NONE',  ( 2.298097038856279362, 7.375000000000000000, -1.201902961143720860 ) ) ;
#15246=DIRECTION ( 'NONE',  ( 1.000000000000000000, 0.000000000000000000, 0.000000000000000000 ) ) ;
#15247=( BOUNDED_SURFACE ( )  B_SPLINE_SURFACE ( 3, 2, ( 
 ( #8262, #12991, #11740, #8492, #1160, #3702, #154, #14302, #1312, #6094, #9575, #13143, #12914, #11889, #14156, #8188, #2327, #4791, #7027, #2472, #2395, #5940, #9656, #1230, #10809, #5863, #225, #10582, #2226, #9430, #79, #4940, #4719, #9505, #13224, #14229, #3631, #13058, #7169, #6017, #10739, #2553, #7253, #11971, #14387, #9742, #8878, #1623, #1693, #12354, #9964, #1774, #3943, #14627, #6174, #14471, #13381, #7638, #11050, #12283, #6483, #7404, #6336, #2934, #13461, #310, #14548, #5254, #4024, #2787, #10974, #3867, #8569, #12042, #11200, #5024, #541, #13610, #3012, #622, #5328, #13301, #4104, #10040, #5101, #7489, #466, #14777, #1463, #2704, #12129, #8805, #1545, #6258, #4174, #9815, #392, #5179, #13535, #12207, #8645, #10894, #6404, #8729, #9889, #2865, #7564, #14703, #11122, #694, #1855, #6560, #11273, #12433, #7719, #2119, #888, #15042, #10382, #11472, #5592, #12513, #6794, #851, #924, #1072, #12821, #5483, #9035, #8958, #8024, #9263, #2229, #15235, #777, #3155, #12589, #2006, #6717, #11429, #6242, #2979, #10822, #239, #6384, #12099, #13118, #129, #370, #7306, #5080, #5153, #13355, #1367, #6070, #4916, #10950, #9793, #14363, #3763, #14523, #3103, #13774, #1875, #6580, #11368, #12681, #10216, #5569, #10354, #15020, #4410, #7099, #13235, #11899, #7339, #3876, #652, #7789, #11338, #11188, #12553, #12785, #10463, #14296, #9499, #13900, #11639, #2225, #5778, #2699, #10969, #6087, #4019, #4857, #14540, #14295, #7484, #14382, #6253, #2780, #7248, #8488, #461, #3938, #7325, #5171, #9568, #13296, #2621, #387, #9737, #12202, #1689, #3781, #6330, #9883, #11045, #13219, #7398, #14621, #8639, #9650, #8722, #12121, #12279, #12037, #9809, #8560, #7560, #13456, #6400, #1539, #1618, #218, #14466, #147, #5096, #13375, #2860, #3695 ),
 ( #11962, #8404, #1458, #13136, #1386, #3862, #2547, #10804, #6165, #5019, #4934, #10887, #305, #536, #4098, #14927, #7940, #12659, #11422, #845, #4249, #14773, #2076, #14849, #1850, #8950, #9099, #11114, #12349, #2930, #3147, #6478, #5323, #14994, #4170, #8874, #5395, #7861, #6555, #13605, #5250, #11341, #13680, #3079, #4392, #1767, #4323, #14697, #13821, #7793, #11267, #12503, #3007, #7712, #690, #6709, #5547, #767, #9960, #12429, #8801, #10110, #1921, #6633, #3225, #10262, #7633, #11195, #13531, #5474, #10193, #9027, #618, #10036, #13752, #12581, #1995, #15298, #5843, #3307, #2301, #4549, #11500, #13909, #10496, #9178, #8164, #9256, #11647, #271, #12813, #7293, #915, #12006, #10332, #986, #15151, #13982, #10852, #12742, #3378, #14433, #9701, #15228, #5618, #13265, #7006, #8088, #11720, #9406, #4689, #1432, #4468, #3830, #1064, #1140, #6138, #14131, #4985, #2221, #9332, #15072, #8016, #6930, #2592, #5773, #10563, #8531, #2151, #4620, #12968, #12892, #6855, #14052, #3530, #3451, #8240, #5696, #11569, #10416, #6788, #8842, #13569, #11016, #503, #2970, #11163, #12171, #1816, #5221, #14816, #1588, #12316, #11084, #10081, #6527, #8918, #4070, #4142, #2750, #1659, #2670, #9931, #2900, #584, #8771, #3911, #6372, #6446, #14511, #1509, #8607, #5297, #6221, #14666, #4213, #13503, #14585, #10009, #431, #11241, #7370, #7601, #9852, #6299, #3987, #7454, #1734, #14743, #7682, #12395, #354, #5141, #660, #12085, #5365, #12249, #10936, #8692, #13427, #13342, #5067, #2831, #9779, #7531, #953, #9071, #2041, #5658, #11390, #7760, #15039, #6753, #4587, #5587, #6822, #9218, #12703, #10301, #4433, #10236, #7982, #14969, #4290, #11465, #8994, #15194, #9144, #13647, #3049, #11538, #13869, #4509, #6892, #3269, #12474, #885, #1892, #2116, #11311, #7835 ),
 ( #11612, #6602, #14892, #5437, #10379, #13722, #12549, #2188, #6675, #1960, #7902, #15118, #4362, #812, #732, #13948, #3345, #8053, #1031, #3121, #12781, #10157, #5514, #5737, #13792, #10456, #3190, #12627, #7187, #9525, #9594, #2493, #8351, #5812, #4811, #7041, #14019, #1107, #13008, #11689, #10681, #11758, #14176, #2574, #20, #14322, #3416, #3726, #12855, #3498, #2345, #1178, #13164, #15265, #5879, #1411, #11988, #2413, #8126, #247, #14246, #10599, #3648, #11910, #1335, #8431, #6973, #6116, #3578, #13077, #7274, #6038, #10829, #4736, #11829, #2268, #10532, #9447, #4882, #8280, #10758, #9294, #4656, #7109, #175, #99, #9365, #1253, #14095, #5959, #8204, #12935, #2649, #1482, #4962, #11144, #13246, #8749, #1792, #6506, #5274, #9985, #13401, #8587, #11221, #8670, #10993, #2805, #2951, #9677, #6197, #12064, #12299, #331, #14490, #8824, #13320, #2725, #14565, #1711, #409, #7428, #14408, #5198, #7510, #12228, #13551, #10913, #13481, #8511, #7659, #1639, #5118, #6354, #12147, #1564, #9833, #563, #14723, #9912, #3807, #6279, #7351, #3964, #11067, #484, #12375, #4123, #5045, #9761, #3888, #14646, #4043, #2881, #7582, #6425, #640, #10061, #5344, #14797, #4192, #8898, #502, #270, #12315, #12005, #3829, #6371, #1431, #430, #10008, #8691, #9778, #1658, #6220, #1733, #14742, #1587, #5066, #7369, #14510, #13264, #12248, #11083, #11015, #13425, #10851, #10935, #12169, #4141, #5220, #7453, #9930, #3910, #353, #8530, #5296, #2669, #14664, #4069, #8770, #8606, #6298, #13502, #13341, #7292, #14584, #5140, #13185, #9851, #2899, #7600, #6445, #3986, #2830, #2749, #7530, #11162, #12084, #582, #1508, #2591, #6137, #4984, #9699, #14432, #10235, #15038, #2115, #5512, #7681, #1959, #15117, #811, #6526, #3047, #952, #13721, #11389, #4361, #14815 ),
 ( #4212, #7759, #12702, #1891, #12473, #3120, #5586, #14891, #6601, #8841, #9070, #14968, #6674, #6821, #8917, #2040, #12394, #11537, #12548, #4288, #13791, #11310, #731, #8993, #4432, #3268, #3189, #13568, #5436, #10156, #11240, #5364, #2969, #9143, #1814, #12626, #5657, #10378, #13868, #7980, #7901, #7834, #659, #6751, #11464, #884, #10080, #13646, #10300, #11611, #11828, #15193, #14018, #8350, #12854, #8125, #14094, #1252, #10531, #2267, #4508, #4735, #7040, #12933, #13076, #10454, #13007, #8052, #7186, #8203, #15264, #1177, #6972, #11687, #4655, #97, #14245, #9446, #10757, #1106, #13947, #5811, #9364, #3497, #11909, #9524, #1030, #4586, #9216, #14174, #2344, #2412, #6037, #3577, #8279, #9293, #4810, #7108, #5958, #5736, #19, #11757, #3344, #3415, #5878, #6891, #10598, #10680, #3647, #2492, #1334, #12780, #2187, #483, #3725, #9676, #8510, #2648, #4042, #6115, #12063, #7581, #2880, #3887, #4881, #6424, #408, #7350, #5117, #2804, #8669, #5197, #13163, #12298, #5043, #9832, #9911, #13400, #14645, #1481, #2724, #9593, #2572, #6196, #11066, #14489, #14564, #8747, #10828, #9760, #6353, #1563, #8430, #10912, #7508, #7427, #330, #11987, #246, #174, #3963, #8586, #12227, #1710, #1638, #13480, #4961, #14321, #7273, #1410, #14407, #10992, #13245, #3805, #13319, #12146, #6277, #9983, #562, #5273, #4122, #14722, #11143, #288, #11177, #14451, #5082, #3924, #13357, #14759, #1525, #7468, #2989, #13585, #14602, #5001, #1833, #11097, #2765, #519, #13516, #4084, #601, #8544, #7697, #446, #5236, #5311, #8787, #10023, #12184, #13441, #9718, #13281, #1603, #6460, #9867, #9944, #4157, #6236, #5155, #1750, #12264, #3845, #6316, #2916, #2847, #11030, #9795, #2683, #7382, #10868, #8859, #12102, #14681, #12411, #10952, #373, #14525, #4004, #8620 ),
 ( #1673, #7616, #8706, #7545, #6386, #12331, #13737, #11555, #11255, #4379, #9012, #6772, #827, #9166, #8075, #5459, #12725, #6839, #2136, #14910, #9088, #971, #15058, #748, #5678, #13809, #3364, #10176, #904, #14983, #13969, #10405, #12799, #7928, #8003, #6621, #5605, #3209, #6542, #15137, #676, #12646, #4532, #11329, #5532, #5382, #2060, #11488, #4452, #10319, #10251, #13893, #8936, #9242, #10096, #12490, #3290, #14832, #4231, #13664, #3065, #3136, #7776, #4307, #1907, #7850, #12567, #1979, #6695, #11409, #2287, #1274, #5978, #42, #2432, #15214, #10550, #1195, #14345, #10701, #11777, #4831, #9386, #4675, #12876, #9615, #6992, #9543, #117, #14269, #12955, #5897, #3668, #15283, #11633, #3598, #10619, #8452, #9468, #8370, #13100, #2515, #14194, #8299, #14116, #11848, #3517, #8146, #4752, #11708, #3748, #13027, #2205, #6912, #7210, #7127, #11930, #10776, #1354, #1051, #6058, #5758, #193, #4606, #1126, #10480, #7059, #4903, #9315, #5828, #14038, #3435, #8225, #2362, #1329, #4604, #1477, #11905, #6910, #6192, #5756, #1049, #7182, #9672, #3433, #10478, #12723, #13159, #170, #6033, #10908, #3362, #6111, #969, #326, #10753, #8144, #9589, #15212, #9312, #12874, #8506, #7346, #2568, #8073, #10824, #11553, #4877, #9757, #8426, #14036, #1406, #2285, #5039, #14485, #14317, #3721, #11631, #7269, #12797, #11983, #242, #4957, #14403, #10402, #3801, #13241, #3883, #2644, #12059, #2134, #6837, #5676, #2203, #15135, #4530, #9240, #13967, #11216, #4038, #12295, #636, #6349, #2720, #9979, #1706, #14870, #558, #1788, #4188, #7655, #5269, #14718, #5193, #2947, #9907, #14560, #6420, #3958, #10128, #4118, #8582, #13315, #6502, #8820, #14793, #1870, #13547, #7423, #11139, #12141, #12371, #6273, #2800, #709, #13476, #5340, #10057, #8665, #12452, #1559 ),
 ( #1634, #8894, #13626, #479, #3026, #10988, #7733, #11062, #6575, #2877, #11287, #404, #7504, #5413, #5113, #9828, #14641, #13396, #12223, #8743, #7577, #3396, #2091, #1083, #13769, #13925, #12676, #11666, #8105, #10510, #5636, #5714, #4340, #3244, #4266, #6801, #4486, #2169, #10350, #7956, #6871, #6651, #12830, #3098, #9273, #8968, #11517, #6727, #9196, #13842, #11587, #5790, #3164, #10433, #4564, #15171, #12600, #932, #13997, #12758, #7876, #2243, #15092, #13698, #2017, #3323, #8033, #7810, #6948, #12522, #1004, #1938, #9048, #11360, #787, #5492, #10211, #14945, #11440, #862, #5564, #10279, #15015, #4406, #9115, #8406, #14069, #2465, #12038, #10734, #11807, #3696, #8257, #3783, #1459, #3624, #7086, #9424, #1223, #14887, #14297, #13138, #13053, #148, #12908, #12984, #14223, #6167, #2548, #9500, #7249, #5934, #2389, #10577, #7326, #4712, #11964, #1387, #6088, #10658, #8327, #10805, #73, #9346, #1307, #7163, #15244, #11884, #220, #4935, #9652, #6010, #4858, #4785, #9569, #14383, #5858, #8489, #14150, #4636, #13220, #3472, #8184, #2623, #2322, #7021, #11735, #1155, #3550, #4020, #1851, #2861, #8562, #5097, #3009, #462, #13457, #6401, #1540, #14774, #306, #9961, #9738, #5020, #14467, #9810, #11046, #2700, #3939, #11196, #14698, #2782, #1619, #619, #3863, #5324, #13297, #14542, #8640, #13377, #4171, #6254, #7485, #7714, #13606, #14623, #7399, #10889, #11116, #12203, #538, #13532, #4101, #10037, #12123, #12430, #5173, #5251, #8875, #8802, #10970, #6331, #7561, #388, #9884, #8723, #6479, #12280, #2931, #1690, #7634, #12350, #1769, #5396, #6556, #691, #14850, #10111, #11268, #5000, #3764, #2605, #6071, #12263, #14364, #9866, #2915, #7615, #6385, #11096, #14524, #9717, #12330, #9794, #12101, #3923, #4082, #10788, #8619, #13280, #9943 ),
 ( #13356, #8543, #6315, #371, #8705, #204, #14449, #1672, #518, #5235, #3844, #2764, #14680, #14601, #287, #8786, #7467, #4917, #2682, #445, #12183, #13515, #9631, #8468, #1601, #7544, #6149, #5081, #13200, #11029, #5154, #4003, #13440, #2845, #7307, #12022, #1443, #10867, #7381, #1524, #6235, #10951, #13891, #12564, #13662, #5530, #10094, #5603, #3288, #5457, #8934, #8002, #1977, #6693, #1831, #2058, #10249, #825, #13583, #11407, #14830, #6459, #8857, #10174, #4155, #3134, #4229, #6619, #10317, #7774, #6770, #11176, #11485, #5309, #11253, #3063, #12488, #15056, #7695, #1905, #9164, #4450, #14908, #600, #1749, #14981, #11327, #4377, #9086, #13807, #902, #14757, #10022, #746, #3207, #2987, #7926, #12409, #4305, #9010, #6540, #674, #13735, #12644, #7848, #5380, #2181, #11457, #7751, #8911, #5729, #10295, #4205, #13639, #12695, #5580, #10371, #12774, #877, #3041, #12619, #10448, #15032, #1886, #13715, #11602, #9063, #6745, #4426, #10150, #8046, #12467, #3260, #6595, #11303, #724, #3114, #4355, #5430, #12541, #4502, #7973, #11383, #9210, #14884, #2033, #6667, #9136, #13785, #6814, #4281, #7827, #15109, #13940, #3338, #1952, #13862, #6885, #2109, #805, #1024, #11532, #8986, #5506, #946, #5650, #10228, #14962, #3183, #7895, #1325, #15258, #14166, #6106, #8272, #90, #13068, #1242, #3569, #7034, #3714, #13000, #9358, #8421, #8196, #3489, #9439, #11901, #5871, #12927, #15186, #4801, #2404, #7102, #13154, #5803, #8342, #3409, #2564, #11821, #10590, #5950, #2337, #11748, #9, #10748, #9585, #9517, #4580, #1170, #9287, #4728, #10673, #14238, #7265, #4873, #11681, #10525, #14012, #3640, #2483, #7178, #1399, #6027, #166, #4649, #14311, #11980, #8119, #1098, #12847, #2260, #6966, #14085, #14557, #13237, #12220, #8578, #401, #4114, #1555 ) ),
 .UNSPECIFIED., .T., .F., .T. ) 
 B_SPLINE_SURFACE_WITH_KNOTS ( ( 4, 3, 4 ),
 ( 3, 2, 2, 2, 2, 2, 2, 2, 2, 2, 2, 2, 2, 2, 2, 2, 2, 2, 2, 2, 2, 2, 2, 2, 2, 2, 2, 2, 2, 2, 2, 2, 2, 2, 2, 2, 2, 2, 2, 2, 2, 2, 2, 2, 2, 2, 2, 2, 2, 2, 2, 2, 2, 2, 2, 2, 2, 2, 2, 2, 2, 2, 2, 2, 2, 2, 2, 2, 2, 2, 2, 2, 2, 2, 2, 2, 2, 2, 2, 2, 2, 2, 2, 2, 2, 2, 2, 2, 2, 2, 2, 2, 2, 2, 2, 2, 2, 2, 2, 2, 2, 2, 2, 2, 2, 2, 2, 2, 2, 2, 2, 2, 2, 2, 2, 2, 2, 2, 2, 2, 3 ),
 ( 0.000000000000000000, 0.5000000000000000000, 1.000000000000000000 ),
 ( 0.000000000000000000, 0.008333333333333333218, 0.01666666666666666644, 0.02500000000000000139, 0.03333333333333333287, 0.04166666666666666435, 0.05000000000000000278, 0.05833333333333333426, 0.06666666666666666574, 0.07499999999999999722, 0.08333333333333332871, 0.09166666666666666019, 0.1000000000000000056, 0.1083333333333333370, 0.1166666666666666685, 0.1250000000000000000, 0.1333333333333333315, 0.1416666666666666630, 0.1499999999999999944, 0.1583333333333333259, 0.1666666666666666574, 0.1749999999999999889, 0.1833333333333333204, 0.1916666666666666519, 0.2000000000000000111, 0.2083333333333333426, 0.2166666666666666741, 0.2250000000000000056, 0.2333333333333333370, 0.2416666666666666685, 0.2500000000000000000, 0.2583333333333333037, 0.2666666666666666630, 0.2750000000000000222, 0.2833333333333333259, 0.2916666666666666852, 0.2999999999999999889, 0.3083333333333333481, 0.3166666666666666519, 0.3250000000000000111, 0.3333333333333333148, 0.3416666666666666741, 0.3499999999999999778, 0.3583333333333333370, 0.3666666666666666408, 0.3750000000000000000, 0.3833333333333333037, 0.3916666666666666630, 0.4000000000000000222, 0.4083333333333333259, 0.4166666666666666852, 0.4249999999999999889, 0.4333333333333333481, 0.4416666666666666519, 0.4500000000000000111, 0.4583333333333333148, 0.4666666666666666741, 0.4749999999999999778, 0.4833333333333333370, 0.4916666666666666408, 0.5000000000000000000, 0.5083333333333333037, 0.5166666666666666075, 0.5250000000000000222, 0.5333333333333333259, 0.5416666666666666297, 0.5500000000000000444, 0.5583333333333333481, 0.5666666666666666519, 0.5749999999999999556, 0.5833333333333333703, 0.5916666666666666741, 0.5999999999999999778, 0.6083333333333332815, 0.6166666666666666963, 0.6250000000000000000, 0.6333333333333333037, 0.6416666666666666075, 0.6500000000000000222, 0.6583333333333333259, 0.6666666666666666297, 0.6750000000000000444, 0.6833333333333333481, 0.6916666666666666519, 0.6999999999999999556, 0.7083333333333333703, 0.7166666666666666741, 0.7249999999999999778, 0.7333333333333332815, 0.7416666666666666963, 0.7500000000000000000, 0.7583333333333333037, 0.7666666666666666075, 0.7750000000000000222, 0.7833333333333333259, 0.7916666666666666297, 0.8000000000000000444, 0.8083333333333333481, 0.8166666666666666519, 0.8249999999999999556, 0.8333333333333333703, 0.8416666666666666741, 0.8499999999999999778, 0.8583333333333332815, 0.8666666666666666963, 0.8750000000000000000, 0.8833333333333333037, 0.8916666666666666075, 0.9000000000000000222, 0.9083333333333333259, 0.9166666666666666297, 0.9249999999999999334, 0.9333333333333333481, 0.9416666666666666519, 0.9499999999999999556, 0.9583333333333333703, 0.9666666666666666741, 0.9749999999999999778, 0.9833333333333332815, 0.9916666666666666963, 1.000000000000000000 ),
 .UNSPECIFIED. ) 
 GEOMETRIC_REPRESENTATION_ITEM ( )  RATIONAL_B_SPLINE_SURFACE ( (
 ( 1.000000000000000000, 0.9238795325112867385, 1.000000000000000000, 0.9238795325112867385, 1.000000000000000000, 0.9238795325112867385, 1.000000000000000000, 0.9238795325112867385, 1.000000000000000000, 0.9238795325112867385, 1.000000000000000000, 0.9238795325112867385, 1.000000000000000000, 0.9238795325112867385, 1.000000000000000000, 0.9238795325112867385, 1.000000000000000000, 0.9238795325112867385, 1.000000000000000000, 0.9238795325112867385, 1.000000000000000000, 0.9238795325112867385, 1.000000000000000000, 0.9238795325112867385, 1.000000000000000000, 0.9238795325112867385, 1.000000000000000000, 0.9238795325112867385, 1.000000000000000000, 0.9238795325112867385, 1.000000000000000000, 0.9238795325112867385, 1.000000000000000000, 0.9238795325112867385, 1.000000000000000000, 0.9238795325112867385, 1.000000000000000000, 0.9238795325112867385, 1.000000000000000000, 0.9238795325112867385, 1.000000000000000000, 0.9238795325112867385, 1.000000000000000000, 0.9238795325112867385, 1.000000000000000000, 0.9238795325112867385, 1.000000000000000000, 0.9238795325112867385, 1.000000000000000000, 0.9238795325112867385, 1.000000000000000000, 0.9238795325112867385, 1.000000000000000000, 0.9238795325112867385, 1.000000000000000000, 0.9238795325112867385, 1.000000000000000000, 0.9238795325112867385, 1.000000000000000000, 0.9238795325112867385, 1.000000000000000000, 0.9238795325112867385, 1.000000000000000000, 0.9238795325112867385, 1.000000000000000000, 0.9238795325112867385, 1.000000000000000000, 0.9238795325112867385, 1.000000000000000000, 0.9238795325112867385, 1.000000000000000000, 0.9238795325112867385, 1.000000000000000000, 0.9238795325112867385, 1.000000000000000000, 0.9238795325112867385, 1.000000000000000000, 0.9238795325112867385, 1.000000000000000000, 0.9238795325112867385, 1.000000000000000000, 0.9238795325112867385, 1.000000000000000000, 0.9238795325112867385, 1.000000000000000000, 0.9238795325112867385, 1.000000000000000000, 0.9238795325112867385, 1.000000000000000000, 0.9238795325112867385, 1.000000000000000000, 0.9238795325112867385, 1.000000000000000000, 0.9238795325112867385, 1.000000000000000000, 0.9238795325112867385, 1.000000000000000000, 0.9238795325112867385, 1.000000000000000000, 0.9238795325112867385, 1.000000000000000000, 0.9238795325112867385, 1.000000000000000000, 0.9238795325112867385, 1.000000000000000000, 0.9238795325112867385, 1.000000000000000000, 0.9238795325112867385, 1.000000000000000000, 0.9238795325112867385, 1.000000000000000000, 0.9238795325112867385, 1.000000000000000000, 0.9238795325112867385, 1.000000000000000000, 0.9238795325112867385, 1.000000000000000000, 0.9238795325112867385, 1.000000000000000000, 0.9238795325112867385, 1.000000000000000000, 0.9238795325112867385, 1.000000000000000000, 0.9238795325112867385, 1.000000000000000000, 0.9238795325112867385, 1.000000000000000000, 0.9238795325112867385, 1.000000000000000000, 0.9238795325112867385, 1.000000000000000000, 0.9238795325112867385, 1.000000000000000000, 0.9238795325112867385, 1.000000000000000000, 0.9238795325112867385, 1.000000000000000000, 0.9238795325112867385, 1.000000000000000000, 0.9238795325112867385, 1.000000000000000000, 0.9238795325112867385, 1.000000000000000000, 0.9238795325112867385, 1.000000000000000000, 0.9238795325112867385, 1.000000000000000000, 0.9238795325112867385, 1.000000000000000000, 0.9238795325112867385, 1.000000000000000000, 0.9238795325112867385, 1.000000000000000000, 0.9238795325112867385, 1.000000000000000000, 0.9238795325112867385, 1.000000000000000000, 0.9238795325112867385, 1.000000000000000000, 0.9238795325112867385, 1.000000000000000000, 0.9238795325112867385, 1.000000000000000000, 0.9238795325112867385, 1.000000000000000000, 0.9238795325112867385, 1.000000000000000000, 0.9238795325112867385, 1.000000000000000000, 0.9238795325112867385, 1.000000000000000000, 0.9238795325112867385, 1.000000000000000000, 0.9238795325112867385, 1.000000000000000000, 0.9238795325112867385, 1.000000000000000000, 0.9238795325112867385, 1.000000000000000000, 0.9238795325112867385, 1.000000000000000000, 0.9238795325112867385, 1.000000000000000000, 0.9238795325112867385, 1.000000000000000000, 0.9238795325112867385, 1.000000000000000000, 0.9238795325112867385, 1.000000000000000000, 0.9238795325112867385, 1.000000000000000000, 0.9238795325112867385, 1.000000000000000000, 0.9238795325112867385, 1.000000000000000000, 0.9238795325112867385, 1.000000000000000000, 0.9238795325112867385, 1.000000000000000000, 0.9238795325112867385, 1.000000000000000000, 0.9238795325112867385, 1.000000000000000000, 0.9238795325112867385, 1.000000000000000000, 0.9238795325112867385, 1.000000000000000000, 0.9238795325112867385, 1.000000000000000000, 0.9238795325112867385, 1.000000000000000000, 0.9238795325112867385, 1.000000000000000000, 0.9238795325112867385, 1.000000000000000000, 0.9238795325112867385, 1.000000000000000000, 0.9238795325112867385, 1.000000000000000000, 0.9238795325112867385, 1.000000000000000000, 0.9238795325112867385, 1.000000000000000000, 0.9238795325112867385, 1.000000000000000000, 0.9238795325112867385, 1.000000000000000000, 0.9238795325112867385, 1.000000000000000000, 0.9238795325112867385, 1.000000000000000000, 0.9238795325112867385, 1.000000000000000000, 0.9238795325112867385, 1.000000000000000000, 0.9238795325112867385, 1.000000000000000000, 0.9238795325112867385, 1.000000000000000000, 0.9238795325112867385, 1.000000000000000000),
 ( 0.3333333333333333703, 0.3079598441704289313, 0.3333333333333333703, 0.3079598441704289313, 0.3333333333333333703, 0.3079598441704289313, 0.3333333333333333703, 0.3079598441704289313, 0.3333333333333333703, 0.3079598441704289313, 0.3333333333333333703, 0.3079598441704289313, 0.3333333333333333703, 0.3079598441704289313, 0.3333333333333333703, 0.3079598441704289313, 0.3333333333333333703, 0.3079598441704289313, 0.3333333333333333703, 0.3079598441704289313, 0.3333333333333333703, 0.3079598441704289313, 0.3333333333333333703, 0.3079598441704289313, 0.3333333333333333703, 0.3079598441704289313, 0.3333333333333333703, 0.3079598441704289313, 0.3333333333333333703, 0.3079598441704289313, 0.3333333333333333703, 0.3079598441704289313, 0.3333333333333333703, 0.3079598441704289313, 0.3333333333333333703, 0.3079598441704289313, 0.3333333333333333703, 0.3079598441704289313, 0.3333333333333333703, 0.3079598441704289313, 0.3333333333333333703, 0.3079598441704289313, 0.3333333333333333703, 0.3079598441704289313, 0.3333333333333333703, 0.3079598441704289313, 0.3333333333333333703, 0.3079598441704289313, 0.3333333333333333703, 0.3079598441704289313, 0.3333333333333333703, 0.3079598441704289313, 0.3333333333333333703, 0.3079598441704289313, 0.3333333333333333703, 0.3079598441704289313, 0.3333333333333333703, 0.3079598441704289313, 0.3333333333333333703, 0.3079598441704289313, 0.3333333333333333703, 0.3079598441704289313, 0.3333333333333333703, 0.3079598441704289313, 0.3333333333333333703, 0.3079598441704289313, 0.3333333333333333703, 0.3079598441704289313, 0.3333333333333333703, 0.3079598441704289313, 0.3333333333333333703, 0.3079598441704289313, 0.3333333333333333703, 0.3079598441704289313, 0.3333333333333333703, 0.3079598441704289313, 0.3333333333333333703, 0.3079598441704289313, 0.3333333333333333703, 0.3079598441704289313, 0.3333333333333333703, 0.3079598441704289313, 0.3333333333333333703, 0.3079598441704289313, 0.3333333333333333703, 0.3079598441704289313, 0.3333333333333333703, 0.3079598441704289313, 0.3333333333333333703, 0.3079598441704289313, 0.3333333333333333703, 0.3079598441704289313, 0.3333333333333333703, 0.3079598441704289313, 0.3333333333333333703, 0.3079598441704289313, 0.3333333333333333703, 0.3079598441704289313, 0.3333333333333333703, 0.3079598441704289313, 0.3333333333333333703, 0.3079598441704289313, 0.3333333333333333703, 0.3079598441704289313, 0.3333333333333333703, 0.3079598441704289313, 0.3333333333333333703, 0.3079598441704289313, 0.3333333333333333703, 0.3079598441704289313, 0.3333333333333333703, 0.3079598441704289313, 0.3333333333333333703, 0.3079598441704289313, 0.3333333333333333703, 0.3079598441704289313, 0.3333333333333333703, 0.3079598441704289313, 0.3333333333333333703, 0.3079598441704289313, 0.3333333333333333703, 0.3079598441704289313, 0.3333333333333333703, 0.3079598441704289313, 0.3333333333333333703, 0.3079598441704289313, 0.3333333333333333703, 0.3079598441704289313, 0.3333333333333333703, 0.3079598441704289313, 0.3333333333333333703, 0.3079598441704289313, 0.3333333333333333703, 0.3079598441704289313, 0.3333333333333333703, 0.3079598441704289313, 0.3333333333333333703, 0.3079598441704289313, 0.3333333333333333703, 0.3079598441704289313, 0.3333333333333333703, 0.3079598441704289313, 0.3333333333333333703, 0.3079598441704289313, 0.3333333333333333703, 0.3079598441704289313, 0.3333333333333333703, 0.3079598441704289313, 0.3333333333333333703, 0.3079598441704289313, 0.3333333333333333703, 0.3079598441704289313, 0.3333333333333333703, 0.3079598441704289313, 0.3333333333333333703, 0.3079598441704289313, 0.3333333333333333703, 0.3079598441704289313, 0.3333333333333333703, 0.3079598441704289313, 0.3333333333333333703, 0.3079598441704289313, 0.3333333333333333703, 0.3079598441704289313, 0.3333333333333333703, 0.3079598441704289313, 0.3333333333333333703, 0.3079598441704289313, 0.3333333333333333703, 0.3079598441704289313, 0.3333333333333333703, 0.3079598441704289313, 0.3333333333333333703, 0.3079598441704289313, 0.3333333333333333703, 0.3079598441704289313, 0.3333333333333333703, 0.3079598441704289313, 0.3333333333333333703, 0.3079598441704289313, 0.3333333333333333703, 0.3079598441704289313, 0.3333333333333333703, 0.3079598441704289313, 0.3333333333333333703, 0.3079598441704289313, 0.3333333333333333703, 0.3079598441704289313, 0.3333333333333333703, 0.3079598441704289313, 0.3333333333333333703, 0.3079598441704289313, 0.3333333333333333703, 0.3079598441704289313, 0.3333333333333333703, 0.3079598441704289313, 0.3333333333333333703, 0.3079598441704289313, 0.3333333333333333703, 0.3079598441704289313, 0.3333333333333333703, 0.3079598441704289313, 0.3333333333333333703, 0.3079598441704289313, 0.3333333333333333703, 0.3079598441704289313, 0.3333333333333333703, 0.3079598441704289313, 0.3333333333333333703, 0.3079598441704289313, 0.3333333333333333703, 0.3079598441704289313, 0.3333333333333333703, 0.3079598441704289313, 0.3333333333333333703, 0.3079598441704289313, 0.3333333333333333703, 0.3079598441704289313, 0.3333333333333333703, 0.3079598441704289313, 0.3333333333333333703, 0.3079598441704289313, 0.3333333333333333703, 0.3079598441704289313, 0.3333333333333333703, 0.3079598441704289313, 0.3333333333333333703, 0.3079598441704289313, 0.3333333333333333703, 0.3079598441704289313, 0.3333333333333333703, 0.3079598441704289313, 0.3333333333333333703, 0.3079598441704289313, 0.3333333333333333703, 0.3079598441704289313, 0.3333333333333333703, 0.3079598441704289313, 0.3333333333333333703, 0.3079598441704289313, 0.3333333333333333703),
 ( 0.3333333333333333703, 0.3079598441704289313, 0.3333333333333333703, 0.3079598441704289313, 0.3333333333333333703, 0.3079598441704289313, 0.3333333333333333703, 0.3079598441704289313, 0.3333333333333333703, 0.3079598441704289313, 0.3333333333333333703, 0.3079598441704289313, 0.3333333333333333703, 0.3079598441704289313, 0.3333333333333333703, 0.3079598441704289313, 0.3333333333333333703, 0.3079598441704289313, 0.3333333333333333703, 0.3079598441704289313, 0.3333333333333333703, 0.3079598441704289313, 0.3333333333333333703, 0.3079598441704289313, 0.3333333333333333703, 0.3079598441704289313, 0.3333333333333333703, 0.3079598441704289313, 0.3333333333333333703, 0.3079598441704289313, 0.3333333333333333703, 0.3079598441704289313, 0.3333333333333333703, 0.3079598441704289313, 0.3333333333333333703, 0.3079598441704289313, 0.3333333333333333703, 0.3079598441704289313, 0.3333333333333333703, 0.3079598441704289313, 0.3333333333333333703, 0.3079598441704289313, 0.3333333333333333703, 0.3079598441704289313, 0.3333333333333333703, 0.3079598441704289313, 0.3333333333333333703, 0.3079598441704289313, 0.3333333333333333703, 0.3079598441704289313, 0.3333333333333333703, 0.3079598441704289313, 0.3333333333333333703, 0.3079598441704289313, 0.3333333333333333703, 0.3079598441704289313, 0.3333333333333333703, 0.3079598441704289313, 0.3333333333333333703, 0.3079598441704289313, 0.3333333333333333703, 0.3079598441704289313, 0.3333333333333333703, 0.3079598441704289313, 0.3333333333333333703, 0.3079598441704289313, 0.3333333333333333703, 0.3079598441704289313, 0.3333333333333333703, 0.3079598441704289313, 0.3333333333333333703, 0.3079598441704289313, 0.3333333333333333703, 0.3079598441704289313, 0.3333333333333333703, 0.3079598441704289313, 0.3333333333333333703, 0.3079598441704289313, 0.3333333333333333703, 0.3079598441704289313, 0.3333333333333333703, 0.3079598441704289313, 0.3333333333333333703, 0.3079598441704289313, 0.3333333333333333703, 0.3079598441704289313, 0.3333333333333333703, 0.3079598441704289313, 0.3333333333333333703, 0.3079598441704289313, 0.3333333333333333703, 0.3079598441704289313, 0.3333333333333333703, 0.3079598441704289313, 0.3333333333333333703, 0.3079598441704289313, 0.3333333333333333703, 0.3079598441704289313, 0.3333333333333333703, 0.3079598441704289313, 0.3333333333333333703, 0.3079598441704289313, 0.3333333333333333703, 0.3079598441704289313, 0.3333333333333333703, 0.3079598441704289313, 0.3333333333333333703, 0.3079598441704289313, 0.3333333333333333703, 0.3079598441704289313, 0.3333333333333333703, 0.3079598441704289313, 0.3333333333333333703, 0.3079598441704289313, 0.3333333333333333703, 0.3079598441704289313, 0.3333333333333333703, 0.3079598441704289313, 0.3333333333333333703, 0.3079598441704289313, 0.3333333333333333703, 0.3079598441704289313, 0.3333333333333333703, 0.3079598441704289313, 0.3333333333333333703, 0.3079598441704289313, 0.3333333333333333703, 0.3079598441704289313, 0.3333333333333333703, 0.3079598441704289313, 0.3333333333333333703, 0.3079598441704289313, 0.3333333333333333703, 0.3079598441704289313, 0.3333333333333333703, 0.3079598441704289313, 0.3333333333333333703, 0.3079598441704289313, 0.3333333333333333703, 0.3079598441704289313, 0.3333333333333333703, 0.3079598441704289313, 0.3333333333333333703, 0.3079598441704289313, 0.3333333333333333703, 0.3079598441704289313, 0.3333333333333333703, 0.3079598441704289313, 0.3333333333333333703, 0.3079598441704289313, 0.3333333333333333703, 0.3079598441704289313, 0.3333333333333333703, 0.3079598441704289313, 0.3333333333333333703, 0.3079598441704289313, 0.3333333333333333703, 0.3079598441704289313, 0.3333333333333333703, 0.3079598441704289313, 0.3333333333333333703, 0.3079598441704289313, 0.3333333333333333703, 0.3079598441704289313, 0.3333333333333333703, 0.3079598441704289313, 0.3333333333333333703, 0.3079598441704289313, 0.3333333333333333703, 0.3079598441704289313, 0.3333333333333333703, 0.3079598441704289313, 0.3333333333333333703, 0.3079598441704289313, 0.3333333333333333703, 0.3079598441704289313, 0.3333333333333333703, 0.3079598441704289313, 0.3333333333333333703, 0.3079598441704289313, 0.3333333333333333703, 0.3079598441704289313, 0.3333333333333333703, 0.3079598441704289313, 0.3333333333333333703, 0.3079598441704289313, 0.3333333333333333703, 0.3079598441704289313, 0.3333333333333333703, 0.3079598441704289313, 0.3333333333333333703, 0.3079598441704289313, 0.3333333333333333703, 0.3079598441704289313, 0.3333333333333333703, 0.3079598441704289313, 0.3333333333333333703, 0.3079598441704289313, 0.3333333333333333703, 0.3079598441704289313, 0.3333333333333333703, 0.3079598441704289313, 0.3333333333333333703, 0.3079598441704289313, 0.3333333333333333703, 0.3079598441704289313, 0.3333333333333333703, 0.3079598441704289313, 0.3333333333333333703, 0.3079598441704289313, 0.3333333333333333703, 0.3079598441704289313, 0.3333333333333333703, 0.3079598441704289313, 0.3333333333333333703, 0.3079598441704289313, 0.3333333333333333703, 0.3079598441704289313, 0.3333333333333333703, 0.3079598441704289313, 0.3333333333333333703, 0.3079598441704289313, 0.3333333333333333703, 0.3079598441704289313, 0.3333333333333333703, 0.3079598441704289313, 0.3333333333333333703, 0.3079598441704289313, 0.3333333333333333703, 0.3079598441704289313, 0.3333333333333333703, 0.3079598441704289313, 0.3333333333333333703, 0.3079598441704289313, 0.3333333333333333703, 0.3079598441704289313, 0.3333333333333333703, 0.3079598441704289313, 0.3333333333333333703, 0.3079598441704289313, 0.3333333333333333703),
 ( 1.000000000000000000, 0.9238795325112867385, 1.000000000000000000, 0.9238795325112867385, 1.000000000000000000, 0.9238795325112867385, 1.000000000000000000, 0.9238795325112867385, 1.000000000000000000, 0.9238795325112867385, 1.000000000000000000, 0.9238795325112867385, 1.000000000000000000, 0.9238795325112867385, 1.000000000000000000, 0.9238795325112867385, 1.000000000000000000, 0.9238795325112867385, 1.000000000000000000, 0.9238795325112867385, 1.000000000000000000, 0.9238795325112867385, 1.000000000000000000, 0.9238795325112867385, 1.000000000000000000, 0.9238795325112867385, 1.000000000000000000, 0.9238795325112867385, 1.000000000000000000, 0.9238795325112867385, 1.000000000000000000, 0.9238795325112867385, 1.000000000000000000, 0.9238795325112867385, 1.000000000000000000, 0.9238795325112867385, 1.000000000000000000, 0.9238795325112867385, 1.000000000000000000, 0.9238795325112867385, 1.000000000000000000, 0.9238795325112867385, 1.000000000000000000, 0.9238795325112867385, 1.000000000000000000, 0.9238795325112867385, 1.000000000000000000, 0.9238795325112867385, 1.000000000000000000, 0.9238795325112867385, 1.000000000000000000, 0.9238795325112867385, 1.000000000000000000, 0.9238795325112867385, 1.000000000000000000, 0.9238795325112867385, 1.000000000000000000, 0.9238795325112867385, 1.000000000000000000, 0.9238795325112867385, 1.000000000000000000, 0.9238795325112867385, 1.000000000000000000, 0.9238795325112867385, 1.000000000000000000, 0.9238795325112867385, 1.000000000000000000, 0.9238795325112867385, 1.000000000000000000, 0.9238795325112867385, 1.000000000000000000, 0.9238795325112867385, 1.000000000000000000, 0.9238795325112867385, 1.000000000000000000, 0.9238795325112867385, 1.000000000000000000, 0.9238795325112867385, 1.000000000000000000, 0.9238795325112867385, 1.000000000000000000, 0.9238795325112867385, 1.000000000000000000, 0.9238795325112867385, 1.000000000000000000, 0.9238795325112867385, 1.000000000000000000, 0.9238795325112867385, 1.000000000000000000, 0.9238795325112867385, 1.000000000000000000, 0.9238795325112867385, 1.000000000000000000, 0.9238795325112867385, 1.000000000000000000, 0.9238795325112867385, 1.000000000000000000, 0.9238795325112867385, 1.000000000000000000, 0.9238795325112867385, 1.000000000000000000, 0.9238795325112867385, 1.000000000000000000, 0.9238795325112867385, 1.000000000000000000, 0.9238795325112867385, 1.000000000000000000, 0.9238795325112867385, 1.000000000000000000, 0.9238795325112867385, 1.000000000000000000, 0.9238795325112867385, 1.000000000000000000, 0.9238795325112867385, 1.000000000000000000, 0.9238795325112867385, 1.000000000000000000, 0.9238795325112867385, 1.000000000000000000, 0.9238795325112867385, 1.000000000000000000, 0.9238795325112867385, 1.000000000000000000, 0.9238795325112867385, 1.000000000000000000, 0.9238795325112867385, 1.000000000000000000, 0.9238795325112867385, 1.000000000000000000, 0.9238795325112867385, 1.000000000000000000, 0.9238795325112867385, 1.000000000000000000, 0.9238795325112867385, 1.000000000000000000, 0.9238795325112867385, 1.000000000000000000, 0.9238795325112867385, 1.000000000000000000, 0.9238795325112867385, 1.000000000000000000, 0.9238795325112867385, 1.000000000000000000, 0.9238795325112867385, 1.000000000000000000, 0.9238795325112867385, 1.000000000000000000, 0.9238795325112867385, 1.000000000000000000, 0.9238795325112867385, 1.000000000000000000, 0.9238795325112867385, 1.000000000000000000, 0.9238795325112867385, 1.000000000000000000, 0.9238795325112867385, 1.000000000000000000, 0.9238795325112867385, 1.000000000000000000, 0.9238795325112867385, 1.000000000000000000, 0.9238795325112867385, 1.000000000000000000, 0.9238795325112867385, 1.000000000000000000, 0.9238795325112867385, 1.000000000000000000, 0.9238795325112867385, 1.000000000000000000, 0.9238795325112867385, 1.000000000000000000, 0.9238795325112867385, 1.000000000000000000, 0.9238795325112867385, 1.000000000000000000, 0.9238795325112867385, 1.000000000000000000, 0.9238795325112867385, 1.000000000000000000, 0.9238795325112867385, 1.000000000000000000, 0.9238795325112867385, 1.000000000000000000, 0.9238795325112867385, 1.000000000000000000, 0.9238795325112867385, 1.000000000000000000, 0.9238795325112867385, 1.000000000000000000, 0.9238795325112867385, 1.000000000000000000, 0.9238795325112867385, 1.000000000000000000, 0.9238795325112867385, 1.000000000000000000, 0.9238795325112867385, 1.000000000000000000, 0.9238795325112867385, 1.000000000000000000, 0.9238795325112867385, 1.000000000000000000, 0.9238795325112867385, 1.000000000000000000, 0.9238795325112867385, 1.000000000000000000, 0.9238795325112867385, 1.000000000000000000, 0.9238795325112867385, 1.000000000000000000, 0.9238795325112867385, 1.000000000000000000, 0.9238795325112867385, 1.000000000000000000, 0.9238795325112867385, 1.000000000000000000, 0.9238795325112867385, 1.000000000000000000, 0.9238795325112867385, 1.000000000000000000, 0.9238795325112867385, 1.000000000000000000, 0.9238795325112867385, 1.000000000000000000, 0.9238795325112867385, 1.000000000000000000, 0.9238795325112867385, 1.000000000000000000, 0.9238795325112867385, 1.000000000000000000, 0.9238795325112867385, 1.000000000000000000, 0.9238795325112867385, 1.000000000000000000, 0.9238795325112867385, 1.000000000000000000, 0.9238795325112867385, 1.000000000000000000, 0.9238795325112867385, 1.000000000000000000, 0.9238795325112867385, 1.000000000000000000),
 ( 0.3333333333333333703, 0.3079598441704289313, 0.3333333333333333703, 0.3079598441704289313, 0.3333333333333333703, 0.3079598441704289313, 0.3333333333333333703, 0.3079598441704289313, 0.3333333333333333703, 0.3079598441704289313, 0.3333333333333333703, 0.3079598441704289313, 0.3333333333333333703, 0.3079598441704289313, 0.3333333333333333703, 0.3079598441704289313, 0.3333333333333333703, 0.3079598441704289313, 0.3333333333333333703, 0.3079598441704289313, 0.3333333333333333703, 0.3079598441704289313, 0.3333333333333333703, 0.3079598441704289313, 0.3333333333333333703, 0.3079598441704289313, 0.3333333333333333703, 0.3079598441704289313, 0.3333333333333333703, 0.3079598441704289313, 0.3333333333333333703, 0.3079598441704289313, 0.3333333333333333703, 0.3079598441704289313, 0.3333333333333333703, 0.3079598441704289313, 0.3333333333333333703, 0.3079598441704289313, 0.3333333333333333703, 0.3079598441704289313, 0.3333333333333333703, 0.3079598441704289313, 0.3333333333333333703, 0.3079598441704289313, 0.3333333333333333703, 0.3079598441704289313, 0.3333333333333333703, 0.3079598441704289313, 0.3333333333333333703, 0.3079598441704289313, 0.3333333333333333703, 0.3079598441704289313, 0.3333333333333333703, 0.3079598441704289313, 0.3333333333333333703, 0.3079598441704289313, 0.3333333333333333703, 0.3079598441704289313, 0.3333333333333333703, 0.3079598441704289313, 0.3333333333333333703, 0.3079598441704289313, 0.3333333333333333703, 0.3079598441704289313, 0.3333333333333333703, 0.3079598441704289313, 0.3333333333333333703, 0.3079598441704289313, 0.3333333333333333703, 0.3079598441704289313, 0.3333333333333333703, 0.3079598441704289313, 0.3333333333333333703, 0.3079598441704289313, 0.3333333333333333703, 0.3079598441704289313, 0.3333333333333333703, 0.3079598441704289313, 0.3333333333333333703, 0.3079598441704289313, 0.3333333333333333703, 0.3079598441704289313, 0.3333333333333333703, 0.3079598441704289313, 0.3333333333333333703, 0.3079598441704289313, 0.3333333333333333703, 0.3079598441704289313, 0.3333333333333333703, 0.3079598441704289313, 0.3333333333333333703, 0.3079598441704289313, 0.3333333333333333703, 0.3079598441704289313, 0.3333333333333333703, 0.3079598441704289313, 0.3333333333333333703, 0.3079598441704289313, 0.3333333333333333703, 0.3079598441704289313, 0.3333333333333333703, 0.3079598441704289313, 0.3333333333333333703, 0.3079598441704289313, 0.3333333333333333703, 0.3079598441704289313, 0.3333333333333333703, 0.3079598441704289313, 0.3333333333333333703, 0.3079598441704289313, 0.3333333333333333703, 0.3079598441704289313, 0.3333333333333333703, 0.3079598441704289313, 0.3333333333333333703, 0.3079598441704289313, 0.3333333333333333703, 0.3079598441704289313, 0.3333333333333333703, 0.3079598441704289313, 0.3333333333333333703, 0.3079598441704289313, 0.3333333333333333703, 0.3079598441704289313, 0.3333333333333333703, 0.3079598441704289313, 0.3333333333333333703, 0.3079598441704289313, 0.3333333333333333703, 0.3079598441704289313, 0.3333333333333333703, 0.3079598441704289313, 0.3333333333333333703, 0.3079598441704289313, 0.3333333333333333703, 0.3079598441704289313, 0.3333333333333333703, 0.3079598441704289313, 0.3333333333333333703, 0.3079598441704289313, 0.3333333333333333703, 0.3079598441704289313, 0.3333333333333333703, 0.3079598441704289313, 0.3333333333333333703, 0.3079598441704289313, 0.3333333333333333703, 0.3079598441704289313, 0.3333333333333333703, 0.3079598441704289313, 0.3333333333333333703, 0.3079598441704289313, 0.3333333333333333703, 0.3079598441704289313, 0.3333333333333333703, 0.3079598441704289313, 0.3333333333333333703, 0.3079598441704289313, 0.3333333333333333703, 0.3079598441704289313, 0.3333333333333333703, 0.3079598441704289313, 0.3333333333333333703, 0.3079598441704289313, 0.3333333333333333703, 0.3079598441704289313, 0.3333333333333333703, 0.3079598441704289313, 0.3333333333333333703, 0.3079598441704289313, 0.3333333333333333703, 0.3079598441704289313, 0.3333333333333333703, 0.3079598441704289313, 0.3333333333333333703, 0.3079598441704289313, 0.3333333333333333703, 0.3079598441704289313, 0.3333333333333333703, 0.3079598441704289313, 0.3333333333333333703, 0.3079598441704289313, 0.3333333333333333703, 0.3079598441704289313, 0.3333333333333333703, 0.3079598441704289313, 0.3333333333333333703, 0.3079598441704289313, 0.3333333333333333703, 0.3079598441704289313, 0.3333333333333333703, 0.3079598441704289313, 0.3333333333333333703, 0.3079598441704289313, 0.3333333333333333703, 0.3079598441704289313, 0.3333333333333333703, 0.3079598441704289313, 0.3333333333333333703, 0.3079598441704289313, 0.3333333333333333703, 0.3079598441704289313, 0.3333333333333333703, 0.3079598441704289313, 0.3333333333333333703, 0.3079598441704289313, 0.3333333333333333703, 0.3079598441704289313, 0.3333333333333333703, 0.3079598441704289313, 0.3333333333333333703, 0.3079598441704289313, 0.3333333333333333703, 0.3079598441704289313, 0.3333333333333333703, 0.3079598441704289313, 0.3333333333333333703, 0.3079598441704289313, 0.3333333333333333703, 0.3079598441704289313, 0.3333333333333333703, 0.3079598441704289313, 0.3333333333333333703, 0.3079598441704289313, 0.3333333333333333703, 0.3079598441704289313, 0.3333333333333333703, 0.3079598441704289313, 0.3333333333333333703, 0.3079598441704289313, 0.3333333333333333703, 0.3079598441704289313, 0.3333333333333333703, 0.3079598441704289313, 0.3333333333333333703, 0.3079598441704289313, 0.3333333333333333703, 0.3079598441704289313, 0.3333333333333333703, 0.3079598441704289313, 0.3333333333333333703),
 ( 0.3333333333333333703, 0.3079598441704289313, 0.3333333333333333703, 0.3079598441704289313, 0.3333333333333333703, 0.3079598441704289313, 0.3333333333333333703, 0.3079598441704289313, 0.3333333333333333703, 0.3079598441704289313, 0.3333333333333333703, 0.3079598441704289313, 0.3333333333333333703, 0.3079598441704289313, 0.3333333333333333703, 0.3079598441704289313, 0.3333333333333333703, 0.3079598441704289313, 0.3333333333333333703, 0.3079598441704289313, 0.3333333333333333703, 0.3079598441704289313, 0.3333333333333333703, 0.3079598441704289313, 0.3333333333333333703, 0.3079598441704289313, 0.3333333333333333703, 0.3079598441704289313, 0.3333333333333333703, 0.3079598441704289313, 0.3333333333333333703, 0.3079598441704289313, 0.3333333333333333703, 0.3079598441704289313, 0.3333333333333333703, 0.3079598441704289313, 0.3333333333333333703, 0.3079598441704289313, 0.3333333333333333703, 0.3079598441704289313, 0.3333333333333333703, 0.3079598441704289313, 0.3333333333333333703, 0.3079598441704289313, 0.3333333333333333703, 0.3079598441704289313, 0.3333333333333333703, 0.3079598441704289313, 0.3333333333333333703, 0.3079598441704289313, 0.3333333333333333703, 0.3079598441704289313, 0.3333333333333333703, 0.3079598441704289313, 0.3333333333333333703, 0.3079598441704289313, 0.3333333333333333703, 0.3079598441704289313, 0.3333333333333333703, 0.3079598441704289313, 0.3333333333333333703, 0.3079598441704289313, 0.3333333333333333703, 0.3079598441704289313, 0.3333333333333333703, 0.3079598441704289313, 0.3333333333333333703, 0.3079598441704289313, 0.3333333333333333703, 0.3079598441704289313, 0.3333333333333333703, 0.3079598441704289313, 0.3333333333333333703, 0.3079598441704289313, 0.3333333333333333703, 0.3079598441704289313, 0.3333333333333333703, 0.3079598441704289313, 0.3333333333333333703, 0.3079598441704289313, 0.3333333333333333703, 0.3079598441704289313, 0.3333333333333333703, 0.3079598441704289313, 0.3333333333333333703, 0.3079598441704289313, 0.3333333333333333703, 0.3079598441704289313, 0.3333333333333333703, 0.3079598441704289313, 0.3333333333333333703, 0.3079598441704289313, 0.3333333333333333703, 0.3079598441704289313, 0.3333333333333333703, 0.3079598441704289313, 0.3333333333333333703, 0.3079598441704289313, 0.3333333333333333703, 0.3079598441704289313, 0.3333333333333333703, 0.3079598441704289313, 0.3333333333333333703, 0.3079598441704289313, 0.3333333333333333703, 0.3079598441704289313, 0.3333333333333333703, 0.3079598441704289313, 0.3333333333333333703, 0.3079598441704289313, 0.3333333333333333703, 0.3079598441704289313, 0.3333333333333333703, 0.3079598441704289313, 0.3333333333333333703, 0.3079598441704289313, 0.3333333333333333703, 0.3079598441704289313, 0.3333333333333333703, 0.3079598441704289313, 0.3333333333333333703, 0.3079598441704289313, 0.3333333333333333703, 0.3079598441704289313, 0.3333333333333333703, 0.3079598441704289313, 0.3333333333333333703, 0.3079598441704289313, 0.3333333333333333703, 0.3079598441704289313, 0.3333333333333333703, 0.3079598441704289313, 0.3333333333333333703, 0.3079598441704289313, 0.3333333333333333703, 0.3079598441704289313, 0.3333333333333333703, 0.3079598441704289313, 0.3333333333333333703, 0.3079598441704289313, 0.3333333333333333703, 0.3079598441704289313, 0.3333333333333333703, 0.3079598441704289313, 0.3333333333333333703, 0.3079598441704289313, 0.3333333333333333703, 0.3079598441704289313, 0.3333333333333333703, 0.3079598441704289313, 0.3333333333333333703, 0.3079598441704289313, 0.3333333333333333703, 0.3079598441704289313, 0.3333333333333333703, 0.3079598441704289313, 0.3333333333333333703, 0.3079598441704289313, 0.3333333333333333703, 0.3079598441704289313, 0.3333333333333333703, 0.3079598441704289313, 0.3333333333333333703, 0.3079598441704289313, 0.3333333333333333703, 0.3079598441704289313, 0.3333333333333333703, 0.3079598441704289313, 0.3333333333333333703, 0.3079598441704289313, 0.3333333333333333703, 0.3079598441704289313, 0.3333333333333333703, 0.3079598441704289313, 0.3333333333333333703, 0.3079598441704289313, 0.3333333333333333703, 0.3079598441704289313, 0.3333333333333333703, 0.3079598441704289313, 0.3333333333333333703, 0.3079598441704289313, 0.3333333333333333703, 0.3079598441704289313, 0.3333333333333333703, 0.3079598441704289313, 0.3333333333333333703, 0.3079598441704289313, 0.3333333333333333703, 0.3079598441704289313, 0.3333333333333333703, 0.3079598441704289313, 0.3333333333333333703, 0.3079598441704289313, 0.3333333333333333703, 0.3079598441704289313, 0.3333333333333333703, 0.3079598441704289313, 0.3333333333333333703, 0.3079598441704289313, 0.3333333333333333703, 0.3079598441704289313, 0.3333333333333333703, 0.3079598441704289313, 0.3333333333333333703, 0.3079598441704289313, 0.3333333333333333703, 0.3079598441704289313, 0.3333333333333333703, 0.3079598441704289313, 0.3333333333333333703, 0.3079598441704289313, 0.3333333333333333703, 0.3079598441704289313, 0.3333333333333333703, 0.3079598441704289313, 0.3333333333333333703, 0.3079598441704289313, 0.3333333333333333703, 0.3079598441704289313, 0.3333333333333333703, 0.3079598441704289313, 0.3333333333333333703, 0.3079598441704289313, 0.3333333333333333703, 0.3079598441704289313, 0.3333333333333333703, 0.3079598441704289313, 0.3333333333333333703, 0.3079598441704289313, 0.3333333333333333703, 0.3079598441704289313, 0.3333333333333333703, 0.3079598441704289313, 0.3333333333333333703, 0.3079598441704289313, 0.3333333333333333703, 0.3079598441704289313, 0.3333333333333333703, 0.3079598441704289313, 0.3333333333333333703),
 ( 1.000000000000000000, 0.9238795325112867385, 1.000000000000000000, 0.9238795325112867385, 1.000000000000000000, 0.9238795325112867385, 1.000000000000000000, 0.9238795325112867385, 1.000000000000000000, 0.9238795325112867385, 1.000000000000000000, 0.9238795325112867385, 1.000000000000000000, 0.9238795325112867385, 1.000000000000000000, 0.9238795325112867385, 1.000000000000000000, 0.9238795325112867385, 1.000000000000000000, 0.9238795325112867385, 1.000000000000000000, 0.9238795325112867385, 1.000000000000000000, 0.9238795325112867385, 1.000000000000000000, 0.9238795325112867385, 1.000000000000000000, 0.9238795325112867385, 1.000000000000000000, 0.9238795325112867385, 1.000000000000000000, 0.9238795325112867385, 1.000000000000000000, 0.9238795325112867385, 1.000000000000000000, 0.9238795325112867385, 1.000000000000000000, 0.9238795325112867385, 1.000000000000000000, 0.9238795325112867385, 1.000000000000000000, 0.9238795325112867385, 1.000000000000000000, 0.9238795325112867385, 1.000000000000000000, 0.9238795325112867385, 1.000000000000000000, 0.9238795325112867385, 1.000000000000000000, 0.9238795325112867385, 1.000000000000000000, 0.9238795325112867385, 1.000000000000000000, 0.9238795325112867385, 1.000000000000000000, 0.9238795325112867385, 1.000000000000000000, 0.9238795325112867385, 1.000000000000000000, 0.9238795325112867385, 1.000000000000000000, 0.9238795325112867385, 1.000000000000000000, 0.9238795325112867385, 1.000000000000000000, 0.9238795325112867385, 1.000000000000000000, 0.9238795325112867385, 1.000000000000000000, 0.9238795325112867385, 1.000000000000000000, 0.9238795325112867385, 1.000000000000000000, 0.9238795325112867385, 1.000000000000000000, 0.9238795325112867385, 1.000000000000000000, 0.9238795325112867385, 1.000000000000000000, 0.9238795325112867385, 1.000000000000000000, 0.9238795325112867385, 1.000000000000000000, 0.9238795325112867385, 1.000000000000000000, 0.9238795325112867385, 1.000000000000000000, 0.9238795325112867385, 1.000000000000000000, 0.9238795325112867385, 1.000000000000000000, 0.9238795325112867385, 1.000000000000000000, 0.9238795325112867385, 1.000000000000000000, 0.9238795325112867385, 1.000000000000000000, 0.9238795325112867385, 1.000000000000000000, 0.9238795325112867385, 1.000000000000000000, 0.9238795325112867385, 1.000000000000000000, 0.9238795325112867385, 1.000000000000000000, 0.9238795325112867385, 1.000000000000000000, 0.9238795325112867385, 1.000000000000000000, 0.9238795325112867385, 1.000000000000000000, 0.9238795325112867385, 1.000000000000000000, 0.9238795325112867385, 1.000000000000000000, 0.9238795325112867385, 1.000000000000000000, 0.9238795325112867385, 1.000000000000000000, 0.9238795325112867385, 1.000000000000000000, 0.9238795325112867385, 1.000000000000000000, 0.9238795325112867385, 1.000000000000000000, 0.9238795325112867385, 1.000000000000000000, 0.9238795325112867385, 1.000000000000000000, 0.9238795325112867385, 1.000000000000000000, 0.9238795325112867385, 1.000000000000000000, 0.9238795325112867385, 1.000000000000000000, 0.9238795325112867385, 1.000000000000000000, 0.9238795325112867385, 1.000000000000000000, 0.9238795325112867385, 1.000000000000000000, 0.9238795325112867385, 1.000000000000000000, 0.9238795325112867385, 1.000000000000000000, 0.9238795325112867385, 1.000000000000000000, 0.9238795325112867385, 1.000000000000000000, 0.9238795325112867385, 1.000000000000000000, 0.9238795325112867385, 1.000000000000000000, 0.9238795325112867385, 1.000000000000000000, 0.9238795325112867385, 1.000000000000000000, 0.9238795325112867385, 1.000000000000000000, 0.9238795325112867385, 1.000000000000000000, 0.9238795325112867385, 1.000000000000000000, 0.9238795325112867385, 1.000000000000000000, 0.9238795325112867385, 1.000000000000000000, 0.9238795325112867385, 1.000000000000000000, 0.9238795325112867385, 1.000000000000000000, 0.9238795325112867385, 1.000000000000000000, 0.9238795325112867385, 1.000000000000000000, 0.9238795325112867385, 1.000000000000000000, 0.9238795325112867385, 1.000000000000000000, 0.9238795325112867385, 1.000000000000000000, 0.9238795325112867385, 1.000000000000000000, 0.9238795325112867385, 1.000000000000000000, 0.9238795325112867385, 1.000000000000000000, 0.9238795325112867385, 1.000000000000000000, 0.9238795325112867385, 1.000000000000000000, 0.9238795325112867385, 1.000000000000000000, 0.9238795325112867385, 1.000000000000000000, 0.9238795325112867385, 1.000000000000000000, 0.9238795325112867385, 1.000000000000000000, 0.9238795325112867385, 1.000000000000000000, 0.9238795325112867385, 1.000000000000000000, 0.9238795325112867385, 1.000000000000000000, 0.9238795325112867385, 1.000000000000000000, 0.9238795325112867385, 1.000000000000000000, 0.9238795325112867385, 1.000000000000000000, 0.9238795325112867385, 1.000000000000000000, 0.9238795325112867385, 1.000000000000000000, 0.9238795325112867385, 1.000000000000000000, 0.9238795325112867385, 1.000000000000000000, 0.9238795325112867385, 1.000000000000000000, 0.9238795325112867385, 1.000000000000000000, 0.9238795325112867385, 1.000000000000000000, 0.9238795325112867385, 1.000000000000000000, 0.9238795325112867385, 1.000000000000000000, 0.9238795325112867385, 1.000000000000000000, 0.9238795325112867385, 1.000000000000000000, 0.9238795325112867385, 1.000000000000000000, 0.9238795325112867385, 1.000000000000000000, 0.9238795325112867385, 1.000000000000000000, 0.9238795325112867385, 1.000000000000000000) ) ) 
 REPRESENTATION_ITEM ( '' )  SURFACE ( )  );
#15251=CARTESIAN_POINT ( 'NONE',  ( -1.346194077712559167, 12.93750000000000178, -6.749999999999999112 ) ) ;
#15253=CARTESIAN_POINT ( 'NONE',  ( -3.750000000000000000, 0.6875000000000000000, -1.946699141100893149 ) ) ;
#15258=CARTESIAN_POINT ( 'NONE',  ( 3.249999999999998668, 10.68750000000000000, -4.846194077712560500 ) ) ;
#15264=CARTESIAN_POINT ( 'NONE',  ( -2.651650429449553314, 4.375000000000000000, -6.151650429449552426 ) ) ;
#15265=CARTESIAN_POINT ( 'NONE',  ( -3.750000000000000000, 3.812500000000000000, -5.053300858899105741 ) ) ;
#15268=CARTESIAN_POINT ( 'NONE',  ( -2.298097038856278918, 14.37500000000000000, -5.798097038856277585 ) ) ;
#15272=CARTESIAN_POINT ( 'NONE',  ( 0.000000000000000000, 0.000000000000000000, 0.000000000000000000 ) ) ;
#15273=CARTESIAN_POINT ( 'NONE',  ( -3.249999999999999556, 2.312500000000000888, -4.846194077712557835 ) ) ;
#15279=CARTESIAN_POINT ( 'NONE',  ( 0.000000000000000000, 10.00000000000000000, -0.2500000000000002220 ) ) ;
#15283=CARTESIAN_POINT ( 'NONE',  ( 3.750000000000000000, 5.312500000000000000, -1.946699141100892705 ) ) ;
#15284=CARTESIAN_POINT ( 'NONE',  ( -3.980102097228897738E-16, 8.000000000000000000, -6.749999999999999112 ) ) ;
#15287=CARTESIAN_POINT ( 'NONE',  ( -1.346194077712559389, 1.062500000000000222, -0.2500000000000002220 ) ) ;
#15288=CARTESIAN_POINT ( 'NONE',  ( -2.651650429449553314, 9.375000000000000000, -6.151650429449552426 ) ) ;
#15295=ADVANCED_FACE ( 'NONE', ( #3997 ), #13655, .F. ) ;
#15297=ORIENTED_EDGE ( 'NONE', *, *, #7026, .F. ) ;
#15298=CARTESIAN_POINT ( 'NONE',  ( 3.249999999999998224, 5.312500000000000000, -2.153805922287439945 ) ) ;
#15300=CARTESIAN_POINT ( 'NONE',  ( -1.553300858899106629, 12.56250000000000355, 0.2499999999999998335 ) ) ;
#15304=CARTESIAN_POINT ( 'NONE',  ( -1.346194077712558945, 0.5625000000000003331, -0.2500000000000002220 ) ) ;
#15308=CARTESIAN_POINT ( 'NONE',  ( -2.298097038856278473, 14.12500000000000000, -1.201902961143720416 ) ) ;
#15314=CARTESIAN_POINT ( 'NONE',  ( -3.249999999999999556, 2.312500000000000888, -4.846194077712557835 ) ) ;
#15339=COLOUR_RGB('Sky Blue', 0.40784314, 0.44705882, 0.49803922);
#15340=FILL_AREA_STYLE_COLOUR('',#15339);
#15341=FILL_AREA_STYLE('',(#15340));
#15342=SURFACE_STYLE_FILL_AREA(#15341);
#15343=SURFACE_SIDE_STYLE('',(#15342));
#15344=SURFACE_STYLE_USAGE(.BOTH.,#15343);
#15345=PRESENTATION_STYLE_ASSIGNMENT((#15344));
#15367=STYLED_ITEM('',(#15345),#7115);
#15368=MECHANICAL_DESIGN_GEOMETRIC_PRESENTATION_REPRESENTATION('',(#15367),#6710);
ENDSEC;
END-ISO-10303-21;
